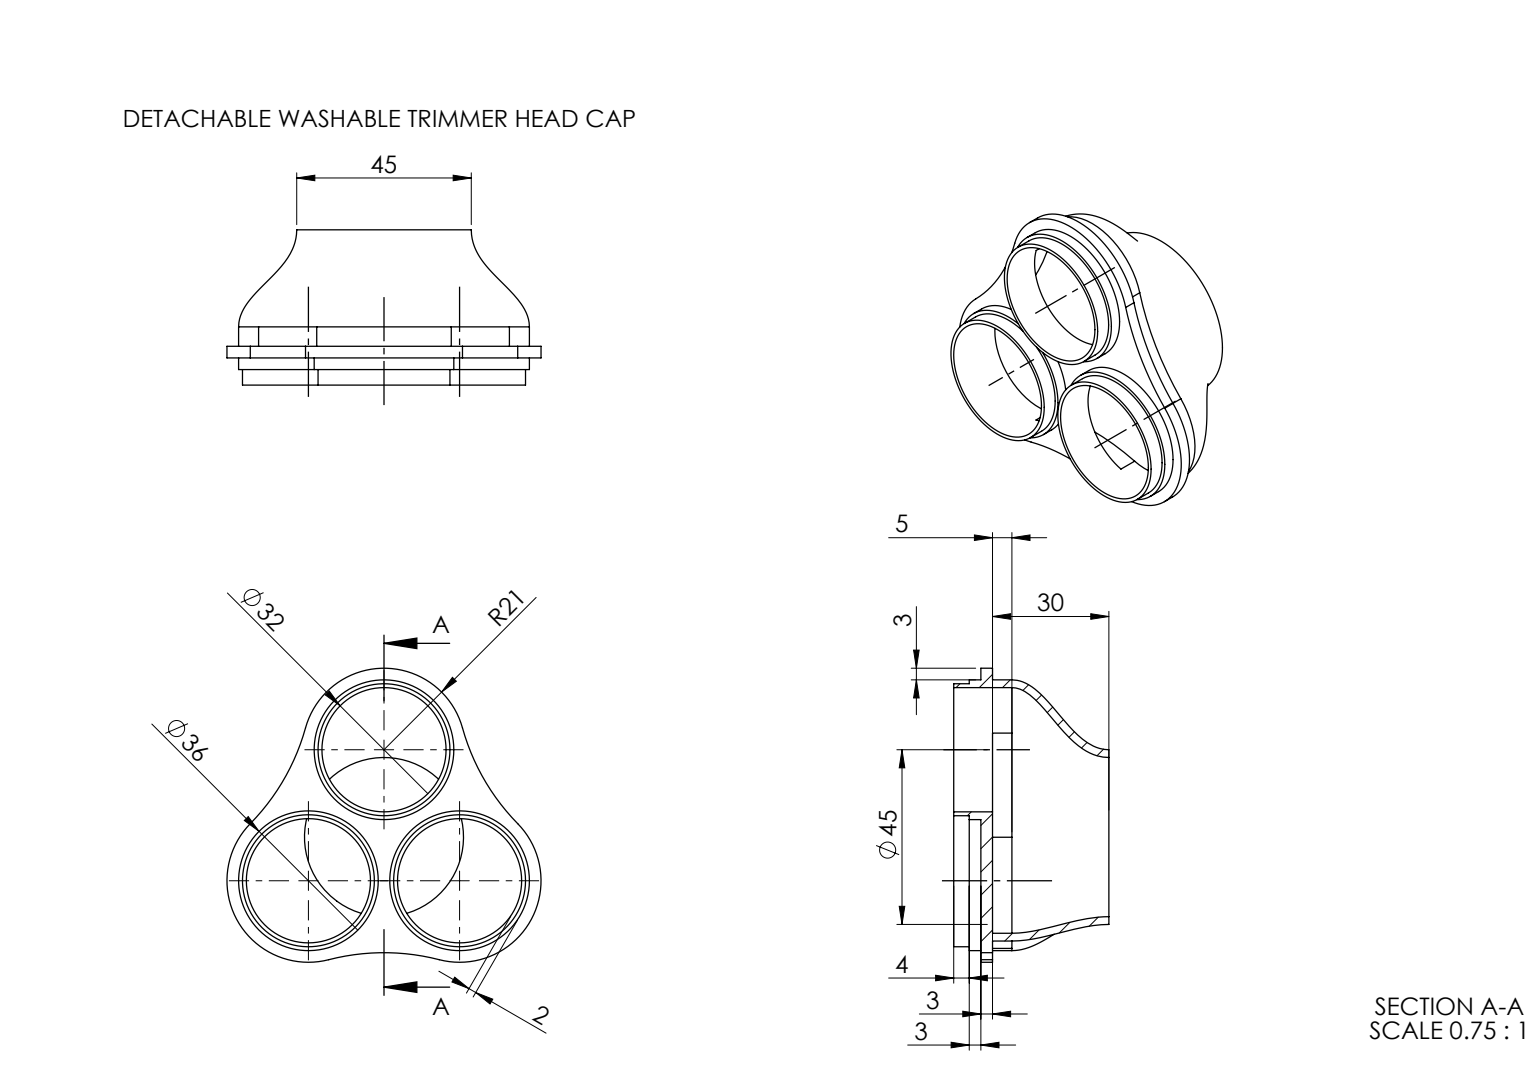
ISO-10303-21;
HEADER;
FILE_DESCRIPTION (('STEP AP214'),
    '1' );
FILE_NAME ('Detachable Washable Trimmer Head Cap.step',
    '2026-10-04T08:29:30',
    ( '' ),
    ( '' ),
    'SwSTEP 2.0',
    'SolidWorks 2026',
    '' );
FILE_SCHEMA (( 'AUTOMOTIVE_DESIGN' ));
ENDSEC;

DATA;
#3=CARTESIAN_POINT ( 'NONE',  ( -6.039637753342756987, 20.17599680590523192, -26.42895019650636712 ) ) ;
#8=CARTESIAN_POINT ( 'NONE',  ( 30.17671132303273041, 0.02011987000799879410, -8.767782600480947153 ) ) ;
#12=CARTESIAN_POINT ( 'NONE',  ( -29.54807517884461632, 0.1037351573273601335, -10.18168607448700591 ) ) ;
#15=CARTESIAN_POINT ( 'NONE',  ( 34.91117196809893386, -7.323106101878850360, -6.322142741489443551 ) ) ;
#28=CARTESIAN_POINT ( 'NONE',  ( 8.056271088701681293, 31.17318759581355536, -12.99397879114828491 ) ) ;
#30=CARTESIAN_POINT ( 'NONE',  ( 10.89305648074092225, -17.83927469781341912, -26.72577608409487127 ) ) ;
#31=PRESENTATION_STYLE_ASSIGNMENT (( #30520 ) ) ;
#35=CARTESIAN_POINT ( 'NONE',  ( -12.95130549116995766, 21.61585988689554227, -17.44156443216185437 ) ) ;
#38=CARTESIAN_POINT ( 'NONE',  ( 9.469227640886519026, -18.41450066817799680, -27.45857254820928262 ) ) ;
#43=CARTESIAN_POINT ( 'NONE',  ( -9.458574418659280170, 18.26235614098742843, -28.64307802517810941 ) ) ;
#44=CARTESIAN_POINT ( 'NONE',  ( -18.65979626009148973, -26.26407584738503331, -9.537061111741776287 ) ) ;
#47=CARTESIAN_POINT ( 'NONE',  ( -20.13126830103601250, -6.281551959463021362, -26.35909575268052052 ) ) ;
#49=CARTESIAN_POINT ( 'NONE',  ( -9.699069978481025700, -18.92072388944653127, -25.04460771491937265 ) ) ;
#52=CARTESIAN_POINT ( 'NONE',  ( 24.45230663209730793, 0.6563593020860170046, -18.47643289388101806 ) ) ;
#57=CARTESIAN_POINT ( 'NONE',  ( -29.40282053116814609, 0.01990383680175984021, -10.64941467521011909 ) ) ;
#59=CARTESIAN_POINT ( 'NONE',  ( 25.10121631073093340, -0.7699293454477268428, -18.29635744866308400 ) ) ;
#60=CARTESIAN_POINT ( 'NONE',  ( 8.060031444180253857, -18.86142350993543104, -30.00000000000000000 ) ) ;
#64=CARTESIAN_POINT ( 'NONE',  ( -20.37227374329378549, 4.299522256352382499, -26.46881427764473926 ) ) ;
#67=DIRECTION ( 'NONE',  ( 0.000000000000000000, 0.000000000000000000, 1.000000000000000000 ) ) ;
#76=CARTESIAN_POINT ( 'NONE',  ( -24.05674159856693706, 7.010567539539591664, -10.83448856670747062 ) ) ;
#79=CARTESIAN_POINT ( 'NONE',  ( 23.11526344011869938, -26.83253816688370819, -5.449048760028999183 ) ) ;
#82=CARTESIAN_POINT ( 'NONE',  ( 11.98848786654193255, 20.09305581486839287, -20.51223356901921235 ) ) ;
#84=CARTESIAN_POINT ( 'NONE',  ( -15.67656793722190045, 23.98187497218004083, -9.264872189972811256 ) ) ;
#89=CARTESIAN_POINT ( 'NONE',  ( 15.36333771843081841, 26.52970315206185958, -6.888084564221619743 ) ) ;
#93=CARTESIAN_POINT ( 'NONE',  ( -15.15181741199034882, 26.67644226825787612, -7.818864437366713993 ) ) ;
#95=CARTESIAN_POINT ( 'NONE',  ( -14.89520944345796494, -25.68604227067969603, -10.17218003502877899 ) ) ;
#99=CARTESIAN_POINT ( 'NONE',  ( -34.90754895111634681, -15.66705718490307753, -5.000000000000001776 ) ) ;
#100=CARTESIAN_POINT ( 'NONE',  ( -8.710418783113659913, -18.55732502341819767, -29.36346440193179674 ) ) ;
#102=CARTESIAN_POINT ( 'NONE',  ( 14.62730537770042893, 21.61436029863431685, -14.58249002882225476 ) ) ;
#104=CARTESIAN_POINT ( 'NONE',  ( 26.12479609234808819, 4.655573347657212757, -9.320158625236146577 ) ) ;
#109=CARTESIAN_POINT ( 'NONE',  ( -20.86432690731735562, 0.1532841330718156259, -26.77785373325384199 ) ) ;
#110=CARTESIAN_POINT ( 'NONE',  ( 30.11859346776113000, -0.3084563647293983579, -9.685108080598787694 ) ) ;
#115=EDGE_CURVE ( 'NONE', #32074, #26123, #27464, .T. ) ;
#116=CARTESIAN_POINT ( 'NONE',  ( 19.54664213359407654, -11.28525909758385914, -19.69475445967423610 ) ) ;
#122=CARTESIAN_POINT ( 'NONE',  ( 0.8345715822200899803, 20.57921025466891507, -28.44513613269969099 ) ) ;
#123=CARTESIAN_POINT ( 'NONE',  ( 0.000000000000000000, 22.50000000000000355, 6.000000000000000000 ) ) ;
#128=CARTESIAN_POINT ( 'NONE',  ( 14.95529536635265089, 27.95853494889172808, -6.397368112980813315 ) ) ;
#131=CARTESIAN_POINT ( 'NONE',  ( -14.93930595609077372, 14.05784520172980834, -29.41333909553293680 ) ) ;
#135=CARTESIAN_POINT ( 'NONE',  ( 15.46971733045241670, -26.73784336799789330, -5.000000000000000000 ) ) ;
#137=CARTESIAN_POINT ( 'NONE',  ( -22.79932625038946981, -26.94340799757786442, -5.449688136485410617 ) ) ;
#138=CARTESIAN_POINT ( 'NONE',  ( 11.00941871237314906, 17.34598387146357013, -28.70709525229845838 ) ) ;
#140=CARTESIAN_POINT ( 'NONE',  ( 11.46362546061642718, 18.45517822843765643, -23.85068629872059986 ) ) ;
#143=CARTESIAN_POINT ( 'NONE',  ( -9.432189322962019062, -18.20121415529274600, -30.00000000000000000 ) ) ;
#146=CARTESIAN_POINT ( 'NONE',  ( -28.29430579339429386, -20.85964472249671076, -11.08156269910200109 ) ) ;
#147=CARTESIAN_POINT ( 'NONE',  ( -0.3376553287050821917, -22.96943114444468392, -15.94602349255009521 ) ) ;
#148=CARTESIAN_POINT ( 'NONE',  ( 12.89389314760598104, 20.70404999538203228, -18.49322484050768267 ) ) ;
#149=CARTESIAN_POINT ( 'NONE',  ( 21.24142803452728501, 10.67320610155583971, -12.88465657304564083 ) ) ;
#152=CARTESIAN_POINT ( 'NONE',  ( -34.78690698786454760, -6.577732317142261032, -5.889322506088498166 ) ) ;
#158=CARTESIAN_POINT ( 'NONE',  ( -22.13218141308518483, 1.022649068119683147, -22.77793944450150931 ) ) ;
#160=CARTESIAN_POINT ( 'NONE',  ( 20.77567436899659725, -6.972680293972757681, -24.33364738463043153 ) ) ;
#173=CARTESIAN_POINT ( 'NONE',  ( -3.068187625016429276, 38.20266742920320269, -4.999999999999997335 ) ) ;
#176=B_SPLINE_CURVE_WITH_KNOTS ( 'NONE', 3,
 ( #11426, #39044, #29102, #33170, #14266, #32361 ),
 .UNSPECIFIED., .F., .F.,
 ( 4, 2, 4 ),
 ( 0.000000000000000000, 0.4999999999999998890, 1.000000000000000000 ),
 .UNSPECIFIED. ) ;
#179=CARTESIAN_POINT ( 'NONE',  ( 13.42433502267052958, 29.97960619171108476, -8.615981373113749342 ) ) ;
#181=CARTESIAN_POINT ( 'NONE',  ( -18.60936157838533589, 11.09020867803737609, -21.18208952860758387 ) ) ;
#183=CARTESIAN_POINT ( 'NONE',  ( 15.61814132907574759, -26.77569883083870650, -5.473565389543558091 ) ) ;
#185=CARTESIAN_POINT ( 'NONE',  ( 11.02015971874664224, 17.53795386546354962, -27.44368206178839387 ) ) ;
#187=CARTESIAN_POINT ( 'NONE',  ( -13.28992586503615847, -18.25382200079944539, -30.00000000000000711 ) ) ;
#191=CARTESIAN_POINT ( 'NONE',  ( -15.40573053741202791, 26.82015453055286969, -5.474029462766525356 ) ) ;
#192=CARTESIAN_POINT ( 'NONE',  ( -23.94859168923916215, -23.92721191009457726, -11.16030928171529979 ) ) ;
#193=CARTESIAN_POINT ( 'NONE',  ( 10.29923522730770280, -24.86304583090714004, -10.26489670867711546 ) ) ;
#194=CARTESIAN_POINT ( 'NONE',  ( 11.75310639014839431, 18.84718256836299588, -22.74606834583529036 ) ) ;
#195=CARTESIAN_POINT ( 'NONE',  ( 27.78181535516823786, -20.09500351851029265, -11.98703701457788462 ) ) ;
#199=CARTESIAN_POINT ( 'NONE',  ( -9.363295122093004963, 31.29718702830158605, -12.10286225948017602 ) ) ;
#200=CARTESIAN_POINT ( 'NONE',  ( 19.48557158514988075, -11.24999999999998224, 6.000000000000000000 ) ) ;
#204=CARTESIAN_POINT ( 'NONE',  ( 20.69210506600241217, 0.8672995041115374448, -27.44967104096003396 ) ) ;
#208=CARTESIAN_POINT ( 'NONE',  ( -20.60935208275203578, 0.8679898295200253466, -28.07838543686035493 ) ) ;
#213=CARTESIAN_POINT ( 'NONE',  ( 21.39727014468892108, -3.719077462541732437, -24.55904260327581667 ) ) ;
#214=AXIS2_PLACEMENT_3D ( 'NONE', #6009, #9672, #24306 ) ;
#227=CARTESIAN_POINT ( 'NONE',  ( -17.67638173720171935, 10.46809921990191228, -30.00000000000000355 ) ) ;
#231=CARTESIAN_POINT ( 'NONE',  ( 8.287352997579366942, 32.06355925594149880, -12.06759070029764480 ) ) ;
#233=CARTESIAN_POINT ( 'NONE',  ( 15.92400346575717762, -24.84455697418767528, -12.40895801513320507 ) ) ;
#238=CARTESIAN_POINT ( 'NONE',  ( -11.15269954372922356, 17.20160742699127709, -29.35198317640747234 ) ) ;
#241=CARTESIAN_POINT ( 'NONE',  ( 12.53737549699592435, -22.55629599919020123, -16.45275500735702323 ) ) ;
#243=ORIENTED_EDGE ( 'NONE', *, *, #35669, .F. ) ;
#245=CARTESIAN_POINT ( 'NONE',  ( -12.34506054626673333, 24.84528727421060523, -15.23039115023100543 ) ) ;
#246=CARTESIAN_POINT ( 'NONE',  ( -12.69359228199308376, -19.47210042018829768, -21.37302842195050800 ) ) ;
#250=CARTESIAN_POINT ( 'NONE',  ( -34.76827517156570480, -10.82915826946258697, -8.018781004229030174 ) ) ;
#251=CARTESIAN_POINT ( 'NONE',  ( -10.41464456071557265, -19.61101364636477484, -22.74980965849629300 ) ) ;
#254=CARTESIAN_POINT ( 'NONE',  ( 26.95107570311581213, 1.250167503761063559, -13.57310776412708897 ) ) ;
#258=CARTESIAN_POINT ( 'NONE',  ( -25.23791706649960176, 0.3308843942117839498, -17.43238208906259601 ) ) ;
#260=CARTESIAN_POINT ( 'NONE',  ( 20.49417979596975314, -0.6040919881699248206, -29.32140277093775893 ) ) ;
#261=VECTOR ( 'NONE', #29396, 1000.000000000000000 ) ;
#262=CARTESIAN_POINT ( 'NONE',  ( 17.66709127915118671, -10.40404091307350143, -30.00000000000003553 ) ) ;
#264=EDGE_CURVE ( 'NONE', #18645, #2968, #39539, .T. ) ;
#266=CARTESIAN_POINT ( 'NONE',  ( -26.84733007877831312, 4.410852123475765829, -6.430833405535962832 ) ) ;
#270=DIRECTION ( 'NONE',  ( 0.000000000000000000, 0.000000000000000000, 1.000000000000000000 ) ) ;
#276=CARTESIAN_POINT ( 'NONE',  ( -24.00624866131704493, 7.997915524243389918, -7.901842696615398509 ) ) ;
#279=CARTESIAN_POINT ( 'NONE',  ( 24.11167876243596098, -26.47814462355511367, -6.319563270833929103 ) ) ;
#281=CARTESIAN_POINT ( 'NONE',  ( 15.24364315846217899, 26.94041793836633403, -6.881005480939310637 ) ) ;
#284=CARTESIAN_POINT ( 'NONE',  ( -15.22236539853330761, 22.23089076743169912, -12.63797464781087676 ) ) ;
#286=ADVANCED_FACE ( 'NONE', ( #33861 ), #24901, .T. ) ;
#288=CARTESIAN_POINT ( 'NONE',  ( 14.31318613898417524, 24.41519415167184803, -12.55250302939356821 ) ) ;
#293=CARTESIAN_POINT ( 'NONE',  ( -10.86943063858312364, 17.38123995523577037, -29.34587341292847995 ) ) ;
#295=CARTESIAN_POINT ( 'NONE',  ( -15.32260095203325001, -26.31805409878302271, -8.292144503809835143 ) ) ;
#296=DIRECTION ( 'NONE',  ( 0.000000000000000000, 0.000000000000000000, 1.000000000000000000 ) ) ;
#298=CARTESIAN_POINT ( 'NONE',  ( -26.12381248617423068, -12.68530465514329997, -16.63598258512395489 ) ) ;
#299=CARTESIAN_POINT ( 'NONE',  ( -14.44360165411499786, -26.36321174074733165, -6.890051424692051896 ) ) ;
#301=CARTESIAN_POINT ( 'NONE',  ( 13.00986382136603048, 17.59953731938587040, -22.93413497736658258 ) ) ;
#303=CARTESIAN_POINT ( 'NONE',  ( 23.03828965240228754, 4.549470553047555654, -17.79268152331741604 ) ) ;
#309=CARTESIAN_POINT ( 'NONE',  ( -22.83159479309421869, 0.2693187709842888578, -21.57099463304014364 ) ) ;
#311=CARTESIAN_POINT ( 'NONE',  ( 30.96672106747950792, -0.2830252396438242557, -6.880588437363266863 ) ) ;
#315=CARTESIAN_POINT ( 'NONE',  ( -8.937590682902627037, -20.71651963383551731, -30.00000000000000000 ) ) ;
#319=ADVANCED_FACE ( 'NONE', ( #18023 ), #21649, .T. ) ;
#323=CARTESIAN_POINT ( 'NONE',  ( 1.450876755219358882, 20.54457168034460679, -28.44848653506505443 ) ) ;
#330=CIRCLE ( 'NONE', #13283, 56.99999999999991473 ) ;
#331=CARTESIAN_POINT ( 'NONE',  ( 12.99210526215103556, 23.76632269208105441, -15.34428991681221532 ) ) ;
#334=CARTESIAN_POINT ( 'NONE',  ( -16.63603619446163862, 16.45028161191871874, -16.85965045874825563 ) ) ;
#338=CARTESIAN_POINT ( 'NONE',  ( 9.776760815194750265, -18.56791727838074380, -26.22569070247839917 ) ) ;
#339=CARTESIAN_POINT ( 'NONE',  ( -21.82450030762573689, -25.89388939475013629, -9.434448713217458149 ) ) ;
#340=CARTESIAN_POINT ( 'NONE',  ( 15.37031333667682098, 26.67843416892376496, -6.417118344468947910 ) ) ;
#341=CARTESIAN_POINT ( 'NONE',  ( 14.28094865762740007, 24.49797395571547654, -12.54832579113776880 ) ) ;
#345=CARTESIAN_POINT ( 'NONE',  ( -12.21665226880467614, -22.02497210351782542, -17.44395964285717326 ) ) ;
#349=CARTESIAN_POINT ( 'NONE',  ( -16.60566614357999171, -12.18170714992408499, -28.45539122509774899 ) ) ;
#350=CARTESIAN_POINT ( 'NONE',  ( -0.2655791104724142260, -20.51720577492729092, -28.86250569332989002 ) ) ;
#351=CARTESIAN_POINT ( 'NONE',  ( 15.20852936758548779, 24.97080914613512448, -9.721994908021176940 ) ) ;
#353=CARTESIAN_POINT ( 'NONE',  ( 21.80268670686854549, 10.92046029907020888, -9.886650491983484557 ) ) ;
#355=EDGE_CURVE ( 'NONE', #35064, #7027, #28384, .T. ) ;
#357=CARTESIAN_POINT ( 'NONE',  ( -22.70368315883370158, -2.084503118412175393, -22.39977614792177008 ) ) ;
#362=CARTESIAN_POINT ( 'NONE',  ( -22.08665753359741402, 1.201892654560031248, -22.79865112719603459 ) ) ;
#363=CARTESIAN_POINT ( 'NONE',  ( 35.20762394452638944, -14.18514843260475011, -5.860995113772236920 ) ) ;
#378=CARTESIAN_POINT ( 'NONE',  ( -2.141861647269084123, 26.68515866033992623, -18.63047281487552098 ) ) ;
#384=CARTESIAN_POINT ( 'NONE',  ( 8.496730143421112658, 19.88634191853696720, -24.66085836945053700 ) ) ;
#386=CARTESIAN_POINT ( 'NONE',  ( -20.41576651639842765, 13.46337821832906201, -9.393711450338390279 ) ) ;
#388=CARTESIAN_POINT ( 'NONE',  ( 9.606819337878498288, -18.10969338424137831, -30.00000000000000000 ) ) ;
#390=CARTESIAN_POINT ( 'NONE',  ( 12.61335593425192769, 21.11317950107521568, -18.44339444917419613 ) ) ;
#391=CARTESIAN_POINT ( 'NONE',  ( 20.90924525106827758, -8.502318254486461058, -30.00000000000001421 ) ) ;
#394=CARTESIAN_POINT ( 'NONE',  ( -27.04961384508420608, -25.34883885810744886, -5.000000000000005329 ) ) ;
#395=CARTESIAN_POINT ( 'NONE',  ( 12.91994108110150208, -25.87706059209097731, -7.842292722746678990 ) ) ;
#396=CARTESIAN_POINT ( 'NONE',  ( 11.37508884758295657, 17.98716365035634368, -25.02329199648203328 ) ) ;
#397=CARTESIAN_POINT ( 'NONE',  ( 23.48339511270637914, -16.96163556805249684, -16.64869766514032889 ) ) ;
#401=CARTESIAN_POINT ( 'NONE',  ( -8.576574787394006805, 28.66784900714714723, -14.90473514947470157 ) ) ;
#403=CARTESIAN_POINT ( 'NONE',  ( -15.48853126089653642, -26.74269726827072446, -4.999999999999999112 ) ) ;
#409=CARTESIAN_POINT ( 'NONE',  ( 26.48649879351080472, 0.3041964394036508201, -15.45264338181639019 ) ) ;
#411=CIRCLE ( 'NONE', #35441, 18.00000000000000000 ) ;
#412=DIRECTION ( 'NONE',  ( 0.000000000000000000, 0.000000000000000000, 1.000000000000000000 ) ) ;
#414=CARTESIAN_POINT ( 'NONE',  ( -21.70419570142134802, 0.7541476106288704795, -23.85713393182268049 ) ) ;
#415=CARTESIAN_POINT ( 'NONE',  ( -20.01115660715129962, -26.54103525642217321, -8.595240659906115965 ) ) ;
#417=CARTESIAN_POINT ( 'NONE',  ( 20.40443380874665991, -3.526399787616441461, -27.86714167302821821 ) ) ;
#424=CARTESIAN_POINT ( 'NONE',  ( -19.48557158514988785, -11.24999999999987743, 10.00000000000000000 ) ) ;
#427=CARTESIAN_POINT ( 'NONE',  ( -20.50991189059329400, -0.1799011681176667099, -29.99999999999999645 ) ) ;
#430=CARTESIAN_POINT ( 'NONE',  ( 16.64822277588917032, 18.43813335370595752, -13.76538777124787494 ) ) ;
#431=CARTESIAN_POINT ( 'NONE',  ( 5.310336667938341471, 20.67330757391770035, -25.72323559496285128 ) ) ;
#434=CARTESIAN_POINT ( 'NONE',  ( 15.14142468963127897, -22.46172105866550339, -16.19430842129408177 ) ) ;
#439=CARTESIAN_POINT ( 'NONE',  ( -11.15269954372922356, 17.20160742699127709, -29.99999999999999645 ) ) ;
#441=CARTESIAN_POINT ( 'NONE',  ( 12.06224686842067406, -22.02997600949163015, -17.45733707754455821 ) ) ;
#446=CARTESIAN_POINT ( 'NONE',  ( -9.540218894060958021, 18.45143627731958347, -27.33005333713524720 ) ) ;
#447=CARTESIAN_POINT ( 'NONE',  ( -11.69803459526607625, -17.05285100544052312, -27.95431881375518657 ) ) ;
#451=CARTESIAN_POINT ( 'NONE',  ( -30.99736797329587290, -9.614891179495492324, -12.97104570887609931 ) ) ;
#452=CARTESIAN_POINT ( 'NONE',  ( -12.89014915853426224, -23.08559641726087719, -15.45851670612495887 ) ) ;
#455=CARTESIAN_POINT ( 'NONE',  ( 29.37184732250830521, 0.3033203897905300539, -10.18640792684451846 ) ) ;
#459=CARTESIAN_POINT ( 'NONE',  ( -30.88976141255646368, -0.06313707789208813925, -5.945739447080108597 ) ) ;
#461=CARTESIAN_POINT ( 'NONE',  ( 20.74532546937688338, -0.6322448352572834773, -27.35194312868669186 ) ) ;
#463=CARTESIAN_POINT ( 'NONE',  ( -5.359815401306925686, -19.79953048918116565, -30.00000000000000000 ) ) ;
#475=CARTESIAN_POINT ( 'NONE',  ( -19.72218505466810967, 7.980765556227030544, -23.29036116115986133 ) ) ;
#476=CARTESIAN_POINT ( 'NONE',  ( 22.61779009251464956, -26.31551665274535523, -8.089115201911514674 ) ) ;
#479=CARTESIAN_POINT ( 'NONE',  ( 10.88003517233900297, 17.37455259072008573, -30.00000000000000000 ) ) ;
#482=CARTESIAN_POINT ( 'NONE',  ( -14.02863424743453891, 20.80391705836231608, -16.56546359749882669 ) ) ;
#485=EDGE_CURVE ( 'NONE', #2217, #31250, #21009, .T. ) ;
#487=CARTESIAN_POINT ( 'NONE',  ( 11.04029860655090012, 17.32608448718281480, -28.70838011759155961 ) ) ;
#492=CARTESIAN_POINT ( 'NONE',  ( -11.33960866872714135, 18.56140262423198450, -23.83101412075703252 ) ) ;
#494=CARTESIAN_POINT ( 'NONE',  ( -14.24405758500416930, -24.64403535565174508, -12.53474328698910334 ) ) ;
#496=AXIS2_PLACEMENT_3D ( 'NONE', #14949, #12490, #18205 ) ;
#498=CARTESIAN_POINT ( 'NONE',  ( -33.71791919605428944, -15.10493296938091845, -8.852922798908716473 ) ) ;
#499=CARTESIAN_POINT ( 'NONE',  ( -9.692485564073882287, -19.34668444509729568, -23.91709408057471364 ) ) ;
#501=CARTESIAN_POINT ( 'NONE',  ( 13.86637344848912257, 19.30070053511032668, -18.64709189320727489 ) ) ;
#503=CARTESIAN_POINT ( 'NONE',  ( 26.00311425638208362, 4.651086067102406574, -9.804938788202040456 ) ) ;
#508=CARTESIAN_POINT ( 'NONE',  ( -22.38012257604306399, -0.01397392160533758761, -22.64776935873009123 ) ) ;
#509=CARTESIAN_POINT ( 'NONE',  ( 21.73684131651624796, 0.5819632018348794844, -23.83618332979514776 ) ) ;
#513=CARTESIAN_POINT ( 'NONE',  ( 12.33616729053617966, -27.99489201236593416, -13.58461195433497437 ) ) ;
#522=CARTESIAN_POINT ( 'NONE',  ( 2.722378455267432606, 20.72894175598409205, -26.99545394230949924 ) ) ;
#529=CARTESIAN_POINT ( 'NONE',  ( 14.90937338384046207, 27.40770937021949294, -7.795567658461852290 ) ) ;
#532=CARTESIAN_POINT ( 'NONE',  ( -17.91418368663225635, 16.64594202802076595, -12.82604463341725598 ) ) ;
#535=CARTESIAN_POINT ( 'NONE',  ( 11.53193418976769102, -20.97837345754841820, -19.49836150433041837 ) ) ;
#537=CARTESIAN_POINT ( 'NONE',  ( 15.17870064116790374, 26.26746426438345594, -8.297842380696128117 ) ) ;
#538=CARTESIAN_POINT ( 'NONE',  ( 14.73308801456976980, 25.40969082412797420, -10.65228738806455766 ) ) ;
#541=CARTESIAN_POINT ( 'NONE',  ( -9.556882383769263356, -18.37204861498985053, -27.45237673257718924 ) ) ;
#545=CARTESIAN_POINT ( 'NONE',  ( -26.76216378966945086, -19.72671915244844953, -12.90723624995964691 ) ) ;
#546=CARTESIAN_POINT ( 'NONE',  ( -4.347975343347115995, -23.51214084136499594, -13.86639182548506533 ) ) ;
#547=CARTESIAN_POINT ( 'NONE',  ( 15.43728935786161216, 25.42686383105192860, -8.304351359789887255 ) ) ;
#549=CARTESIAN_POINT ( 'NONE',  ( 21.75928845812402557, 9.796106908765645827, -12.87849264206665190 ) ) ;
#554=CARTESIAN_POINT ( 'NONE',  ( -32.67788646804365271, -3.365289809214419670, -8.615938099305980202 ) ) ;
#560=CARTESIAN_POINT ( 'NONE',  ( -29.88325193432147842, 0.8555504981620180027, -6.890743476730220252 ) ) ;
#561=CARTESIAN_POINT ( 'NONE',  ( 29.51672614961463736, -12.91057139293011602, -13.82673195968690649 ) ) ;
#572=CARTESIAN_POINT ( 'NONE',  ( -1.887696780556682219, 23.64799547898650189, -21.85798975256318855 ) ) ;
#573=CARTESIAN_POINT ( 'NONE',  ( -35.07906678349440455, -7.111640533861553592, -4.999999999999999112 ) ) ;
#580=CARTESIAN_POINT ( 'NONE',  ( 13.04798778810585347, 29.04188371427077087, -10.44273296311215304 ) ) ;
#582=CARTESIAN_POINT ( 'NONE',  ( -21.00653608580854481, 12.56855149973239172, -8.901572196327759201 ) ) ;
#583=DIRECTION ( 'NONE',  ( 0.000000000000000000, 0.000000000000000000, 1.000000000000000000 ) ) ;
#584=CARTESIAN_POINT ( 'NONE',  ( 10.31172964540912673, -19.13411530003786964, -23.84291266785244545 ) ) ;
#586=CARTESIAN_POINT ( 'NONE',  ( 15.26830110528803530, 26.60668572641256802, -7.355644065423295075 ) ) ;
#587=CARTESIAN_POINT ( 'NONE',  ( 37.62663912510992503, -8.659558992827971480, -14.26382729546509687 ) ) ;
#589=CARTESIAN_POINT ( 'NONE',  ( -25.85745970633643864, -25.73337701278340006, -6.737025561790457751 ) ) ;
#590=CARTESIAN_POINT ( 'NONE',  ( 8.302662708387121171, -24.93668839658822023, -8.846291834586214264 ) ) ;
#591=CARTESIAN_POINT ( 'NONE',  ( 15.08502492231579595, 25.75735284694121319, -9.240969017626685655 ) ) ;
#592=CARTESIAN_POINT ( 'NONE',  ( 18.23446778745489638, -12.32129691478622213, -24.23299356642612423 ) ) ;
#598=CARTESIAN_POINT ( 'NONE',  ( -8.428619364643951783, 35.98800784865809277, -6.299206775149388982 ) ) ;
#604=CARTESIAN_POINT ( 'NONE',  ( 28.92463652500844162, 0.06159917911152616721, -11.59545931083614079 ) ) ;
#610=CARTESIAN_POINT ( 'NONE',  ( -30.44556900789973852, 0.02942595176201418319, -7.828065574714944574 ) ) ;
#613=CARTESIAN_POINT ( 'NONE',  ( 31.36889017270395286, -5.558195913421866585, -12.17070191464305751 ) ) ;
#620=DIRECTION ( 'NONE',  ( 0.000000000000000000, 0.000000000000000000, 1.000000000000000000 ) ) ;
#623=CARTESIAN_POINT ( 'NONE',  ( -13.94509305167025204, 15.04106830562277253, -30.00000000000002132 ) ) ;
#626=CARTESIAN_POINT ( 'NONE',  ( 14.98739814520312130, 15.86604096426238364, -22.05070079658612059 ) ) ;
#627=CARTESIAN_POINT ( 'NONE',  ( 4.580011667354150440, 20.37550453228363878, -27.05156434026686441 ) ) ;
#630=CARTESIAN_POINT ( 'NONE',  ( 10.08241157172804670, -17.84938614438609505, -30.00000000000000000 ) ) ;
#635=CARTESIAN_POINT ( 'NONE',  ( -11.01210778500241361, 17.34425618060466689, -28.70720727591743682 ) ) ;
#637=CARTESIAN_POINT ( 'NONE',  ( 9.889788205164110835, -18.84469253480084205, -25.02328945438690866 ) ) ;
#639=EDGE_CURVE ( 'NONE', #11613, #16948, #14507, .T. ) ;
#640=ORIENTED_EDGE ( 'NONE', *, *, #14841, .F. ) ;
#642=CARTESIAN_POINT ( 'NONE',  ( -8.669908543505703946, 19.79285976321129681, -24.67981830963679357 ) ) ;
#645=CARTESIAN_POINT ( 'NONE',  ( -35.42614648568259383, -9.922089300916915988, -5.873467316378663483 ) ) ;
#646=CARTESIAN_POINT ( 'NONE',  ( -13.57768790248920254, -24.10155420078447719, -13.51926864417577079 ) ) ;
#648=VERTEX_POINT ( 'NONE', #32814 ) ;
#649=CARTESIAN_POINT ( 'NONE',  ( 24.49786104224794769, 0.5606131564536942502, -18.46619948923875754 ) ) ;
#653=CARTESIAN_POINT ( 'NONE',  ( -30.66481745429630834, -0.06869490606624445439, -7.356079483744078829 ) ) ;
#655=CARTESIAN_POINT ( 'NONE',  ( 31.43862993417205587, -1.740267522059486760, -9.139700976824004286 ) ) ;
#671=CARTESIAN_POINT ( 'NONE',  ( -22.79758257504442653, 9.829873109737514270, -7.912986613509453981 ) ) ;
#672=CARTESIAN_POINT ( 'NONE',  ( 24.21359695930263101, -26.57684320323437532, -5.000000000000000888 ) ) ;
#674=CARTESIAN_POINT ( 'NONE',  ( 14.20562871930490978, 24.69601559057154816, -12.53150451778845564 ) ) ;
#676=CARTESIAN_POINT ( 'NONE',  ( -13.79767463674636296, 21.20177806324913306, -16.53259672287590831 ) ) ;
#679=CARTESIAN_POINT ( 'NONE',  ( 11.91825936693510535, 19.35450465693568844, -21.62159660657380300 ) ) ;
#681=CARTESIAN_POINT ( 'NONE',  ( 18.51255757462615037, -10.21466864353301141, -26.25688464355175711 ) ) ;
#685=EDGE_LOOP ( 'NONE', ( #29987, #10385, #3731, #31281 ) ) ;
#686=CARTESIAN_POINT ( 'NONE',  ( -15.13223720903381420, 26.73911770198351334, -7.816828578819325024 ) ) ;
#689=CARTESIAN_POINT ( 'NONE',  ( -11.68873037371707646, -20.37810347578055215, -20.47508729926761006 ) ) ;
#693=CARTESIAN_POINT ( 'NONE',  ( -34.20107842149033672, -15.32937321432364541, -7.980157440187811702 ) ) ;
#694=CARTESIAN_POINT ( 'NONE',  ( -14.38923059561778750, -26.28103352123245884, -7.361378720437378398 ) ) ;
#696=CARTESIAN_POINT ( 'NONE',  ( 13.27244829273280580, 17.32419186230290364, -22.96854396723484371 ) ) ;
#698=CARTESIAN_POINT ( 'NONE',  ( 25.23600728880220601, 5.524756554899235006, -10.31010501861125483 ) ) ;
#703=CARTESIAN_POINT ( 'NONE',  ( -26.28050422335599734, -0.3854494769453477576, -16.35547130288665585 ) ) ;
#704=CARTESIAN_POINT ( 'NONE',  ( 29.81715026116830813, -0.1969218862350708976, -10.16156011328718733 ) ) ;
#709=CARTESIAN_POINT ( 'NONE',  ( 8.937590682902566641, -20.71651963383554218, -30.00000000000000000 ) ) ;
#718=CARTESIAN_POINT ( 'NONE',  ( 2.668841116913946987, 20.33496311051875693, -29.22043024060798544 ) ) ;
#723=CARTESIAN_POINT ( 'NONE',  ( 29.12711452743133123, -22.43287856296975136, -8.860495667039732126 ) ) ;
#726=LINE ( 'NONE', #37894, #21676 ) ;
#727=CARTESIAN_POINT ( 'NONE',  ( 10.90121339050992688, 18.34931554698703238, -24.95865895646690902 ) ) ;
#729=ORIENTED_EDGE ( 'NONE', *, *, #21810, .F. ) ;
#731=CARTESIAN_POINT ( 'NONE',  ( -17.41140981635742691, 20.80174530708337244, -5.476551464811988623 ) ) ;
#735=CARTESIAN_POINT ( 'NONE',  ( 10.20950366300454171, -19.16978685508543023, -23.85584966388176298 ) ) ;
#737=CARTESIAN_POINT ( 'NONE',  ( 10.99090272494190224, 17.30462611091308034, -29.34849402232231697 ) ) ;
#739=CARTESIAN_POINT ( 'NONE',  ( 15.22950456640031014, 26.41560797655204240, -7.827722518576876176 ) ) ;
#742=CARTESIAN_POINT ( 'NONE',  ( -9.628986672078191589, -18.46998302835118011, -26.83562301995240773 ) ) ;
#744=CARTESIAN_POINT ( 'NONE',  ( -31.54076586169206919, -21.75719626739306634, -5.857273151554024615 ) ) ;
#745=CARTESIAN_POINT ( 'NONE',  ( -4.676031460464607825, -24.51955512654058467, -9.374897136078594428 ) ) ;
#746=CARTESIAN_POINT ( 'NONE',  ( 11.42286652154374416, 17.26241004482871588, -27.47436460497770838 ) ) ;
#748=CARTESIAN_POINT ( 'NONE',  ( 18.42271044342168551, 9.437130544017666267, -26.61798538005301751 ) ) ;
#752=CARTESIAN_POINT ( 'NONE',  ( -33.32611593189657384, -4.382374629824890455, -8.137203135799296660 ) ) ;
#757=CARTESIAN_POINT ( 'NONE',  ( -24.93452846701059045, 1.910380023892134904, -16.57983970799203988 ) ) ;
#758=CARTESIAN_POINT ( 'NONE',  ( 33.76608682364540925, -14.77791854593863441, -8.856012205662965542 ) ) ;
#767=CARTESIAN_POINT ( 'NONE',  ( -0.5252917279287608876, 26.85053590416535485, -18.61061436390101420 ) ) ;
#774=CARTESIAN_POINT ( 'NONE',  ( 14.48331725184759478, 29.32085274443433676, -5.463096073128409280 ) ) ;
#777=CARTESIAN_POINT ( 'NONE',  ( -20.20127174136113979, 10.94879929003026575, -15.94514669860665812 ) ) ;
#780=CARTESIAN_POINT ( 'NONE',  ( 9.559327499438646569, -18.18575031750659576, -28.70543891380848933 ) ) ;
#782=CARTESIAN_POINT ( 'NONE',  ( 11.84840861761741770, 19.42896758927500755, -21.60864054467572970 ) ) ;
#783=CARTESIAN_POINT ( 'NONE',  ( -6.023418944065151770, 39.81932404830322270, -14.45070082761206365 ) ) ;
#784=FACE_OUTER_BOUND ( 'NONE', #14646, .T. ) ;
#785=CARTESIAN_POINT ( 'NONE',  ( -25.61532841618020129, -25.51455009192830659, -7.602007375326987670 ) ) ;
#786=CARTESIAN_POINT ( 'NONE',  ( 6.254033923143232698, -25.07628688208260215, -5.959964782852217979 ) ) ;
#787=CARTESIAN_POINT ( 'NONE',  ( 12.02371930289417712, 19.24250431711205422, -21.63974928700125844 ) ) ;
#788=CARTESIAN_POINT ( 'NONE',  ( 28.51898608182493433, -20.62815466463653635, -11.07930801063890591 ) ) ;
#793=CARTESIAN_POINT ( 'NONE',  ( -5.299830568715972134, 19.88204471691616249, -28.50950821733531271 ) ) ;
#796=CARTESIAN_POINT ( 'NONE',  ( 20.97107657471919140, 0.7936463442397385659, -26.22365389466587970 ) ) ;
#803=CARTESIAN_POINT ( 'NONE',  ( -29.22185649745145852, 0.2267782905184046460, -10.65771505781855844 ) ) ;
#804=CARTESIAN_POINT ( 'NONE',  ( -20.43668243666616391, -27.04690956338842867, -6.800953625924956114 ) ) ;
#806=CARTESIAN_POINT ( 'NONE',  ( 30.02603344819934961, -7.132601230694261218, -13.96448966489334254 ) ) ;
#818=( NAMED_UNIT ( * ) SI_UNIT ( $, .STERADIAN. ) SOLID_ANGLE_UNIT ( ) );
#819=CARTESIAN_POINT ( 'NONE',  ( 8.691530736372195420, 18.57012985596350774, -29.99999999999999645 ) ) ;
#823=CARTESIAN_POINT ( 'NONE',  ( 18.08305879496937507, 18.91083807987443777, -6.919464382693917059 ) ) ;
#825=CARTESIAN_POINT ( 'NONE',  ( 9.988892050414650114, 34.83439005035236846, -6.311689768854881422 ) ) ;
#828=CARTESIAN_POINT ( 'NONE',  ( 15.07574506840335182, -25.19415529391676145, -11.54849945562353675 ) ) ;
#832=CARTESIAN_POINT ( 'NONE',  ( -15.41919230091076187, 26.77186013819068577, -5.000000000000001776 ) ) ;
#835=CARTESIAN_POINT ( 'NONE',  ( 9.471631541704100599, -18.70210992107973880, -26.25392865717030233 ) ) ;
#838=B_SPLINE_CURVE_WITH_KNOTS ( 'NONE', 3,
 ( #28197, #3416, #573, #3223, #34107, #28798 ),
 .UNSPECIFIED., .F., .F.,
 ( 4, 2, 4 ),
 ( 0.7014326802556738460, 0.8507163401278369230, 1.000000000000000000 ),
 .UNSPECIFIED. ) ;
#840=CARTESIAN_POINT ( 'NONE',  ( -12.69759596664596479, 27.62578264501285474, -12.31174057995972859 ) ) ;
#841=CARTESIAN_POINT ( 'NONE',  ( -18.07439754813544042, -24.11643431014769234, -13.20271803398926735 ) ) ;
#845=CARTESIAN_POINT ( 'NONE',  ( -20.56951523689105343, -4.408057065260900131, -26.45586068485761189 ) ) ;
#848=CARTESIAN_POINT ( 'NONE',  ( 23.25665023848704749, 0.7203469195909389944, -20.56232886303743257 ) ) ;
#849=CARTESIAN_POINT ( 'NONE',  ( 11.47989394321261258, 18.44111858363577383, -23.85327844017400523 ) ) ;
#851=EDGE_CURVE ( 'NONE', #39696, #20959, #15707, .T. ) ;
#853=CARTESIAN_POINT ( 'NONE',  ( -29.63796514091300338, 0.003639834609975854327, -10.17682443054809838 ) ) ;
#856=CARTESIAN_POINT ( 'NONE',  ( 30.99264825080417651, -2.094996292503707558, -10.50450261084496262 ) ) ;
#860=VERTEX_POINT ( 'NONE', #18763 ) ;
#861=VECTOR ( 'NONE', #15724, 1000.000000000000000 ) ;
#874=CARTESIAN_POINT ( 'NONE',  ( -19.24333380943624050, 7.104126583969421205, -29.42120498672176154 ) ) ;
#875=CARTESIAN_POINT ( 'NONE',  ( 19.08127237847830315, -22.31786008396426624, -14.97965334449903629 ) ) ;
#878=CARTESIAN_POINT ( 'NONE',  ( 15.36998952511977912, 26.94570423236723755, -5.000000000000000888 ) ) ;
#881=CARTESIAN_POINT ( 'NONE',  ( -15.13444618763030469, 24.74347023186265204, -10.19675551309649997 ) ) ;
#884=CARTESIAN_POINT ( 'NONE',  ( 11.21793679047693892, 17.73202320564904966, -26.22846769416230472 ) ) ;
#886=CARTESIAN_POINT ( 'NONE',  ( 29.77249239352657284, -15.24433919496233258, -12.89210252282047797 ) ) ;
#887=DIRECTION ( 'NONE',  ( 1.000000000000000000, 0.000000000000000000, 0.000000000000000000 ) ) ;
#889=CARTESIAN_POINT ( 'NONE',  ( -15.23011890149219738, 27.15271631207409797, -6.409557253276911837 ) ) ;
#891=CARTESIAN_POINT ( 'NONE',  ( -9.617847002920147048, -18.10379274102027836, -29.34587326035947541 ) ) ;
#896=CARTESIAN_POINT ( 'NONE',  ( -35.24776836081323239, -13.33918002079275844, -6.287261223954184075 ) ) ;
#897=CARTESIAN_POINT ( 'NONE',  ( -8.710418783113659913, -18.55732502341819767, -29.99999999999999645 ) ) ;
#899=CARTESIAN_POINT ( 'NONE',  ( 15.07270250660410227, 20.73502926711271854, -14.63261333351891480 ) ) ;
#901=CARTESIAN_POINT ( 'NONE',  ( 26.80184643760344798, 3.774889638419365312, -9.304333590497897433 ) ) ;
#906=CARTESIAN_POINT ( 'NONE',  ( -20.62742209940435600, 0.5119082021479205435, -28.06054629692573243 ) ) ;
#907=CARTESIAN_POINT ( 'NONE',  ( 30.31228144303179661, -0.3231585995110547449, -9.216521076407452995 ) ) ;
#911=CARTESIAN_POINT ( 'NONE',  ( -20.55563217186184133, -29.52600041847739476, -4.999999999999992006 ) ) ;
#924=CARTESIAN_POINT ( 'NONE',  ( 16.57621650368579935, -13.52450271667361648, -25.63860445636134244 ) ) ;
#927=CARTESIAN_POINT ( 'NONE',  ( 10.41696638283783471, 17.65700839937217381, -30.00000000000000355 ) ) ;
#930=CARTESIAN_POINT ( 'NONE',  ( -16.52919907445785697, 19.39618867232801591, -12.74319168300435123 ) ) ;
#934=CARTESIAN_POINT ( 'NONE',  ( 12.62357604078584572, -22.55721479133982044, -16.44622715326968532 ) ) ;
#936=CARTESIAN_POINT ( 'NONE',  ( 14.93762947894291493, 25.79075299017892320, -9.709418743867059831 ) ) ;
#938=CARTESIAN_POINT ( 'NONE',  ( 15.41558956916364664, 26.78481017491955285, -5.474206059968303784 ) ) ;
#941=CARTESIAN_POINT ( 'NONE',  ( -11.26290815293687686, 18.07476739303793067, -25.00808982776462841 ) ) ;
#943=CARTESIAN_POINT ( 'NONE',  ( -14.82428456515288673, -25.82275059238470760, -9.709745829346953627 ) ) ;
#946=CARTESIAN_POINT ( 'NONE',  ( -19.10838325939929661, -14.03250534646638137, -21.87301868147889650 ) ) ;
#947=CARTESIAN_POINT ( 'NONE',  ( -7.052297394767913730, -25.17996142191265463, -5.478637597918203817 ) ) ;
#948=CARTESIAN_POINT ( 'NONE',  ( 15.36816765326552314, 25.28887897332994328, -8.776245744413783356 ) ) ;
#951=CARTESIAN_POINT ( 'NONE',  ( 20.10518103393213352, 8.324311984002667586, -21.14455001357749708 ) ) ;
#955=CARTESIAN_POINT ( 'NONE',  ( -33.52901403654990276, -3.501605748354566394, -5.457694923509727403 ) ) ;
#962=CARTESIAN_POINT ( 'NONE',  ( 34.52637764006742316, -16.38715731849997681, -6.278547096120509430 ) ) ;
#967=CARTESIAN_POINT ( 'NONE',  ( -20.20214925928707572, 14.56229221429976128, -5.000000000000000000 ) ) ;
#968=EDGE_CURVE ( 'NONE', #18645, #35629, #176, .T. ) ;
#973=CARTESIAN_POINT ( 'NONE',  ( -1.088922936409942421, 21.99923614848890097, -24.22294042631511246 ) ) ;
#980=CARTESIAN_POINT ( 'NONE',  ( 14.23920029309381974, 28.74314447264790928, -8.209473521281651642 ) ) ;
#983=ORIENTED_EDGE ( 'NONE', *, *, #3827, .F. ) ;
#984=CARTESIAN_POINT ( 'NONE',  ( -20.28121371388173344, 13.36466378765053165, -10.38440001512937627 ) ) ;
#987=CARTESIAN_POINT ( 'NONE',  ( 12.33240784613131602, -22.02210067590966958, -17.43238452351191370 ) ) ;
#989=CARTESIAN_POINT ( 'NONE',  ( 15.38567911973872171, 26.79894733746586510, -5.945569934900782449 ) ) ;
#990=CARTESIAN_POINT ( 'NONE',  ( 3.091399026088761826, 22.35909668862748489, -19.80438750953543803 ) ) ;
#993=CARTESIAN_POINT ( 'NONE',  ( -14.07208788724811477, -14.92005942896404669, -29.25347274896327932 ) ) ;
#994=CARTESIAN_POINT ( 'NONE',  ( 5.770784699189574596, -20.01892754147923270, -26.51040416381328058 ) ) ;
#995=CARTESIAN_POINT ( 'NONE',  ( 14.80735206003844340, 25.19352138484959980, -10.65771637371773117 ) ) ;
#997=CARTESIAN_POINT ( 'NONE',  ( 26.16185303258038886, -18.91739542788047501, -13.82176542154406818 ) ) ;
#998=CARTESIAN_POINT ( 'NONE',  ( -19.48557158514998022, -11.24999999999982414, -5.000000000000000000 ) ) ;
#1001=CARTESIAN_POINT ( 'NONE',  ( -6.470191821340285365, 24.31185124780299844, -19.83456026983462905 ) ) ;
#1005=CARTESIAN_POINT ( 'NONE',  ( 30.88264071866746008, -0.05584998072600699803, -5.946076430058510276 ) ) ;
#1009=CIRCLE ( 'NONE', #38616, 16.00000000000000000 ) ;
#1010=CARTESIAN_POINT ( 'NONE',  ( -26.44429670257990495, 0.3694839107847344151, -15.45773263958803945 ) ) ;
#1013=CARTESIAN_POINT ( 'NONE',  ( 33.18948647224070214, -7.908499970437028459, -10.28410421794941776 ) ) ;
#1023=ORIENTED_EDGE ( 'NONE', *, *, #968, .T. ) ;
#1024=CARTESIAN_POINT ( 'NONE',  ( -12.43436401264212954, 16.30149266761548787, -29.99999999999998579 ) ) ;
#1028=CARTESIAN_POINT ( 'NONE',  ( 16.44760013473877791, 18.13359219541155909, -14.76563877920854573 ) ) ;
#1029=CARTESIAN_POINT ( 'NONE',  ( 8.055990078716707359, 27.84801368489809192, -15.86024324141795105 ) ) ;
#1033=CARTESIAN_POINT ( 'NONE',  ( 10.44076220327837135, -18.61599742478032127, -24.95863081061211020 ) ) ;
#1038=CARTESIAN_POINT ( 'NONE',  ( -11.08838803815796048, 17.49214405190394217, -27.44899145124595918 ) ) ;
#1041=CARTESIAN_POINT ( 'NONE',  ( 14.97886844088684200, -26.54010076781190364, -6.417509905602858389 ) ) ;
#1046=CARTESIAN_POINT ( 'NONE',  ( -11.80691721808442018, 25.54223282131769324, -15.16446032101342034 ) ) ;
#1049=CARTESIAN_POINT ( 'NONE',  ( -20.04600691274970714, -4.289688609580842638, -29.25985845626247084 ) ) ;
#1052=CARTESIAN_POINT ( 'NONE',  ( 27.05411555961266856, 0.3588468966283088202, -14.48483347321499259 ) ) ;
#1057=CARTESIAN_POINT ( 'NONE',  ( -27.75511952204637112, 0.1671360698226562469, -13.51159890575608458 ) ) ;
#1060=CARTESIAN_POINT ( 'NONE',  ( 20.88781296840016566, -0.9792067608458780992, -26.69013418581465658 ) ) ;
#1061=CARTESIAN_POINT ( 'NONE',  ( 16.08977793723792615, 12.77418664379545277, -30.00000000000000000 ) ) ;
#1078=CARTESIAN_POINT ( 'NONE',  ( -22.43125282700144396, 9.709888685033304156, -10.37626387228879921 ) ) ;
#1080=CARTESIAN_POINT ( 'NONE',  ( 13.53326846751017776, -16.93861287502592461, -24.59972970754256139 ) ) ;
#1083=CARTESIAN_POINT ( 'NONE',  ( 13.39395081145689126, 23.01331212264283010, -15.42805658671999147 ) ) ;
#1085=CARTESIAN_POINT ( 'NONE',  ( -15.32210889896768080, 24.20449498080214568, -10.20718785661471273 ) ) ;
#1088=CARTESIAN_POINT ( 'NONE',  ( 15.43057444885795526, 26.63884252548692899, -5.946095807145699297 ) ) ;
#1089=VERTEX_POINT ( 'NONE', #32564 ) ;
#1090=CARTESIAN_POINT ( 'NONE',  ( 23.49686793660233164, -12.95939375123112924, -18.61325731074879641 ) ) ;
#1093=CARTESIAN_POINT ( 'NONE',  ( -11.97960752203429635, 20.10336228911335610, -20.51048379201368732 ) ) ;
#1095=CARTESIAN_POINT ( 'NONE',  ( -15.17654956054996340, -24.76925620166926834, -12.46321089911742419 ) ) ;
#1096=CARTESIAN_POINT ( 'NONE',  ( 0.000000000000000000, 22.50000000000000355, 0.000000000000000000 ) ) ;
#1098=CARTESIAN_POINT ( 'NONE',  ( -29.69559183934828184, -12.23830469681641198, -13.83596335006340361 ) ) ;
#1099=CARTESIAN_POINT ( 'NONE',  ( -13.96032889325439896, -26.00713114000728154, -8.307085670361487928 ) ) ;
#1100=DIRECTION ( 'NONE',  ( 1.000000000000000000, 0.000000000000000000, 0.000000000000000000 ) ) ;
#1101=CARTESIAN_POINT ( 'NONE',  ( 16.44978060298200262, 23.23702767493066901, -6.423945567198219742 ) ) ;
#1104=CARTESIAN_POINT ( 'NONE',  ( 20.14573521205405626, 4.508281606648074202, -27.63363721710107157 ) ) ;
#1109=ORIENTED_EDGE ( 'NONE', *, *, #6611, .F. ) ;
#1110=CARTESIAN_POINT ( 'NONE',  ( -22.28238350020720304, 0.4113152637605046458, -22.70236739277193294 ) ) ;
#1111=CARTESIAN_POINT ( 'NONE',  ( 20.62616697249115560, 0.5412120207698293273, -28.06201873610561748 ) ) ;
#1114=CARTESIAN_POINT ( 'NONE',  ( -16.77267017469753085, -29.13948811618693924, -13.79123840944732748 ) ) ;
#1126=CARTESIAN_POINT ( 'NONE',  ( 15.78360135397623232, -13.68898427767162218, -27.02986149001527849 ) ) ;
#1130=CARTESIAN_POINT ( 'NONE',  ( 11.52463565043312776, 19.76527168737703732, -21.54802219502610683 ) ) ;
#1132=CARTESIAN_POINT ( 'NONE',  ( 35.48557158514975640, -11.24999999999998046, 10.00000000000000000 ) ) ;
#1134=CARTESIAN_POINT ( 'NONE',  ( -17.46789482202738242, 19.19107468640789449, -9.821805770008548819 ) ) ;
#1136=CARTESIAN_POINT ( 'NONE',  ( 9.612089455291110696, -18.34516641601810960, -27.44844517416429852 ) ) ;
#1138=CARTESIAN_POINT ( 'NONE',  ( 15.42600414702388001, 26.74738280129588475, -5.474195457183328450 ) ) ;
#1140=CARTESIAN_POINT ( 'NONE',  ( 15.29107182738991355, 26.52751320015934056, -7.357832120508806639 ) ) ;
#1142=CARTESIAN_POINT ( 'NONE',  ( -11.85453240479826498, 19.42245932160622601, -21.60981001402871016 ) ) ;
#1144=CARTESIAN_POINT ( 'NONE',  ( -15.16455904780920605, -26.28013905145489559, -8.298198564278338907 ) ) ;
#1146=CARTESIAN_POINT ( 'NONE',  ( -31.16588773407646684, -20.14524002064360886, -8.845864470397883039 ) ) ;
#1147=CARTESIAN_POINT ( 'NONE',  ( -3.789163634868768504, -21.80995766230909183, -20.07097836427437443 ) ) ;
#1148=CARTESIAN_POINT ( 'NONE',  ( 11.49276420112067676, 17.21302641401697642, -27.47950092418111012 ) ) ;
#1150=CARTESIAN_POINT ( 'NONE',  ( 20.19436507835331440, 7.509872463613282534, -22.18560086142950993 ) ) ;
#1156=CARTESIAN_POINT ( 'NONE',  ( -32.75383215441653562, -2.524879539945301232, -6.828243879031231423 ) ) ;
#1163=CARTESIAN_POINT ( 'NONE',  ( 32.91113856765019108, -15.59652155672033125, -9.731851003150181256 ) ) ;
#1168=CARTESIAN_POINT ( 'NONE',  ( -15.49888991410544392, 26.48751662061146916, -5.000000000000000000 ) ) ;
#1173=CARTESIAN_POINT ( 'NONE',  ( -1.884094491940191407, 37.39490938450266100, -8.406240364095751261 ) ) ;
#1179=CARTESIAN_POINT ( 'NONE',  ( 10.37878353480403071, 20.06555603763842655, -22.52087948115185156 ) ) ;
#1184=CARTESIAN_POINT ( 'NONE',  ( -16.84542159628621860, 11.77608213748940358, -28.29354725645489665 ) ) ;
#1187=CARTESIAN_POINT ( 'NONE',  ( 15.31617560365994812, -26.41030191234985125, -7.825682279171108924 ) ) ;
#1189=CARTESIAN_POINT ( 'NONE',  ( 11.09563071542133450, 17.63336311864914663, -26.82764557179471510 ) ) ;
#1190=AXIS2_PLACEMENT_3D ( 'NONE', #27894, #67, #9614 ) ;
#1191=CARTESIAN_POINT ( 'NONE',  ( -19.69645987729884595, 11.37175641224115097, -29.99999999999998934 ) ) ;
#1194=CARTESIAN_POINT ( 'NONE',  ( -29.02322137993849438, -24.14915179229603837, -5.000000000000007994 ) ) ;
#1195=CARTESIAN_POINT ( 'NONE',  ( 5.647652911981364099, -19.78961436050011713, -28.81940954220644713 ) ) ;
#1196=CARTESIAN_POINT ( 'NONE',  ( 14.38725729136163345, 24.22873298939326148, -12.55976455580122675 ) ) ;
#1197=CARTESIAN_POINT ( 'NONE',  ( 17.17189741702122063, 11.35564286007100065, -27.73265135103572376 ) ) ;
#1202=CARTESIAN_POINT ( 'NONE',  ( -6.727062190665558106, 25.26119790492828088, -18.80720107704606647 ) ) ;
#1208=CARTESIAN_POINT ( 'NONE',  ( 29.82425386686576019, 0.01900928345093852792, -9.708684470575656533 ) ) ;
#1212=CARTESIAN_POINT ( 'NONE',  ( -29.89861541276895451, 0.1309397030943943996, -9.240080585033846106 ) ) ;
#1214=CARTESIAN_POINT ( 'NONE',  ( 30.12854829685219826, -8.081545850541484555, -13.92922311047432693 ) ) ;
#1231=CARTESIAN_POINT ( 'NONE',  ( 14.37745063133728962, 14.88579328056754392, -27.07234760961560838 ) ) ;
#1232=CARTESIAN_POINT ( 'NONE',  ( 10.87246471302026585, 34.12433032489231977, -6.319560934679609332 ) ) ;
#1236=CARTESIAN_POINT ( 'NONE',  ( 11.20115890257327429, -19.37169324739840803, -22.64800607319368098 ) ) ;
#1241=CARTESIAN_POINT ( 'NONE',  ( -12.14073867079856228, 19.91215881038760216, -20.54295507933877829 ) ) ;
#1244=CARTESIAN_POINT ( 'NONE',  ( 10.56033047147009363, -20.05577440089765773, -21.65083658459305838 ) ) ;
#1249=CARTESIAN_POINT ( 'NONE',  ( -12.16410700443224435, 28.43824891296100787, -12.25767132112050284 ) ) ;
#1252=CARTESIAN_POINT ( 'NONE',  ( -34.40806036129627898, -8.519187409710106351, -8.488083742945722321 ) ) ;
#1255=CARTESIAN_POINT ( 'NONE',  ( 30.57967879765778108, 0.1203670305863910467, -6.888307866855733153 ) ) ;
#1259=CARTESIAN_POINT ( 'NONE',  ( -20.81612948364115567, 0.8239250655022540837, -26.83009370459933152 ) ) ;
#1262=CARTESIAN_POINT ( 'NONE',  ( 33.89061681622978028, -4.196143601155450931, -5.455404339117079004 ) ) ;
#1273=CIRCLE ( 'NONE', #40184, 21.00000000000002842 ) ;
#1277=CARTESIAN_POINT ( 'NONE',  ( -23.34228009291333805, 8.898789006328664541, -8.395681560599031812 ) ) ;
#1278=CARTESIAN_POINT ( 'NONE',  ( 12.77972917816506104, -16.04224856310990432, -29.99999999999998224 ) ) ;
#1279=CARTESIAN_POINT ( 'NONE',  ( -13.29616015536805662, -18.15165799370312882, -30.00000000000000711 ) ) ;
#1281=CARTESIAN_POINT ( 'NONE',  ( 12.04731220300567962, 20.02368371182513229, -20.52401430719184816 ) ) ;
#1282=ORIENTED_EDGE ( 'NONE', *, *, #10347, .F. ) ;
#1283=CARTESIAN_POINT ( 'NONE',  ( -14.05791702678590482, 21.72486893603357316, -15.52982955538085363 ) ) ;
#1286=CARTESIAN_POINT ( 'NONE',  ( 12.44038979486233742, 20.42548900545279977, -19.50506954796185610 ) ) ;
#1288=CARTESIAN_POINT ( 'NONE',  ( 17.94885553750267349, -9.904091770223047320, -29.21232500953899347 ) ) ;
#1290=VERTEX_POINT ( 'NONE', #17733 ) ;
#1291=CARTESIAN_POINT ( 'NONE',  ( -13.60097212438034653, 23.76709706593192095, -14.43766431921598681 ) ) ;
#1293=CARTESIAN_POINT ( 'NONE',  ( -9.617847002920147048, -18.10379274102027836, -30.00000000000000000 ) ) ;
#1297=CARTESIAN_POINT ( 'NONE',  ( -19.30384401185921917, -8.002489564330206306, -26.99704546719047471 ) ) ;
#1298=CARTESIAN_POINT ( 'NONE',  ( -9.169462346764058580, -18.33493501355543742, -30.00000000000000000 ) ) ;
#1300=CARTESIAN_POINT ( 'NONE',  ( 14.17125917010577574, 17.46214553589771157, -20.85956934933411233 ) ) ;
#1302=CARTESIAN_POINT ( 'NONE',  ( 27.36042259163830082, 3.779474170926635512, -6.428186719520351922 ) ) ;
#1308=CARTESIAN_POINT ( 'NONE',  ( -30.66527662088913075, -0.2016734898252389718, -7.819459957311872600 ) ) ;
#1309=CARTESIAN_POINT ( 'NONE',  ( 31.16058696847114362, -0.7566004393934862016, -7.796922074218358922 ) ) ;
#1314=CARTESIAN_POINT ( 'NONE',  ( -11.10756861982300947, 19.59949212537556562, -29.99999999999999645 ) ) ;
#1319=CARTESIAN_POINT ( 'NONE',  ( 30.90412082983250741, -0.04211290444289944590, -5.000000000000000000 ) ) ;
#1326=CARTESIAN_POINT ( 'NONE',  ( 15.49469401537697877, -13.43643885346290645, -30.00000000000000000 ) ) ;
#1329=CARTESIAN_POINT ( 'NONE',  ( 13.75857034051007588, 24.56595210210346636, -13.45474119376723188 ) ) ;
#1332=CARTESIAN_POINT ( 'NONE',  ( -14.93930595609077372, 14.05784520172980834, -30.00000000000002132 ) ) ;
#1334=CARTESIAN_POINT ( 'NONE',  ( 9.515264969114221927, -18.30106724108619787, -28.08047306799037202 ) ) ;
#1336=CARTESIAN_POINT ( 'NONE',  ( 15.02664410326935851, 25.94178776440897494, -9.238651380280199277 ) ) ;
#1338=CARTESIAN_POINT ( 'NONE',  ( 15.09864989872857244, 26.14700263954316029, -8.767557201553991320 ) ) ;
#1340=CARTESIAN_POINT ( 'NONE',  ( -14.70308516012370248, 25.50042804345432756, -10.64636925701135617 ) ) ;
#1342=CARTESIAN_POINT ( 'NONE',  ( -14.31400716352764668, -25.06285765673995769, -11.60025332831071054 ) ) ;
#1345=CARTESIAN_POINT ( 'NONE',  ( -31.84658246857330965, -19.23773494732160572, -8.842712113036586885 ) ) ;
#1346=CARTESIAN_POINT ( 'NONE',  ( -2.475031807174856713, -24.15412266750587023, -10.88196088067523881 ) ) ;
#1347=CARTESIAN_POINT ( 'NONE',  ( 11.56847964180033728, 16.97430105090107233, -28.72963091288654169 ) ) ;
#1349=CARTESIAN_POINT ( 'NONE',  ( 22.28759716408703895, 8.923642387558418321, -12.86559102559659351 ) ) ;
#1352=CARTESIAN_POINT ( 'NONE',  ( -10.15119711060580343, -25.59814205317665881, -4.999999999999997335 ) ) ;
#1355=CARTESIAN_POINT ( 'NONE',  ( -20.87597923362057983, -1.832164627360789666, -26.62503287721647993 ) ) ;
#1362=CARTESIAN_POINT ( 'NONE',  ( 1.485571585149874529, -11.25000000000009415, 3.000000000000000000 ) ) ;
#1363=CARTESIAN_POINT ( 'NONE',  ( 21.69165369200475624, -9.527500816022886454, -21.87585738750458475 ) ) ;
#1371=CARTESIAN_POINT ( 'NONE',  ( -0.7505169017605982651, 38.27747495725317606, -6.696244658323041499 ) ) ;
#1380=CARTESIAN_POINT ( 'NONE',  ( 11.86081488739372958, 24.33169448125006795, -16.19729836796659939 ) ) ;
#1383=CARTESIAN_POINT ( 'NONE',  ( -17.39430208471609163, 11.24351447107411772, -26.62001118384078779 ) ) ;
#1386=CARTESIAN_POINT ( 'NONE',  ( 9.770751854196934261, -18.40326536504920796, -26.82356556862325547 ) ) ;
#1388=CARTESIAN_POINT ( 'NONE',  ( 15.32336983265158281, 26.66990810724929872, -6.886851398718627948 ) ) ;
#1389=CARTESIAN_POINT ( 'NONE',  ( 4.336808689942017736E-15, 40.84107189184581443, -5.000000000000008882 ) ) ;
#1391=CARTESIAN_POINT ( 'NONE',  ( -16.43502440684527599, -14.51438213871383454, -24.33132401675261747 ) ) ;
#1392=CARTESIAN_POINT ( 'NONE',  ( 5.635282026549600864, -19.76630616200782242, -29.40695735224786844 ) ) ;
#1393=CARTESIAN_POINT ( 'NONE',  ( 15.52561063650128759, 26.30458316266247110, -5.946179686823199972 ) ) ;
#1394=CARTESIAN_POINT ( 'NONE',  ( 18.66890321014120246, 12.51461972714008652, -18.00895683570465522 ) ) ;
#1398=CARTESIAN_POINT ( 'NONE',  ( -8.453943144716905778, 36.13191751627968529, -5.000000000000000888 ) ) ;
#1401=CARTESIAN_POINT ( 'NONE',  ( -11.40809387606930336, -20.99419242044788803, -19.51149134545002184 ) ) ;
#1410=CARTESIAN_POINT ( 'NONE',  ( -30.38029091318623642, 0.09813233376897281812, -7.828559720627486840 ) ) ;
#1412=CARTESIAN_POINT ( 'NONE',  ( 34.90301088146017605, -9.422820822732527191, -7.602032696592240235 ) ) ;
#1428=CARTESIAN_POINT ( 'NONE',  ( 17.57999905932629048, 16.66487347840518041, -13.82914334805849421 ) ) ;
#1429=CARTESIAN_POINT ( 'NONE',  ( 10.76909278579559981, 33.72652210473967926, -7.628981730212053947 ) ) ;
#1433=CARTESIAN_POINT ( 'NONE',  ( 16.42748648437301640, -26.82053992255703889, -6.866534988705063292 ) ) ;
#1434=FACE_BOUND ( 'NONE', #30961, .T. ) ;
#1437=CARTESIAN_POINT ( 'NONE',  ( -10.98473797697927701, 17.30853926952405075, -29.34836101394438401 ) ) ;
#1439=CARTESIAN_POINT ( 'NONE',  ( 14.86825508979877064, -26.56089389575996407, -5.946233135902982525 ) ) ;
#1443=CARTESIAN_POINT ( 'NONE',  ( -13.13940279579264825, 30.96237069512062590, -7.695636096163062767 ) ) ;
#1448=CARTESIAN_POINT ( 'NONE',  ( -33.37315695507471958, -7.245599113437738659, -9.850161829985118800 ) ) ;
#1450=VERTEX_POINT ( 'NONE', #28600 ) ;
#1451=CARTESIAN_POINT ( 'NONE',  ( 27.60362641570377207, 0.3697951749082440953, -13.52364084678252887 ) ) ;
#1457=CARTESIAN_POINT ( 'NONE',  ( -28.35170116396216144, 0.1243089573432585720, -12.54891019634939298 ) ) ;
#1460=CARTESIAN_POINT ( 'NONE',  ( 23.33064708864463555, -1.963756010919469830, -21.28980525675968849 ) ) ;
#1462=CARTESIAN_POINT ( 'NONE',  ( 12.92776996871492479, 15.91343586356105533, -30.00000000000001421 ) ) ;
#1475=CARTESIAN_POINT ( 'NONE',  ( 4.832435196289363688, 29.43795123185613249, -15.73446877130611377 ) ) ;
#1479=CARTESIAN_POINT ( 'NONE',  ( -20.87744296876565286, 11.29336303379088235, -12.88788702006255349 ) ) ;
#1480=CARTESIAN_POINT ( 'NONE',  ( 18.22149445818437385, -22.61346887214493862, -15.02646902325029643 ) ) ;
#1482=CARTESIAN_POINT ( 'NONE',  ( -33.63536641588170539, -18.98279099655679758, -4.999999999999999112 ) ) ;
#1483=CARTESIAN_POINT ( 'NONE',  ( 15.38842093998857230, 26.88136989284191003, -5.000000000000000000 ) ) ;
#1485=CARTESIAN_POINT ( 'NONE',  ( -12.44742484898385904, 17.58201857736815299, -23.99274416867952553 ) ) ;
#1488=CARTESIAN_POINT ( 'NONE',  ( 11.16523723692197478, 17.58493466368048530, -26.83415995730371506 ) ) ;
#1490=CARTESIAN_POINT ( 'NONE',  ( 32.80703094730063185, -16.80140863343335766, -9.283588785457341785 ) ) ;
#1492=CARTESIAN_POINT ( 'NONE',  ( -12.24516985351738718, 20.68376759742653093, -19.46578503039011210 ) ) ;
#1494=CARTESIAN_POINT ( 'NONE',  ( -16.22334360803714404, -26.92298677526160233, -5.000000000000000888 ) ) ;
#1498=CARTESIAN_POINT ( 'NONE',  ( -26.43177126521426956, -11.85372628369261250, -16.64861771188786221 ) ) ;
#1499=CARTESIAN_POINT ( 'NONE',  ( -11.10430509875484084, -21.03298634457605232, -19.54320612427354931 ) ) ;
#1501=CARTESIAN_POINT ( 'NONE',  ( 17.03376377104290640, 20.70341664989160435, -8.831506936632600002 ) ) ;
#1503=CARTESIAN_POINT ( 'NONE',  ( 20.24413271415620841, 3.804288779818567612, -28.19920182012378973 ) ) ;
#1508=CARTESIAN_POINT ( 'NONE',  ( -29.12724189388964291, -0.1775561609936863183, -11.57335334406140426 ) ) ;
#1509=CARTESIAN_POINT ( 'NONE',  ( 30.44880780573000933, -0.6958124801958616157, -9.659808045383314834 ) ) ;
#1513=CARTESIAN_POINT ( 'NONE',  ( -28.42036332966587509, 2.623993810986071651, -5.474604813331526820 ) ) ;
#1514=CARTESIAN_POINT ( 'NONE',  ( 11.31392148919589680, 36.91540483778863546, -14.26382729546508088 ) ) ;
#1528=CARTESIAN_POINT ( 'NONE',  ( 27.06419666510200273, -24.97747390337942619, -7.153125932697236067 ) ) ;
#1532=CARTESIAN_POINT ( 'NONE',  ( 10.61561400868404093, 17.69690613582448080, -28.05214642998929619 ) ) ;
#1536=CARTESIAN_POINT ( 'NONE',  ( -16.97888402983207001, 18.46751920095590194, -12.77518134462292920 ) ) ;
#1538=CARTESIAN_POINT ( 'NONE',  ( 11.46880063084097578, -20.98643766582429393, -19.50507162110192638 ) ) ;
#1541=CARTESIAN_POINT ( 'NONE',  ( 15.02941416159078791, 25.93298973513185146, -9.238761048664686726 ) ) ;
#1543=CARTESIAN_POINT ( 'NONE',  ( 15.39919595897972826, 26.75075905497473627, -5.946079338151666782 ) ) ;
#1545=CARTESIAN_POINT ( 'NONE',  ( -13.99993087335245256, 24.00799898784267583, -13.50638822794025629 ) ) ;
#1547=CARTESIAN_POINT ( 'NONE',  ( -9.487969581998370927, -18.17220041443854583, -29.34855226819949081 ) ) ;
#1549=CARTESIAN_POINT ( 'NONE',  ( -19.95015686455310799, -12.87654000693452083, -21.84574686077818484 ) ) ;
#1551=CARTESIAN_POINT ( 'NONE',  ( -6.273692019901858430, -19.88452076598854745, -26.48636925569244127 ) ) ;
#1552=CARTESIAN_POINT ( 'NONE',  ( 11.77204130854469000, 17.01331900727792856, -27.49973913441361972 ) ) ;
#1554=CARTESIAN_POINT ( 'NONE',  ( 21.35817030649165105, 7.746940167569142943, -17.95549415092490975 ) ) ;
#1559=CARTESIAN_POINT ( 'NONE',  ( -25.18061870383569811, -0.9857286467851488210, -18.27162094256875591 ) ) ;
#1567=CARTESIAN_POINT ( 'NONE',  ( 18.88476749628562246, -8.988548275649279162, -26.97612708522287761 ) ) ;
#1575=CARTESIAN_POINT ( 'NONE',  ( -0.4624081962452046834, 23.76772061069408792, -21.83626832166117282 ) ) ;
#1576=DIRECTION ( 'NONE',  ( 1.000000000000000000, 0.000000000000000000, 0.000000000000000000 ) ) ;
#1584=CARTESIAN_POINT ( 'NONE',  ( 12.73726530754508701, 25.36863251623071491, -14.28276732290829898 ) ) ;
#1587=CARTESIAN_POINT ( 'NONE',  ( -20.06818878704502751, 14.54951294394186689, -7.913531450302784265 ) ) ;
#1591=CARTESIAN_POINT ( 'NONE',  ( 15.44320054554677846, -26.65646054649087660, -6.416728767745834894 ) ) ;
#1594=CARTESIAN_POINT ( 'NONE',  ( 13.75002412159893694, 23.44003394427787512, -14.47165457257529653 ) ) ;
#1595=CARTESIAN_POINT ( 'NONE',  ( -27.08779848459120743, 7.221796966026712283, -13.42901749168596481 ) ) ;
#1598=CARTESIAN_POINT ( 'NONE',  ( -15.21888313924808855, -14.28223729339822157, -27.05990642766832721 ) ) ;
#1599=CARTESIAN_POINT ( 'NONE',  ( 3.973911541953894400, -24.68614102020093881, -7.909360114664225172 ) ) ;
#1600=CARTESIAN_POINT ( 'NONE',  ( 12.57937835649980052, 20.24290211102249160, -19.52900479813045465 ) ) ;
#1601=CARTESIAN_POINT ( 'NONE',  ( 18.03593615372940917, 12.02637506715544724, -21.17004988786488084 ) ) ;
#1604=CARTESIAN_POINT ( 'NONE',  ( -4.144713709954233494, 20.47503900711864588, -27.03594048031756358 ) ) ;
#1609=ADVANCED_FACE ( 'NONE', ( #26963 ), #20476, .T. ) ;
#1613=CARTESIAN_POINT ( 'NONE',  ( -20.96534858468971407, 0.8490077867318273075, -26.22846716918471799 ) ) ;
#1615=CARTESIAN_POINT ( 'NONE',  ( 21.10173320963569310, -5.688633216797759573, -24.40913811835638114 ) ) ;
#1632=CARTESIAN_POINT ( 'NONE',  ( 15.29022352314591870, 13.67480013622697044, -29.41691902321640129 ) ) ;
#1633=CARTESIAN_POINT ( 'NONE',  ( 6.698736661597710196, 23.19293624795248121, -20.94025436800699680 ) ) ;
#1637=CARTESIAN_POINT ( 'NONE',  ( 16.00895768845574096, -26.86996021029318626, -5.000000000000000888 ) ) ;
#1642=CARTESIAN_POINT ( 'NONE',  ( -10.97587534684186927, 17.31416389292776614, -29.99999999999999289 ) ) ;
#1644=CARTESIAN_POINT ( 'NONE',  ( 14.88849274807932765, -26.59100623965352739, -5.474081762690492958 ) ) ;
#1648=CARTESIAN_POINT ( 'NONE',  ( -9.086544612771062290, 22.80237608603660959, -20.06330228535229310 ) ) ;
#1653=CARTESIAN_POINT ( 'NONE',  ( -26.18072848307312483, -5.656370036759490461, -17.86034429590615602 ) ) ;
#1657=CARTESIAN_POINT ( 'NONE',  ( 29.30560488958938237, 0.1302769183488891036, -10.65503282581417643 ) ) ;
#1662=CARTESIAN_POINT ( 'NONE',  ( -20.61119921438281821, 0.8364689388151540506, -28.07681394956128784 ) ) ;
#1666=CARTESIAN_POINT ( 'NONE',  ( 33.23936858253276228, -3.197057837266320313, -6.364182858326340231 ) ) ;
#1668=ORIENTED_EDGE ( 'NONE', *, *, #24369, .T. ) ;
#1679=CARTESIAN_POINT ( 'NONE',  ( 6.086663952044554016, 37.28955090192621213, -5.862872072945212842 ) ) ;
#1684=CARTESIAN_POINT ( 'NONE',  ( 18.27717518933982177, -25.33298382040178609, -11.36505120164252247 ) ) ;
#1689=CARTESIAN_POINT ( 'NONE',  ( 15.37200336808687950, 26.84711675505732131, -5.945063123470434974 ) ) ;
#1691=CARTESIAN_POINT ( 'NONE',  ( -11.29390458575034373, 17.10922195600983997, -29.99999999999999645 ) ) ;
#1695=CARTESIAN_POINT ( 'NONE',  ( 14.06582128944119070, 23.85096756361283354, -13.51722347730761697 ) ) ;
#1697=CARTESIAN_POINT ( 'NONE',  ( 28.82830481445685677, -17.06062050408562669, -12.88833261073628478 ) ) ;
#1699=CARTESIAN_POINT ( 'NONE',  ( -11.51955146840040456, 19.07033770647171877, -22.70621963616805061 ) ) ;
#1701=CARTESIAN_POINT ( 'NONE',  ( -10.72424208444558147, -18.49280626366203961, -24.92494540156139138 ) ) ;
#1704=CARTESIAN_POINT ( 'NONE',  ( -35.38382356931356298, -13.39769055746643112, -5.000000000000005329 ) ) ;
#1705=CARTESIAN_POINT ( 'NONE',  ( -10.14892113523442951, -19.68697069789514842, -22.78142312659023005 ) ) ;
#1707=CARTESIAN_POINT ( 'NONE',  ( 14.83185561455345791, 18.64992817094902122, -17.71824246541178738 ) ) ;
#1709=CARTESIAN_POINT ( 'NONE',  ( 21.00252652683522570, 3.785488330333473872, -24.15676876065577972 ) ) ;
#1716=CARTESIAN_POINT ( 'NONE',  ( -31.05219368549945003, -0.2312423517573455878, -5.943383185067190766 ) ) ;
#1718=CARTESIAN_POINT ( 'NONE',  ( 20.99902718400924329, 0.4997691857017135253, -26.19762432007799546 ) ) ;
#1723=CARTESIAN_POINT ( 'NONE',  ( -28.19395260050296770, 0.9484113493885590884, -11.62985173043690246 ) ) ;
#1724=CARTESIAN_POINT ( 'NONE',  ( -15.29245034862078256, 32.56469986091995850, -13.99876745781543441 ) ) ;
#1733=CARTESIAN_POINT ( 'NONE',  ( -21.26609381498803231, 5.820186529508268869, -21.02685273093531748 ) ) ;
#1736=CARTESIAN_POINT ( 'NONE',  ( 15.94941446643157512, -13.01052313326162491, -28.46982544010355198 ) ) ;
#1739=CARTESIAN_POINT ( 'NONE',  ( 11.83975480655455392, 20.26533495932481799, -20.48298615583043869 ) ) ;
#1742=CARTESIAN_POINT ( 'NONE',  ( -13.44539276212325341, 15.67996942108016967, -27.60600344130554262 ) ) ;
#1745=CARTESIAN_POINT ( 'NONE',  ( 14.90790700096789045, -25.97435605518935731, -9.239200025327670929 ) ) ;
#1747=CARTESIAN_POINT ( 'NONE',  ( 14.54031622545319813, 24.94891456728954537, -11.59962563409148650 ) ) ;
#1751=CARTESIAN_POINT ( 'NONE',  ( -14.49572269434710137, 25.07545077057084981, -11.59117096907117173 ) ) ;
#1753=CARTESIAN_POINT ( 'NONE',  ( -9.942277346636780422, -18.82355019788865746, -25.01733364873610199 ) ) ;
#1755=CARTESIAN_POINT ( 'NONE',  ( -26.28505616161186964, -16.99079149096458607, -14.73553854996467827 ) ) ;
#1756=CARTESIAN_POINT ( 'NONE',  ( -7.384991535497307247, -21.86536290796619397, -18.83959722162714812 ) ) ;
#1757=CARTESIAN_POINT ( 'NONE',  ( 15.64374290521436706, 24.45313499581702743, -8.785383034557462167 ) ) ;
#1759=CARTESIAN_POINT ( 'NONE',  ( 19.22578323039330428, 8.090122520240742077, -25.48513230106247107 ) ) ;
#1763=ORIENTED_EDGE ( 'NONE', *, *, #15705, .F. ) ;
#1764=CARTESIAN_POINT ( 'NONE',  ( -32.47918921017399896, -2.488034356860049368, -7.737705398647766408 ) ) ;
#1770=CARTESIAN_POINT ( 'NONE',  ( 25.18859414265934049, -11.95731909848912089, -17.61046221350143526 ) ) ;
#1780=CARTESIAN_POINT ( 'NONE',  ( 0.4095834978660508607, 38.24721862872263500, -6.696645721537974438 ) ) ;
#1786=CARTESIAN_POINT ( 'NONE',  ( 12.58176986377051954, 23.30251563080998878, -16.31430736139012083 ) ) ;
#1789=CARTESIAN_POINT ( 'NONE',  ( -17.05764571048761624, 11.96101966799990812, -25.49672756633158599 ) ) ;
#1792=CARTESIAN_POINT ( 'NONE',  ( 11.92998010801955289, -21.48326688710186616, -18.44930693513468967 ) ) ;
#1793=FACE_OUTER_BOUND ( 'NONE', #18159, .T. ) ;
#1794=CARTESIAN_POINT ( 'NONE',  ( 12.63339664555651609, 21.08327326440629079, -18.44782762665456843 ) ) ;
#1799=CARTESIAN_POINT ( 'NONE',  ( -15.54722730493476135, -13.72744853134184062, -27.75932108635244333 ) ) ;
#1800=CARTESIAN_POINT ( 'NONE',  ( 1.815840917229304186, -24.74890125078012915, -5.967798877961429049 ) ) ;
#1801=CARTESIAN_POINT ( 'NONE',  ( 15.30416110356804182, 25.85440126521964999, -8.300953238907675669 ) ) ;
#1802=CARTESIAN_POINT ( 'NONE',  ( 17.40089361578718297, 12.57718761390114715, -22.22887343362824097 ) ) ;
#1806=CARTESIAN_POINT ( 'NONE',  ( -4.503003596829367794, 22.23197666336542255, -23.10559598243666812 ) ) ;
#1807=AXIS2_PLACEMENT_3D ( 'NONE', #17374, #39086, #17572 ) ;
#1816=CARTESIAN_POINT ( 'NONE',  ( -30.29861199217504009, 0.4131864886508529455, -6.889171040952208891 ) ) ;
#1818=CARTESIAN_POINT ( 'NONE',  ( 34.32017124965129540, -10.33516403750143198, -8.900617703435305117 ) ) ;
#1830=CIRCLE ( 'NONE', #39428, 18.00000000000003553 ) ;
#1838=CARTESIAN_POINT ( 'NONE',  ( 15.49054523282929807, 15.24218747636109050, -22.10330208559187426 ) ) ;
#1840=CARTESIAN_POINT ( 'NONE',  ( 6.309536247299392109, 19.51471286317475773, -29.99999999999999645 ) ) ;
#1846=CARTESIAN_POINT ( 'NONE',  ( 15.43059434986342104, -26.34277824748516039, -8.288079929563053838 ) ) ;
#1847=CARTESIAN_POINT ( 'NONE',  ( 37.48557158514985588, -11.25000000000009415, 0.000000000000000000 ) ) ;
#1849=CARTESIAN_POINT ( 'NONE',  ( -14.73215445377065258, 25.41255716721991220, -10.65209943420422434 ) ) ;
#1851=CARTESIAN_POINT ( 'NONE',  ( 14.23504194582299753, -26.35893216010225615, -6.418547458806204808 ) ) ;
#1855=CARTESIAN_POINT ( 'NONE',  ( -8.078176917764361420, 20.10266963944688356, -24.61727802958278133 ) ) ;
#1860=CARTESIAN_POINT ( 'NONE',  ( -26.92548543374830672, -4.182384202632584369, -16.97462146561391805 ) ) ;
#1863=CARTESIAN_POINT ( 'NONE',  ( 26.45401934139566791, 0.3544644617807020670, -15.45655976044637825 ) ) ;
#1869=CARTESIAN_POINT ( 'NONE',  ( -21.70835098058958934, 0.7322611594438664939, -23.85456472341968492 ) ) ;
#1873=CARTESIAN_POINT ( 'NONE',  ( 22.74168006064742187, -2.578368022317651054, -22.34712926292036883 ) ) ;
#1885=CARTESIAN_POINT ( 'NONE',  ( 5.995512085838934802, 36.57033614599139781, -7.995356539080317404 ) ) ;
#1890=CARTESIAN_POINT ( 'NONE',  ( 11.74422086145278499, -16.80344316252863734, -29.99999999999999289 ) ) ;
#1893=CARTESIAN_POINT ( 'NONE',  ( -35.48557158811166090, -13.25318502726451442, -4.999999999999997335 ) ) ;
#1896=CARTESIAN_POINT ( 'NONE',  ( 12.06198199496667023, 20.00631599209042832, -20.52696379477532673 ) ) ;
#1898=CARTESIAN_POINT ( 'NONE',  ( -14.84652007656822015, 25.07892745533905554, -10.66023937599700844 ) ) ;
#1901=CARTESIAN_POINT ( 'NONE',  ( 12.97456259195843131, 21.57840362866582140, -17.44539012491156171 ) ) ;
#1903=CARTESIAN_POINT ( 'NONE',  ( 31.48159048268411908, -18.63039699574827779, -9.724746473303273575 ) ) ;
#1905=CARTESIAN_POINT ( 'NONE',  ( -12.34485101014255015, 21.50093162914449962, -18.38636203722984774 ) ) ;
#1907=CARTESIAN_POINT ( 'NONE',  ( -15.27090603634302468, -24.25807912277981160, -13.38554782441437574 ) ) ;
#1910=CARTESIAN_POINT ( 'NONE',  ( -23.87677460445570432, -9.044431454778111501, -19.70507607847654441 ) ) ;
#1911=CARTESIAN_POINT ( 'NONE',  ( -10.43523929675511752, -20.08486062915910964, -21.66559121846610481 ) ) ;
#1913=CARTESIAN_POINT ( 'NONE',  ( 16.74741356090710909, 20.23878986518512590, -10.77388661789859547 ) ) ;
#1915=CARTESIAN_POINT ( 'NONE',  ( 29.41166959288484151, 1.126308269877565937, -7.836244769277370459 ) ) ;
#1919=CARTESIAN_POINT ( 'NONE',  ( -27.34250074455049884, -0.04617288401425825167, -14.44431459720212452 ) ) ;
#1921=CARTESIAN_POINT ( 'NONE',  ( 27.75004729309793561, -0.6577060458606293070, -14.37818117014819919 ) ) ;
#1926=CARTESIAN_POINT ( 'NONE',  ( -23.83078355888692812, 1.968671533367746695, -18.61202462238880528 ) ) ;
#1928=CARTESIAN_POINT ( 'NONE',  ( 9.163310636333564574, 20.63632441393291117, -20.55760979252978871 ) ) ;
#1936=CARTESIAN_POINT ( 'NONE',  ( -19.89457789833269885, 5.001894110080484346, -30.00000000000000355 ) ) ;
#1939=CARTESIAN_POINT ( 'NONE',  ( 15.08063968188699633, -13.89948965651085544, -29.23638960183474467 ) ) ;
#1945=CARTESIAN_POINT ( 'NONE',  ( 12.38141567392068687, 21.44998459107262079, -18.39378981892021514 ) ) ;
#1948=ORIENTED_EDGE ( 'NONE', *, *, #13340, .F. ) ;
#1949=CARTESIAN_POINT ( 'NONE',  ( -16.39082840404886454, 22.60326311949512856, -8.330118112291499344 ) ) ;
#1951=CARTESIAN_POINT ( 'NONE',  ( 9.747420686303255977, -18.58103426662601976, -26.22846927056824029 ) ) ;
#1953=CARTESIAN_POINT ( 'NONE',  ( 12.14677104559135223, 19.90516762884751145, -20.54385670340190728 ) ) ;
#1958=CARTESIAN_POINT ( 'NONE',  ( -10.92371859659766997, 17.40081432387707139, -28.70352546633995061 ) ) ;
#1960=CARTESIAN_POINT ( 'NONE',  ( -14.37944461722531209, -25.07460220977852572, -11.59761445704505434 ) ) ;
#1962=CARTESIAN_POINT ( 'NONE',  ( -17.56844388188584105, -11.33456651210386212, -26.97071349576603794 ) ) ;
#1963=CARTESIAN_POINT ( 'NONE',  ( -6.162728302860261742, -19.68972925932091655, -28.22432696427634724 ) ) ;
#1964=CARTESIAN_POINT ( 'NONE',  ( 13.25686098472626284, 20.17904452966509865, -18.55287099426779562 ) ) ;
#1966=CARTESIAN_POINT ( 'NONE',  ( 24.60674742379866942, 6.403599265695853582, -10.32857759193655767 ) ) ;
#1968=CYLINDRICAL_SURFACE ( 'NONE', #10172, 17.00000000000000000 ) ;
#1971=CARTESIAN_POINT ( 'NONE',  ( -28.56073700750507172, -2.042319486728655598, -14.24662277060652649 ) ) ;
#1973=CARTESIAN_POINT ( 'NONE',  ( 29.61024540805226479, 0.03371321916767414106, -10.18003961060840723 ) ) ;
#1987=CARTESIAN_POINT ( 'NONE',  ( 0.2523995269484193282, 23.75652376906266738, -21.83831241996571748 ) ) ;
#1994=CARTESIAN_POINT ( 'NONE',  ( 10.68390316795789907, 19.09395626910841059, -23.73008332297526835 ) ) ;
#1998=CARTESIAN_POINT ( 'NONE',  ( -17.59558984373777335, 14.85646055678510180, -16.92593635294098675 ) ) ;
#2002=CARTESIAN_POINT ( 'NONE',  ( 9.540684313847151543, -18.19539630009126796, -28.70617519958423358 ) ) ;
#2004=CARTESIAN_POINT ( 'NONE',  ( 11.01682622236871190, 17.44023727289612680, -28.07602756421292511 ) ) ;
#2007=CARTESIAN_POINT ( 'NONE',  ( -16.02710008567369471, -14.15296568158351675, -25.66971380233889377 ) ) ;
#2008=CARTESIAN_POINT ( 'NONE',  ( 1.777943910967427765, -24.47318281018553776, -8.902071781458595012 ) ) ;
#2009=CARTESIAN_POINT ( 'NONE',  ( 15.15225747352173080, 25.54735692720815621, -9.243652212863397111 ) ) ;
#2010=CARTESIAN_POINT ( 'NONE',  ( 16.79293355945483768, 12.02408141436283096, -27.16697041235419263 ) ) ;
#2014=CARTESIAN_POINT ( 'NONE',  ( -5.483409067041409735, 26.92266725723538912, -17.70185542587633520 ) ) ;
#2022=CARTESIAN_POINT ( 'NONE',  ( -28.99011627634691379, 0.4950866871714426076, -10.66519856541149203 ) ) ;
#2024=CARTESIAN_POINT ( 'NONE',  ( 21.66385282246533706, -6.550364480499578868, -23.14497041608409944 ) ) ;
#2038=CARTESIAN_POINT ( 'NONE',  ( 17.38826120058489977, 16.41976207655657305, -14.83715943985794006 ) ) ;
#2039=CARTESIAN_POINT ( 'NONE',  ( 7.074295817134445663, 19.80110017896302921, -26.49286407288892420 ) ) ;
#2044=CARTESIAN_POINT ( 'NONE',  ( 15.12144832649043913, -25.88752217724391969, -9.695795975739306627 ) ) ;
#2046=CARTESIAN_POINT ( 'NONE',  ( 12.05832241004688399, 18.99596958976722760, -21.04195414767209726 ) ) ;
#2047=CARTESIAN_POINT ( 'NONE',  ( -11.89245061573173956, 19.38187911134576069, -21.61709387797126425 ) ) ;
#2050=CARTESIAN_POINT ( 'NONE',  ( 11.73272494866245097, -22.55029353769394618, -16.51294986919664254 ) ) ;
#2056=CARTESIAN_POINT ( 'NONE',  ( -9.368025324006740817, 25.77638131019460843, -16.93723336282096881 ) ) ;
#2061=CARTESIAN_POINT ( 'NONE',  ( 21.26977380105256898, 0.8230692367304124346, -25.01963132466870121 ) ) ;
#2067=CARTESIAN_POINT ( 'NONE',  ( -22.21787668464120813, 0.6769409624482073395, -22.73667545006919255 ) ) ;
#2070=CARTESIAN_POINT ( 'NONE',  ( 24.27315791929659028, -3.535071426570953523, -20.06604538996125697 ) ) ;
#2083=CARTESIAN_POINT ( 'NONE',  ( 3.791040245356329663, 23.32460076806784599, -21.91667373837261223 ) ) ;
#2087=CARTESIAN_POINT ( 'NONE',  ( 12.56835645552544811, -16.80047637095704971, -26.57836621293479951 ) ) ;
#2093=CARTESIAN_POINT ( 'NONE',  ( 11.05230858265422711, 17.66332026264438682, -26.82356531899860741 ) ) ;
#2095=CARTESIAN_POINT ( 'NONE',  ( -13.72572330278604014, 22.36032731891220848, -15.48384944483169257 ) ) ;
#2098=CARTESIAN_POINT ( 'NONE',  ( 12.72840175812996755, 20.94423838021117845, -18.46516121132114208 ) ) ;
#2101=CARTESIAN_POINT ( 'NONE',  ( 23.60227988993529280, -14.95294269409316001, -17.59782747150006443 ) ) ;
#2103=CARTESIAN_POINT ( 'NONE',  ( -15.14733410328086549, 27.40717930319807749, -6.405640806656524688 ) ) ;
#2105=CARTESIAN_POINT ( 'NONE',  ( -12.40151229802639676, -20.21468385990432282, -20.38444596684770360 ) ) ;
#2106=LINE ( 'NONE', #30731, #24355 ) ;
#2108=CARTESIAN_POINT ( 'NONE',  ( -34.94561069989751445, -10.89217094161273103, -7.586357350432970215 ) ) ;
#2109=CARTESIAN_POINT ( 'NONE',  ( -13.90572124313496971, -24.99301111420016497, -11.61183353183253253 ) ) ;
#2113=CARTESIAN_POINT ( 'NONE',  ( 20.51349737526394179, 3.099829992517171728, -26.98082256979993687 ) ) ;
#2117=CARTESIAN_POINT ( 'NONE',  ( -30.06351586540304766, -0.04787271998934088807, -9.233772743391703841 ) ) ;
#2118=CARTESIAN_POINT ( 'NONE',  ( 29.03390384994953521, -0.7637727643468541494, -12.46392547968639164 ) ) ;
#2122=CARTESIAN_POINT ( 'NONE',  ( -21.05807794215131068, 2.162551090963098943, -25.15387685026987796 ) ) ;
#2127=DIRECTION ( 'NONE',  ( 1.000000000000000000, 0.000000000000000000, 0.000000000000000000 ) ) ;
#2131=CARTESIAN_POINT ( 'NONE',  ( -20.93483025502773742, 5.035493566568158386, -23.14963160484778015 ) ) ;
#2134=CARTESIAN_POINT ( 'NONE',  ( 26.03909628386253061, -25.46251251313952935, -7.164779507717623730 ) ) ;
#2138=CARTESIAN_POINT ( 'NONE',  ( 11.58716084138019831, 19.70196545170939473, -21.55946877410309881 ) ) ;
#2142=CARTESIAN_POINT ( 'NONE',  ( -16.33001031136068448, 22.49441389709989991, -8.808442500960499189 ) ) ;
#2146=CARTESIAN_POINT ( 'NONE',  ( 11.00857322187251164, 17.29338995577434446, -30.00000000000000000 ) ) ;
#2148=CARTESIAN_POINT ( 'NONE',  ( 11.47989394144910058, 18.44111857959348200, -23.85327845104781019 ) ) ;
#2150=CARTESIAN_POINT ( 'NONE',  ( -14.46546301679569346, 25.16057478527850932, -11.58477129654782978 ) ) ;
#2152=CARTESIAN_POINT ( 'NONE',  ( -14.95434924768307461, -25.85156499263970531, -9.704675056642397379 ) ) ;
#2155=CARTESIAN_POINT ( 'NONE',  ( -18.86238051352358269, -11.38456432792228945, -24.21681366675842284 ) ) ;
#2156=CARTESIAN_POINT ( 'NONE',  ( -11.57545763705510922, -25.81734924782649543, -5.000000000000000000 ) ) ;
#2158=CARTESIAN_POINT ( 'NONE',  ( 12.88915114296325015, 19.83580132678993735, -19.58108076636484896 ) ) ;
#2160=CARTESIAN_POINT ( 'NONE',  ( 24.92982005813157542, 6.438780434261885510, -8.860171362492041069 ) ) ;
#2161=CARTESIAN_POINT ( 'NONE',  ( 17.34253826539385201, 27.32041144647958575, -13.70816084473008800 ) ) ;
#2165=CARTESIAN_POINT ( 'NONE',  ( -23.09408679231368211, -0.7667527528709867646, -21.43583835363619983 ) ) ;
#2167=CARTESIAN_POINT ( 'NONE',  ( 21.72087342840458746, 0.6664541231550867861, -23.84654602765732179 ) ) ;
#2181=CARTESIAN_POINT ( 'NONE',  ( 0.2177955101729588394, 20.58580882239673926, -28.44449306209597239 ) ) ;
#2189=CARTESIAN_POINT ( 'NONE',  ( 14.58515322177743023, 27.60815066180548882, -8.705533694680715584 ) ) ;
#2192=CARTESIAN_POINT ( 'NONE',  ( -17.80184909226064960, 15.08711156140914689, -15.89312851988550968 ) ) ;
#2197=CARTESIAN_POINT ( 'NONE',  ( 14.90512858723619161, -25.84045694921644554, -9.707335597051320875 ) ) ;
#2199=CARTESIAN_POINT ( 'NONE',  ( 12.64006179627876314, 21.07329801286157434, -18.44930732498576376 ) ) ;
#2200=CARTESIAN_POINT ( 'NONE',  ( 6.155076441694338207, 21.71698211341367113, -30.00000000000000000 ) ) ;
#2204=CARTESIAN_POINT ( 'NONE',  ( -24.39385489856421074, -19.12778200130764006, -14.77000471112758007 ) ) ;
#2205=CARTESIAN_POINT ( 'NONE',  ( 1.706488926421375396, -23.94603835514126899, -11.88489013895719815 ) ) ;
#2206=CARTESIAN_POINT ( 'NONE',  ( 11.17946636088399615, 17.33251866449996825, -28.08565060215844866 ) ) ;
#2207=CARTESIAN_POINT ( 'NONE',  ( 17.93241811013781017, 10.94633007592474172, -24.41574245663013443 ) ) ;
#2210=CARTESIAN_POINT ( 'NONE',  ( -6.555649915732293387, 32.00450200170969595, -12.95390610774645879 ) ) ;
#2217=VERTEX_POINT ( 'NONE', #8019 ) ;
#2218=CARTESIAN_POINT ( 'NONE',  ( -20.60288636730601297, 0.9732602012211746256, -28.08358842701117553 ) ) ;
#2221=CARTESIAN_POINT ( 'NONE',  ( 35.51876124919839839, -10.74978321004375559, -5.000000000000007105 ) ) ;
#2235=CARTESIAN_POINT ( 'NONE',  ( 14.80471852002763100, 14.23397828709298629, -28.82854777094696885 ) ) ;
#2236=CARTESIAN_POINT ( 'NONE',  ( 10.76129760716440487, 27.89257969453655051, -14.07744184314324620 ) ) ;
#2239=CARTESIAN_POINT ( 'NONE',  ( -20.42711629762379744, 10.01608555171554471, -16.97676697675829871 ) ) ;
#2243=CARTESIAN_POINT ( 'NONE',  ( 9.940439430138624743, -18.49387460801144911, -26.20988832591048734 ) ) ;
#2246=CARTESIAN_POINT ( 'NONE',  ( -11.88487758710532027, 19.39000425891907042, -21.61563605934467702 ) ) ;
#2247=CARTESIAN_POINT ( 'NONE',  ( 11.89833276060662115, -23.50684206517228603, -14.55647595399420169 ) ) ;
#2251=CARTESIAN_POINT ( 'NONE',  ( -11.54439467976890654, 29.21207630366558305, -12.21176094404378354 ) ) ;
#2257=CARTESIAN_POINT ( 'NONE',  ( 30.83880836401509029, 0.02450782886024076290, -5.474181074949118653 ) ) ;
#2258=CARTESIAN_POINT ( 'NONE',  ( -1.829593030691901284E-15, 22.50000000000001066, 0.000000000000000000 ) ) ;
#2263=CARTESIAN_POINT ( 'NONE',  ( -22.72401455592816077, 0.6329401436149191262, -21.62019267060189165 ) ) ;
#2265=ORIENTED_EDGE ( 'NONE', *, *, #21986, .F. ) ;
#2266=CARTESIAN_POINT ( 'NONE',  ( 34.17835999317385642, -5.203673669061616991, -6.341916554725859356 ) ) ;
#2273=CARTESIAN_POINT ( 'NONE',  ( -17.00000000000000000, 22.50000000000000355, 10.00000000000000000 ) ) ;
#2280=CARTESIAN_POINT ( 'NONE',  ( 7.040733923968011787, 36.25288937278184420, -7.575589961396375749 ) ) ;
#2284=CARTESIAN_POINT ( 'NONE',  ( 18.69514969737914001, -27.26850006250750624, -5.000000000000007105 ) ) ;
#2290=CARTESIAN_POINT ( 'NONE',  ( 10.89778913317478626, 17.36343269013392643, -30.00000000000000000 ) ) ;
#2291=VERTEX_POINT ( 'NONE', #24067 ) ;
#2293=CARTESIAN_POINT ( 'NONE',  ( -15.39107358607109610, 26.18243249704805820, -7.359043735441920475 ) ) ;
#2298=CARTESIAN_POINT ( 'NONE',  ( 11.54739967089177810, 18.38288522691597748, -23.86353388501674644 ) ) ;
#2300=CARTESIAN_POINT ( 'NONE',  ( 25.52108459349270930, -16.17540792513675640, -15.67991740391578048 ) ) ;
#2302=CARTESIAN_POINT ( 'NONE',  ( -14.04492652393572527, 25.09326306025475972, -12.49859865225124267 ) ) ;
#2304=CARTESIAN_POINT ( 'NONE',  ( -17.46439735134465820, -26.04403205724830528, -10.03879580357975421 ) ) ;
#2307=CARTESIAN_POINT ( 'NONE',  ( -21.45327189537562518, -7.409941418364766719, -23.09511941793392253 ) ) ;
#2308=CARTESIAN_POINT ( 'NONE',  ( -14.88933002184502108, -26.10237849226964002, -8.769526409485358442 ) ) ;
#2311=CARTESIAN_POINT ( 'NONE',  ( 20.29617916935422528, 3.110535768804490786, -28.77477341303289293 ) ) ;
#2315=CARTESIAN_POINT ( 'NONE',  ( -30.08515734786159967, -0.07135867236674159342, -9.232266537557617170 ) ) ;
#2317=CARTESIAN_POINT ( 'NONE',  ( 20.73387816077086399, 0.03120835422459670647, -27.39522693578182455 ) ) ;
#2321=CARTESIAN_POINT ( 'NONE',  ( -20.33089032344865998, 3.598786340304104048, -27.59557066844887174 ) ) ;
#2334=CARTESIAN_POINT ( 'NONE',  ( -20.08579387813589179, 4.300271612531742171, -28.80311731544902187 ) ) ;
#2337=CARTESIAN_POINT ( 'NONE',  ( 25.39385983464903873, -24.87502355768076967, -8.913805553225882861 ) ) ;
#2340=CARTESIAN_POINT ( 'NONE',  ( 11.15208866170259761, 18.71877292872446574, -23.80158545199737574 ) ) ;
#2343=CARTESIAN_POINT ( 'NONE',  ( -16.95359871692699727, 21.80622970928592608, -6.428279578752638557 ) ) ;
#2348=CARTESIAN_POINT ( 'NONE',  ( 15.18952781818666331, 26.23141474697915498, -8.298106924336673629 ) ) ;
#2353=CARTESIAN_POINT ( 'NONE',  ( -14.79703636326500060, 25.74263473257225243, -10.17218918890135271 ) ) ;
#2355=CARTESIAN_POINT ( 'NONE',  ( -12.71873048370224346, -22.55951204540982147, -16.43669669196557237 ) ) ;
#2358=CARTESIAN_POINT ( 'NONE',  ( -17.77200783866643263, -10.72547896874518258, -27.70459291383746248 ) ) ;
#2359=CARTESIAN_POINT ( 'NONE',  ( -4.746940016115302363, -20.05784295341780776, -27.67719817960474415 ) ) ;
#2361=CARTESIAN_POINT ( 'NONE',  ( 13.38699610197189571, 19.18010719891643845, -19.66077882286520406 ) ) ;
#2363=CARTESIAN_POINT ( 'NONE',  ( 24.20446040187360026, 7.319688609815201197, -9.361820473650304564 ) ) ;
#2369=CARTESIAN_POINT ( 'NONE',  ( -27.18895464093139935, -0.8152009208677085672, -15.32376075612282662 ) ) ;
#2370=CARTESIAN_POINT ( 'NONE',  ( 25.89641589905429697, 0.2649541786267404220, -16.43670733185422961 ) ) ;
#2374=CARTESIAN_POINT ( 'NONE',  ( 35.84808252048253507, -3.038699442442316379, -13.99876745781542553 ) ) ;
#2377=DIRECTION ( 'NONE',  ( -0.000000000000000000, -0.000000000000000000, 1.000000000000000000 ) ) ;
#2380=CARTESIAN_POINT ( 'NONE',  ( 1.572519005230682332, 38.31547560893784521, -6.276489886563880738 ) ) ;
#2386=DIRECTION ( 'NONE',  ( 1.000000000000000000, 0.000000000000000000, 0.000000000000000000 ) ) ;
#2388=CARTESIAN_POINT ( 'NONE',  ( 14.62822902851280027, 28.63951968782866331, -6.846782395405623056 ) ) ;
#2391=CARTESIAN_POINT ( 'NONE',  ( -16.28833159386192975, 13.37804228123318318, -24.36285121532279518 ) ) ;
#2394=CARTESIAN_POINT ( 'NONE',  ( 15.25261056305548735, -26.39471828263916109, -7.827771010459708911 ) ) ;
#2396=CARTESIAN_POINT ( 'NONE',  ( 14.53140152873307578, 24.97328356840179353, -11.59890379914566338 ) ) ;
#2397=CARTESIAN_POINT ( 'NONE',  ( 11.87877828677522984, 19.39653357432699821, -21.61446414259498994 ) ) ;
#2399=CARTESIAN_POINT ( 'NONE',  ( -28.79410123593970638, 4.962698632456613801, -4.999999999999999112 ) ) ;
#2401=CARTESIAN_POINT ( 'NONE',  ( -29.70272037912319263, -23.25111303184518619, -6.708336780241142883 ) ) ;
#2402=CARTESIAN_POINT ( 'NONE',  ( 4.201337036921611201, -20.08771302450454499, -28.83765527686704999 ) ) ;
#2403=CARTESIAN_POINT ( 'NONE',  ( 11.68239538796815147, 18.26559943105741723, -23.88377865820274693 ) ) ;
#2404=CARTESIAN_POINT ( 'NONE',  ( 18.51501374778856146, 10.35893760720515466, -23.33396074953557431 ) ) ;
#2406=CARTESIAN_POINT ( 'NONE',  ( -5.159834554421613539, 22.03625837824066025, -23.14505616485400807 ) ) ;
#2414=CARTESIAN_POINT ( 'NONE',  ( -22.18768002425451513, 0.7994764990569520613, -22.75141326800756403 ) ) ;
#2416=CARTESIAN_POINT ( 'NONE',  ( 29.06859794668536878, -9.700207295447865974, -14.81230389778934686 ) ) ;
#2431=CARTESIAN_POINT ( 'NONE',  ( 19.75762832862930907, -16.14151280411838130, -19.70786949030270208 ) ) ;
#2432=CARTESIAN_POINT ( 'NONE',  ( 15.76482823105918385, 13.10325120709816105, -30.00000000000000711 ) ) ;
#2434=CARTESIAN_POINT ( 'NONE',  ( 11.57904490959511712, 30.10906470480531638, -11.27760544223991346 ) ) ;
#2437=CARTESIAN_POINT ( 'NONE',  ( -21.75201666326742966, 11.73857275933465871, -6.939711857671738038 ) ) ;
#2440=CARTESIAN_POINT ( 'NONE',  ( 15.74830575105852226, -26.80738400109229147, -5.472937640529008441 ) ) ;
#2448=CARTESIAN_POINT ( 'NONE',  ( -14.01060747619464486, 23.98181712051333747, -13.50887074865789828 ) ) ;
#2449=CARTESIAN_POINT ( 'NONE',  ( -23.04127009990159891, -25.77385733438709892, -8.962383121669381225 ) ) ;
#2450=CARTESIAN_POINT ( 'NONE',  ( 8.986720564395060507, -19.19316913704046001, -25.11960455031415407 ) ) ;
#2454=CARTESIAN_POINT ( 'NONE',  ( -10.29087960479974839, 28.35764963828314933, -14.04442573278240403 ) ) ;
#2459=CARTESIAN_POINT ( 'NONE',  ( 25.81175492159683316, 0.4056748218298066311, -16.45145585693692070 ) ) ;
#2464=CARTESIAN_POINT ( 'NONE',  ( -30.83932063798821943, -0.01157433484235278337, -5.946084096651039985 ) ) ;
#2468=CARTESIAN_POINT ( 'NONE',  ( 20.56644879191631858, -2.251167489236703734, -27.92353585182003428 ) ) ;
#2482=CARTESIAN_POINT ( 'NONE',  ( 4.284595636533838459, 26.24047331256504734, -18.68436667907231552 ) ) ;
#2485=CARTESIAN_POINT ( 'NONE',  ( 15.23343791758566823, -20.13306411397316609, -19.07499260615857395 ) ) ;
#2490=CARTESIAN_POINT ( 'NONE',  ( 12.62004824291777005, 21.10321597694743545, -18.44487059424978170 ) ) ;
#2493=CARTESIAN_POINT ( 'NONE',  ( -12.41076023834438047, 19.59308009719089583, -20.58983577532683285 ) ) ;
#2497=CARTESIAN_POINT ( 'NONE',  ( 13.83252988835445230, 23.26147414863088514, -14.48414622511842786 ) ) ;
#2499=CARTESIAN_POINT ( 'NONE',  ( 20.86300852440544418, -13.20907702042890186, -20.69370547666579441 ) ) ;
#2502=CARTESIAN_POINT ( 'NONE',  ( -14.85775003842022102, 28.53279358564904555, -5.000000000000001776 ) ) ;
#2504=CARTESIAN_POINT ( 'NONE',  ( -10.81924648548876355, -18.06583327712415254, -26.12370104260517678 ) ) ;
#2508=CARTESIAN_POINT ( 'NONE',  ( -35.48442078681456024, -11.08901139838818040, -5.000000000000004441 ) ) ;
#2509=CARTESIAN_POINT ( 'NONE',  ( -9.513019653046374202, -18.52389691873554156, -26.84529393937997099 ) ) ;
#2512=CARTESIAN_POINT ( 'NONE',  ( 29.78831017271203763, 1.106291696078458120, -5.473890122755831200 ) ) ;
#2516=CARTESIAN_POINT ( 'NONE',  ( -30.41772674068107918, -0.07296283099214972978, -8.294073688046619708 ) ) ;
#2517=EDGE_LOOP ( 'NONE', ( #30775, #35673 ) ) ;
#2518=CARTESIAN_POINT ( 'NONE',  ( 21.84932286874548879, -0.09515477611452517748, -23.75395710783811865 ) ) ;
#2521=CARTESIAN_POINT ( 'NONE',  ( -27.27092024678508153, 3.518473056539207722, -8.338086808340122502 ) ) ;
#2522=CARTESIAN_POINT ( 'NONE',  ( -19.48557158514988785, -11.24999999999987743, 10.00000000000000000 ) ) ;
#2532=CARTESIAN_POINT ( 'NONE',  ( -24.09052910358969157, 6.077159936355657877, -12.79381164378030533 ) ) ;
#2535=CARTESIAN_POINT ( 'NONE',  ( 15.61423674409565265, -15.29117231345428252, -24.39877605513977343 ) ) ;
#2537=CARTESIAN_POINT ( 'NONE',  ( 14.81862396006678750, 26.15963469534062469, -9.689294582542693490 ) ) ;
#2540=CARTESIAN_POINT ( 'NONE',  ( -14.72765650035312035, 19.61305159137336673, -16.65999048068721677 ) ) ;
#2544=CARTESIAN_POINT ( 'NONE',  ( 11.14342221288931967, 17.60014963584713499, -26.83212941470313240 ) ) ;
#2546=CARTESIAN_POINT ( 'NONE',  ( 11.07256710390411669, 17.50279746095967326, -27.44776494551611279 ) ) ;
#2548=CARTESIAN_POINT ( 'NONE',  ( -14.24127349493501526, 24.60312559476172467, -12.53936607505307776 ) ) ;
#2550=CARTESIAN_POINT ( 'NONE',  ( -9.705925585825449176, -18.43389087049540009, -26.82911780702928084 ) ) ;
#2554=CARTESIAN_POINT ( 'NONE',  ( -17.94496189389409579, -10.10876580532987390, -28.44359840047881249 ) ) ;
#2555=CARTESIAN_POINT ( 'NONE',  ( -8.614355843301860105, -20.92117845966354750, -20.81903466987984075 ) ) ;
#2556=DIRECTION ( 'NONE',  ( 0.000000000000000000, 0.000000000000000000, 1.000000000000000000 ) ) ;
#2557=CARTESIAN_POINT ( 'NONE',  ( 14.15128070507878633, 21.55177582895931465, -15.54190844270684302 ) ) ;
#2559=ORIENTED_EDGE ( 'NONE', *, *, #25538, .F. ) ;
#2560=CARTESIAN_POINT ( 'NONE',  ( 25.01923217006082112, 6.448405193624610732, -8.373492425512845116 ) ) ;
#2567=CARTESIAN_POINT ( 'NONE',  ( -30.68056625920112523, -0.7425512605776362074, -9.191107723028629550 ) ) ;
#2568=CARTESIAN_POINT ( 'NONE',  ( 30.85535809781197258, -0.09603343769173000588, -6.415643733099492430 ) ) ;
#2569=DIRECTION ( 'NONE',  ( 0.000000000000000000, 0.000000000000000000, 1.000000000000000000 ) ) ;
#2571=CARTESIAN_POINT ( 'NONE',  ( 37.62663912510992503, -8.659558992827964374, -5.000000000000018652 ) ) ;
#2573=ADVANCED_FACE ( 'NONE', ( #8829 ), #5968, .F. ) ;
#2576=CARTESIAN_POINT ( 'NONE',  ( 32.33143948541791701, 1.358872982501826865, -5.000000000000000000 ) ) ;
#2579=CARTESIAN_POINT ( 'NONE',  ( 32.33143948541783885, 1.358872982501748927, -5.000000000000000000 ) ) ;
#2580=CARTESIAN_POINT ( 'NONE',  ( 1.427212664744208492, 34.45065703016087610, -11.97499105156896881 ) ) ;
#2588=CARTESIAN_POINT ( 'NONE',  ( 11.74081726099163347, 22.30219342717537856, -18.27100175958907968 ) ) ;
#2591=CARTESIAN_POINT ( 'NONE',  ( -17.65798338100345788, 13.64237717712649811, -19.02918139907341910 ) ) ;
#2592=LINE ( 'NONE', #20687, #16816 ) ;
#2594=CARTESIAN_POINT ( 'NONE',  ( 10.54418320030637268, -19.57350299331167065, -22.73395184212085596 ) ) ;
#2595=CARTESIAN_POINT ( 'NONE',  ( 15.29107182738988158, 26.52751320015942937, -7.357832120508801310 ) ) ;
#2596=CARTESIAN_POINT ( 'NONE',  ( 11.04637056303654319, 17.52039979612685272, -27.44572375426643163 ) ) ;
#2601=CARTESIAN_POINT ( 'NONE',  ( -20.13935109294277481, -15.75254866237664153, -19.68832395494088772 ) ) ;
#2602=CARTESIAN_POINT ( 'NONE',  ( -0.2690799054783746258, -20.63332487587387121, -27.17690005459235181 ) ) ;
#2603=CARTESIAN_POINT ( 'NONE',  ( 11.21662988401310024, 17.21094317106729576, -28.71561903827853257 ) ) ;
#2604=CARTESIAN_POINT ( 'NONE',  ( 17.91334720694058902, 10.03521261366046069, -28.86326398646745872 ) ) ;
#2605=DIRECTION ( 'NONE',  ( -0.000000000000000000, -0.000000000000000000, 1.000000000000000000 ) ) ;
#2606=CARTESIAN_POINT ( 'NONE',  ( -3.472550923952060220, 20.28740512945706342, -28.47266432443047890 ) ) ;
#2608=CARTESIAN_POINT ( 'NONE',  ( -34.11471017283468399, -5.440626125914022282, -7.222970549378350036 ) ) ;
#2613=CARTESIAN_POINT ( 'NONE',  ( -29.40512185744006146, 0.2655052950593886907, -10.18551000707841503 ) ) ;
#2614=CARTESIAN_POINT ( 'NONE',  ( 35.28872890698186637, -12.99774170744852064, -6.288584514710181317 ) ) ;
#2618=ORIENTED_EDGE ( 'NONE', *, *, #10524, .T. ) ;
#2619=EDGE_CURVE ( 'NONE', #4159, #31948, #35256, .T. ) ;
#2628=CARTESIAN_POINT ( 'NONE',  ( 16.77110579274708968, -12.86178676763160134, -26.29076339887767233 ) ) ;
#2629=CARTESIAN_POINT ( 'NONE',  ( 19.05516563486750670, 15.43659885783165819, -10.86377891658857031 ) ) ;
#2630=CARTESIAN_POINT ( 'NONE',  ( 8.895693167633664800, 22.91615671184446867, -20.04609200397479540 ) ) ;
#2632=CARTESIAN_POINT ( 'NONE',  ( -22.31145927236271120, 10.79378405826409981, -6.938958974488863340 ) ) ;
#2635=CARTESIAN_POINT ( 'NONE',  ( 14.87691899169173659, -25.68218598931080976, -10.17324441562808701 ) ) ;
#2640=CARTESIAN_POINT ( 'NONE',  ( -14.83071926596090329, 25.63857572950853125, -10.17844402408916160 ) ) ;
#2641=CARTESIAN_POINT ( 'NONE',  ( -23.37310973299193151, -26.11789763318362745, -8.074212004804937948 ) ) ;
#2642=CARTESIAN_POINT ( 'NONE',  ( 9.006842323280976004, -18.63255999496335136, -27.49008004293749963 ) ) ;
#2647=CARTESIAN_POINT ( 'NONE',  ( -7.714721346952166492, 25.82618255026152454, -17.82262248225727674 ) ) ;
#2653=CARTESIAN_POINT ( 'NONE',  ( 29.98824418678894332, 0.03310433232545182541, -9.238498873535908373 ) ) ;
#2657=ORIENTED_EDGE ( 'NONE', *, *, #38722, .T. ) ;
#2658=CARTESIAN_POINT ( 'NONE',  ( -30.45863603936437869, 0.01568503498656502113, -7.827967170345961456 ) ) ;
#2661=CARTESIAN_POINT ( 'NONE',  ( 29.18684330182384912, -3.473580796607973920, -14.14225801422634632 ) ) ;
#2675=CARTESIAN_POINT ( 'NONE',  ( 7.188809461230587061, 31.68087858109696597, -12.96927761962711223 ) ) ;
#2679=CARTESIAN_POINT ( 'NONE',  ( 11.51504914472953267, -18.67855797424754627, -23.68894626656194546 ) ) ;
#2682=DIRECTION ( 'NONE',  ( 1.000000000000000000, 0.000000000000000000, 0.000000000000000000 ) ) ;
#2686=CARTESIAN_POINT ( 'NONE',  ( -15.34645457225791887, 26.58874063551486699, -6.887964196757459412 ) ) ;
#2688=CARTESIAN_POINT ( 'NONE',  ( 13.65468850750463936, -24.11061919912373597, -13.51576474134096273 ) ) ;
#2693=CARTESIAN_POINT ( 'NONE',  ( -14.33337269284760751, 29.34602042987353343, -6.833538065190099431 ) ) ;
#2694=DIRECTION ( 'NONE',  ( 1.000000000000000000, 0.000000000000000000, 0.000000000000000000 ) ) ;
#2695=CARTESIAN_POINT ( 'NONE',  ( -16.69208956396090926, -23.66209404026361796, -14.20132963311727714 ) ) ;
#2699=CARTESIAN_POINT ( 'NONE',  ( -28.05765197305022696, -9.635955780168286466, -15.75866516396918726 ) ) ;
#2700=CARTESIAN_POINT ( 'NONE',  ( -14.97948837623191132, -26.23672582955694921, -8.299150191911987662 ) ) ;
#2703=CARTESIAN_POINT ( 'NONE',  ( 28.88634399658755214, 1.998445312983448741, -6.421604194170203783 ) ) ;
#2707=CARTESIAN_POINT ( 'NONE',  ( -28.39807035044848860, 0.06794131916572514196, -12.54307312449454415 ) ) ;
#2709=CARTESIAN_POINT ( 'NONE',  ( 30.80942456744107005, -0.9143650800732036066, -9.182418516798353636 ) ) ;
#2714=CARTESIAN_POINT ( 'NONE',  ( -21.78239903333861349, 3.553677865574983663, -21.93178419694463344 ) ) ;
#2725=CARTESIAN_POINT ( 'NONE',  ( -19.95945058307471953, 5.721769224514986263, -26.53156390793591868 ) ) ;
#2726=CARTESIAN_POINT ( 'NONE',  ( 36.48557158514975640, -11.24999999999995559, 10.00000000000000000 ) ) ;
#2728=CARTESIAN_POINT ( 'NONE',  ( 14.69851482477425719, -14.40017170160419901, -28.50529416406689620 ) ) ;
#2730=CARTESIAN_POINT ( 'NONE',  ( 12.22522338894938088, 20.70977026341328653, -19.46168301453599625 ) ) ;
#2733=CARTESIAN_POINT ( 'NONE',  ( -16.03826714829968125, 24.67705000163143580, -5.474135182149290735 ) ) ;
#2737=CARTESIAN_POINT ( 'NONE',  ( 14.75231007449413312, 25.35299502146948925, -10.65417580594813174 ) ) ;
#2741=CARTESIAN_POINT ( 'NONE',  ( -10.90492496769149433, 17.35893878472046126, -29.34663910038763746 ) ) ;
#2742=DIRECTION ( 'NONE',  ( 0.000000000000000000, 0.000000000000000000, 1.000000000000000000 ) ) ;
#2743=CARTESIAN_POINT ( 'NONE',  ( -15.22980700598171211, -26.18112790717167826, -8.761347792469088347 ) ) ;
#2745=CARTESIAN_POINT ( 'NONE',  ( -21.52496464139200683, -12.12314022445560724, -20.68871519823034077 ) ) ;
#2746=CARTESIAN_POINT ( 'NONE',  ( -11.78551508893061417, -23.03824580411184186, -15.52955309715219023 ) ) ;
#2748=CARTESIAN_POINT ( 'NONE',  ( 12.28898657554147711, 17.72469657176861091, -23.97054147917551603 ) ) ;
#2750=CARTESIAN_POINT ( 'NONE',  ( 19.15330224686634963, 7.305649259636135540, -30.00000000000000000 ) ) ;
#2756=CARTESIAN_POINT ( 'NONE',  ( -25.04116001157528970, -0.6213440581654174899, -18.31437346914016828 ) ) ;
#2757=CARTESIAN_POINT ( 'NONE',  ( 23.36948692125722005, 0.4087503446080729130, -20.52222899045708715 ) ) ;
#2770=CARTESIAN_POINT ( 'NONE',  ( 3.295098241983883014, 32.08381273648824106, -13.82339927732507512 ) ) ;
#2778=CARTESIAN_POINT ( 'NONE',  ( 11.53528522782755417, 20.60494803806667008, -20.42540399034420773 ) ) ;
#2782=CARTESIAN_POINT ( 'NONE',  ( -19.34266190408123975, 15.30325114017860066, -9.874887699621096360 ) ) ;
#2785=CARTESIAN_POINT ( 'NONE',  ( 13.38383379236761961, -23.62348432274365351, -14.47560677120037731 ) ) ;
#2786=CARTESIAN_POINT ( 'NONE',  ( -22.16237596998683657, -26.26640487554014314, -8.538874403386357059 ) ) ;
#2789=CARTESIAN_POINT ( 'NONE',  ( 14.27584049633174246, 24.51164464966358025, -12.54715642964581157 ) ) ;
#2794=CARTESIAN_POINT ( 'NONE',  ( -28.22238894054767044, -23.52913000678562838, -8.433307499048945388 ) ) ;
#2795=CARTESIAN_POINT ( 'NONE',  ( -0.3713521775821578275, -24.14560739446480042, -10.88444230627014520 ) ) ;
#2796=CARTESIAN_POINT ( 'NONE',  ( 11.26908400546618871, 17.12495040990986794, -30.00000000000000355 ) ) ;
#2797=CARTESIAN_POINT ( 'NONE',  ( 19.58307402619674775, 12.02054371642003083, -15.94811493075723163 ) ) ;
#2798=EDGE_CURVE ( 'NONE', #8550, #34673, #11022, .T. ) ;
#2799=CARTESIAN_POINT ( 'NONE',  ( -3.563111756202009595, 20.80833165756875758, -26.31733160343138067 ) ) ;
#2801=CARTESIAN_POINT ( 'NONE',  ( -33.94661022151303342, -5.405014578827573857, -7.666919038779478335 ) ) ;
#2808=CARTESIAN_POINT ( 'NONE',  ( -29.94900022519512461, 0.8516863067260661557, -6.418642555037194164 ) ) ;
#2809=CARTESIAN_POINT ( 'NONE',  ( 19.23659220497393108, -7.112289578705962789, -30.00000000000000000 ) ) ;
#2822=CARTESIAN_POINT ( 'NONE',  ( -1.644293514239202558, 20.68013128552042446, -27.71419510687025323 ) ) ;
#2827=CARTESIAN_POINT ( 'NONE',  ( 29.14969154284566955, -23.82267159204295837, -6.287676784333006808 ) ) ;
#2828=CARTESIAN_POINT ( 'NONE',  ( 16.77886244865171150, 13.09686862389438211, -23.29364800532082569 ) ) ;
#2830=CARTESIAN_POINT ( 'NONE',  ( 10.66234920991248103, 30.15450380941021535, -12.15963120324809843 ) ) ;
#2832=CARTESIAN_POINT ( 'NONE',  ( -21.77806019913552404, 11.75179560353630848, -6.453505103389286290 ) ) ;
#2835=CARTESIAN_POINT ( 'NONE',  ( 12.38193221270099365, -22.02126375945465142, -17.42657776036095996 ) ) ;
#2837=CARTESIAN_POINT ( 'NONE',  ( 19.79815887584821610, 19.84782313723624370, -13.42901749168597192 ) ) ;
#2838=CARTESIAN_POINT ( 'NONE',  ( -15.40119896161133006, 26.83624744099596171, -5.473949411210034199 ) ) ;
#2840=CARTESIAN_POINT ( 'NONE',  ( -14.34583555374895525, -17.16037222123812356, -23.35150257132816876 ) ) ;
#2841=CARTESIAN_POINT ( 'NONE',  ( 10.66118309792825336, -25.49418724601090247, -7.379814460239313867 ) ) ;
#2847=CARTESIAN_POINT ( 'NONE',  ( -10.22043165594364034, 34.42610915102720526, -7.180433678547599285 ) ) ;
#2853=CARTESIAN_POINT ( 'NONE',  ( 22.21841090602945457, 0.6747637996796579385, -22.73641212969366876 ) ) ;
#2858=CARTESIAN_POINT ( 'NONE',  ( -26.47678993223912869, 0.3192213469539110227, -15.45381411608538968 ) ) ;
#2861=CARTESIAN_POINT ( 'NONE',  ( 24.34856821748838129, -4.279746131925105779, -19.99731643529021241 ) ) ;
#2873=DIRECTION ( 'NONE',  ( 0.000000000000000000, 0.000000000000000000, 1.000000000000000000 ) ) ;
#2876=CARTESIAN_POINT ( 'NONE',  ( 8.060800481109751559, 35.74480146002363767, -7.585522589778642910 ) ) ;
#2878=CARTESIAN_POINT ( 'NONE',  ( 14.68260282716209630, -21.83111036330549481, -17.17910696205039756 ) ) ;
#2884=CARTESIAN_POINT ( 'NONE',  ( -11.91667304890831680, 19.35618664243762765, -21.62132196524237671 ) ) ;
#2886=CARTESIAN_POINT ( 'NONE',  ( 14.88441567456970915, -26.21443660824652255, -8.299845255435092994 ) ) ;
#2890=CARTESIAN_POINT ( 'NONE',  ( -10.79837678754097574, 21.37684657782732245, -20.29484020400954236 ) ) ;
#2891=CARTESIAN_POINT ( 'NONE',  ( -12.22911246598414614, -17.74238687663815739, -24.74578340650955610 ) ) ;
#2892=CARTESIAN_POINT ( 'NONE',  ( 11.31392148919590923, 36.91540483778863546, -5.000000000000002665 ) ) ;
#2896=CARTESIAN_POINT ( 'NONE',  ( -34.27855427131117949, -9.549784089487717509, -8.912513341492028118 ) ) ;
#2897=CARTESIAN_POINT ( 'NONE',  ( -13.74267396692251531, -24.56729334661521946, -12.56146162201199878 ) ) ;
#2900=CARTESIAN_POINT ( 'NONE',  ( 30.42361321058833212, 0.1827335297003471470, -7.358803297337979998 ) ) ;
#2904=CARTESIAN_POINT ( 'NONE',  ( -29.67980999164576872, -0.04279675855848630306, -10.17325362659203414 ) ) ;
#2906=CARTESIAN_POINT ( 'NONE',  ( 21.43241828677356864, -0.7131419970486393423, -24.85227051139408516 ) ) ;
#2910=CARTESIAN_POINT ( 'NONE',  ( -25.82288576596329932, 3.514228647792512206, -12.69986980209609762 ) ) ;
#2924=CARTESIAN_POINT ( 'NONE',  ( -24.17774524110126322, 7.027723166510716268, -10.34013492986881744 ) ) ;
#2927=CARTESIAN_POINT ( 'NONE',  ( 14.10981997949339117, -15.61727850128731987, -26.45440405776506765 ) ) ;
#2929=CARTESIAN_POINT ( 'NONE',  ( 10.82808496700584477, 17.46135606781462712, -28.69954358548662299 ) ) ;
#2931=CARTESIAN_POINT ( 'NONE',  ( -15.87097346945386889, 23.44423284912781469, -9.272708727512497973 ) ) ;
#2934=CARTESIAN_POINT ( 'NONE',  ( 12.66836227548348326, 21.03152034328669018, -18.45485530985660461 ) ) ;
#2939=CARTESIAN_POINT ( 'NONE',  ( -12.82069841282840095, 21.83108406841477844, -17.41332505554854393 ) ) ;
#2942=CARTESIAN_POINT ( 'NONE',  ( -12.76993028032038602, -22.56078344509325007, -16.43107071015407783 ) ) ;
#2946=CARTESIAN_POINT ( 'NONE',  ( -26.35083455085015558, -14.83645574100917131, -15.67644099750071440 ) ) ;
#2947=CARTESIAN_POINT ( 'NONE',  ( -13.59131951343294276, -25.82231284968012019, -8.782825323748010504 ) ) ;
#2949=CARTESIAN_POINT ( 'NONE',  ( 15.68066481369410248, 23.61642061338914189, -9.744478434708410575 ) ) ;
#2951=CARTESIAN_POINT ( 'NONE',  ( 25.90794112815367356, 5.571130670237141480, -6.915715379737312318 ) ) ;
#2957=CARTESIAN_POINT ( 'NONE',  ( -20.64517791135504510, -0.4843551386664524672, -28.01037723252847655 ) ) ;
#2958=CARTESIAN_POINT ( 'NONE',  ( 31.05798941631825727, -0.2002603227334578129, -4.999999999999999112 ) ) ;
#2963=ORIENTED_EDGE ( 'NONE', *, *, #33839, .T. ) ;
#2964=CARTESIAN_POINT ( 'NONE',  ( 21.88444403592371756, 6.126538576424477966, -30.00000000000001066 ) ) ;
#2968=VERTEX_POINT ( 'NONE', #5923 ) ;
#2969=DIRECTION ( 'NONE',  ( -0.000000000000000000, -0.000000000000000000, -1.000000000000000000 ) ) ;
#2972=CARTESIAN_POINT ( 'NONE',  ( 1.462604112257996247, 20.70414128060931702, -27.71111028557563927 ) ) ;
#2980=CARTESIAN_POINT ( 'NONE',  ( 12.39613117785802920, 22.48878480139081759, -17.32547671766618791 ) ) ;
#2984=CARTESIAN_POINT ( 'NONE',  ( -17.84890069020828562, 18.10929763232169165, -10.32883059554979788 ) ) ;
#2989=CARTESIAN_POINT ( 'NONE',  ( 12.65230758151554014, -22.55754344927865063, -16.44404600518156201 ) ) ;
#2990=CARTESIAN_POINT ( 'NONE',  ( -20.38544652068658181, -25.64170277295648859, -10.37427513536433743 ) ) ;
#2992=CARTESIAN_POINT ( 'NONE',  ( 11.88256809692872729, 19.39247382671743480, -21.61519272832449445 ) ) ;
#2995=CARTESIAN_POINT ( 'NONE',  ( -13.64179698895352288, -24.10910305434091327, -13.51635134767616364 ) ) ;
#2997=CARTESIAN_POINT ( 'NONE',  ( -25.23528266485080707, -19.79492694554141607, -13.84032828069353194 ) ) ;
#2998=CARTESIAN_POINT ( 'NONE',  ( -0.2665898626985158115, -20.55074757747597758, -28.29937881637059505 ) ) ;
#2999=CARTESIAN_POINT ( 'NONE',  ( 15.19726048192972634, 25.40763732123437890, -9.245452804566358651 ) ) ;
#3000=CARTESIAN_POINT ( 'NONE',  ( 21.60539011535767528, 12.02606291333052368, -6.454038670498706054 ) ) ;
#3002=CARTESIAN_POINT ( 'NONE',  ( -4.822863700933563536, 33.73409833160523874, -12.00050471651474204 ) ) ;
#3004=CARTESIAN_POINT ( 'NONE',  ( -33.42954140234754590, -6.257036898190599494, -9.426039654913852317 ) ) ;
#3007=PLANE ( 'NONE',  #27811 ) ;
#3010=CARTESIAN_POINT ( 'NONE',  ( -23.70214251413468531, 1.055375858189379956, -19.56052323388921721 ) ) ;
#3011=CARTESIAN_POINT ( 'NONE',  ( 28.97475848703913925, -10.63545647045585874, -14.78716727546217946 ) ) ;
#3021=CARTESIAN_POINT ( 'NONE',  ( -1.624100677291493877, 20.43571491435562493, -30.00000000000000000 ) ) ;
#3025=CARTESIAN_POINT ( 'NONE',  ( 20.30746460111456742, -15.60079166006380724, -19.67824267733233157 ) ) ;
#3026=CARTESIAN_POINT ( 'NONE',  ( 19.69380245318583178, 14.63332033592687687, -9.880714762412520002 ) ) ;
#3027=CARTESIAN_POINT ( 'NONE',  ( 13.15697686552113588, 29.30913038656967018, -9.982777366939737718 ) ) ;
#3029=CARTESIAN_POINT ( 'NONE',  ( -17.64762046312857180, 10.49585427871703658, -28.86324443608691226 ) ) ;
#3031=CARTESIAN_POINT ( 'NONE',  ( 15.62075852780784047, -26.70067611967377985, -6.413895762741850248 ) ) ;
#3033=CARTESIAN_POINT ( 'NONE',  ( 20.55563217186196212, -29.52600041847795254, -5.000000000000015987 ) ) ;
#3034=CARTESIAN_POINT ( 'NONE',  ( 19.48557158514975285, -11.24999999999995737, 10.00000000000000000 ) ) ;
#3036=CARTESIAN_POINT ( 'NONE',  ( -15.22219195120841739, 26.44100515191062328, -7.826622911995333887 ) ) ;
#3037=VECTOR ( 'NONE', #17147, 1000.000000000000000 ) ;
#3038=CARTESIAN_POINT ( 'NONE',  ( -22.43675667947073293, -25.13256344364474160, -10.31126045143009051 ) ) ;
#3039=CARTESIAN_POINT ( 'NONE',  ( 10.20831112218712278, -21.62331746727261361, -18.60984041202089401 ) ) ;
#3043=CARTESIAN_POINT ( 'NONE',  ( -9.862325270099388419, 33.04988333219784380, -9.830511281312073635 ) ) ;
#3048=CARTESIAN_POINT ( 'NONE',  ( 24.55482339067931719, 0.4410777889133716823, -18.45331033963499223 ) ) ;
#3051=DIRECTION ( 'NONE',  ( 0.000000000000000000, 0.000000000000000000, -1.000000000000000000 ) ) ;
#3054=CARTESIAN_POINT ( 'NONE',  ( -27.12366736632709774, 0.2592640696602764305, -14.47817184671785817 ) ) ;
#3057=CARTESIAN_POINT ( 'NONE',  ( 20.52978982471044489, -3.550452485816113946, -27.17543462584250236 ) ) ;
#3075=CARTESIAN_POINT ( 'NONE',  ( 6.270378422840378718, 27.73110307447709744, -16.74549866864413517 ) ) ;
#3077=CARTESIAN_POINT ( 'NONE',  ( 11.37404163648363387, -17.38721229013356862, -27.31762905785370776 ) ) ;
#3082=CARTESIAN_POINT ( 'NONE',  ( -14.04545270995350670, 23.89835750463747743, -13.51489203531869521 ) ) ;
#3084=CARTESIAN_POINT ( 'NONE',  ( 10.06203327364132427, -19.22105317348337650, -23.87374111627889306 ) ) ;
#3088=CARTESIAN_POINT ( 'NONE',  ( -12.81438437627916294, 24.11148518490756842, -15.30534549235409614 ) ) ;
#3089=CARTESIAN_POINT ( 'NONE',  ( -20.01115666102352009, -26.54103525232406824, -8.595240658381658960 ) ) ;
#3095=CARTESIAN_POINT ( 'NONE',  ( -34.28623899043527956, -10.66410740567661897, -8.897208059971323024 ) ) ;
#3096=CARTESIAN_POINT ( 'NONE',  ( -15.07568792015453063, -26.56401150065150674, -6.417385571140632905 ) ) ;
#3099=CARTESIAN_POINT ( 'NONE',  ( 22.16878676813625049, 0.8754114111470541193, -22.76043277781719709 ) ) ;
#3104=CARTESIAN_POINT ( 'NONE',  ( -20.52801489595192308, 0.8352239444486609932, -28.70617517559551501 ) ) ;
#3106=CARTESIAN_POINT ( 'NONE',  ( 32.44839610264516239, -1.855716912065746627, -5.000000000000000000 ) ) ;
#3108=CARTESIAN_POINT ( 'NONE',  ( -10.99858019813223642, -17.35606952494162769, -30.00000000000001421 ) ) ;
#3111=CARTESIAN_POINT ( 'NONE',  ( -23.58591353912177624, 4.323729375759905125, -16.75487901750983966 ) ) ;
#3113=CARTESIAN_POINT ( 'NONE',  ( 19.48557158514982746, -11.25000000000009415, -5.000000000000000000 ) ) ;
#3121=CARTESIAN_POINT ( 'NONE',  ( -19.69137326279327027, 5.702251777040514114, -29.41124866415784567 ) ) ;
#3124=CARTESIAN_POINT ( 'NONE',  ( 22.74023349794498827, -25.07456572998067656, -10.30111323015509761 ) ) ;
#3127=CARTESIAN_POINT ( 'NONE',  ( 10.91336093707554333, 17.75825062284819467, -26.81050411434687675 ) ) ;
#3129=CARTESIAN_POINT ( 'NONE',  ( -15.43817069320426860, 22.63450057941196647, -11.66983478573951061 ) ) ;
#3132=CARTESIAN_POINT ( 'NONE',  ( 15.42533216934834250, 26.65747446338114557, -5.946092576581627931 ) ) ;
#3136=CARTESIAN_POINT ( 'NONE',  ( -15.00041699303972287, 26.46481294341050372, -8.753260597601569160 ) ) ;
#3138=CARTESIAN_POINT ( 'NONE',  ( -11.28598964761482470, -20.45078756188820535, -20.52814714296091836 ) ) ;
#3142=CARTESIAN_POINT ( 'NONE',  ( -33.84242992198449684, -16.42796269968979317, -7.975450335500420707 ) ) ;
#3143=CARTESIAN_POINT ( 'NONE',  ( -9.612297877367879551, -19.83582942224187207, -22.84230155296175369 ) ) ;
#3145=CARTESIAN_POINT ( 'NONE',  ( 13.63576238296606036, 20.52424253562647039, -17.54980119926154813 ) ) ;
#3148=CARTESIAN_POINT ( 'NONE',  ( 26.35199392063378099, 4.663862263929487995, -8.352515954957800304 ) ) ;
#3154=CARTESIAN_POINT ( 'NONE',  ( -30.06454056556724197, -0.2461126078811654294, -9.689261385093018930 ) ) ;
#3156=CARTESIAN_POINT ( 'NONE',  ( 27.92911499328061709, -0.05970110741965063694, -13.48672115538755278 ) ) ;
#3163=CARTESIAN_POINT ( 'NONE',  ( 13.47223693944937750, 18.09844039693851769, -21.24786896499729139 ) ) ;
#3165=ORIENTED_EDGE ( 'NONE', *, *, #15617, .T. ) ;
#3166=EDGE_CURVE ( 'NONE', #34935, #18367, #30408, .T. ) ;
#3172=CARTESIAN_POINT ( 'NONE',  ( 3.789724143065339224, 37.00233177767923110, -8.414891994916880336 ) ) ;
#3179=CARTESIAN_POINT ( 'NONE',  ( 14.18938711277078291, 25.87820699252437961, -11.53243986395856702 ) ) ;
#3183=CARTESIAN_POINT ( 'NONE',  ( -15.00437050688289986, 14.15087644790256682, -27.67883097521226787 ) ) ;
#3186=CARTESIAN_POINT ( 'NONE',  ( 12.66509161227769553, -22.55792390413381554, -16.44263127660910939 ) ) ;
#3187=CARTESIAN_POINT ( 'NONE',  ( -13.08565055680642786, -16.70549789365643178, -25.90368761856597146 ) ) ;
#3189=CARTESIAN_POINT ( 'NONE',  ( 11.02121864814410657, 17.43735474281069386, -28.07628969929118412 ) ) ;
#3191=ORIENTED_EDGE ( 'NONE', *, *, #10347, .T. ) ;
#3193=CARTESIAN_POINT ( 'NONE',  ( -9.901882729520171011, -18.83983749962000687, -25.02192390785083731 ) ) ;
#3196=ADVANCED_FACE ( 'NONE', ( #6001 ), #22998, .T. ) ;
#3197=CARTESIAN_POINT ( 'NONE',  ( -30.78128484184130187, -22.64136542128004592, -5.000000000000004441 ) ) ;
#3198=CARTESIAN_POINT ( 'NONE',  ( -0.3522767274228070788, -23.48013668842627766, -13.90457325883725659 ) ) ;
#3199=CARTESIAN_POINT ( 'NONE',  ( 15.53783880108225190, 26.09496515834549868, -6.417711193549261672 ) ) ;
#3201=CARTESIAN_POINT ( 'NONE',  ( 22.35343170176878402, 10.00543086905888934, -9.882773338075907077 ) ) ;
#3203=CARTESIAN_POINT ( 'NONE',  ( -2.860784471046919020, 20.39385230774454882, -28.46275780569326130 ) ) ;
#3205=CARTESIAN_POINT ( 'NONE',  ( -33.57168893143874300, -5.326829507069609448, -8.556972795487428840 ) ) ;
#3206=EDGE_CURVE ( 'NONE', #860, #31932, #12254, .T. ) ;
#3211=CARTESIAN_POINT ( 'NONE',  ( -28.80707638399428916, 0.7099290160774374137, -10.67124776689043841 ) ) ;
#3212=CARTESIAN_POINT ( 'NONE',  ( 28.79193172513320675, -11.56792772201013086, -14.76806894771908674 ) ) ;
#3222=CARTESIAN_POINT ( 'NONE',  ( -3.069715041284517110, 27.64360125249429601, -17.62585475904647225 ) ) ;
#3223=CARTESIAN_POINT ( 'NONE',  ( -33.51290647813895163, -3.280245463522580174, -4.999999999999997335 ) ) ;
#3227=CARTESIAN_POINT ( 'NONE',  ( 16.93876653066008586, 13.26377307663926963, -22.20805623995693168 ) ) ;
#3228=CARTESIAN_POINT ( 'NONE',  ( 9.509799170644791744, 22.48628651136178647, -20.11318651558298143 ) ) ;
#3230=CARTESIAN_POINT ( 'NONE',  ( -21.24184681333255753, 12.71378638656511484, -5.967672426067079705 ) ) ;
#3232=CARTESIAN_POINT ( 'NONE',  ( 9.633777947662931496, -18.14705080549017424, -28.70249247701261197 ) ) ;
#3234=CARTESIAN_POINT ( 'NONE',  ( 10.99485921934411081, 17.45463166253034260, -28.07471671999386942 ) ) ;
#3235=CARTESIAN_POINT ( 'NONE',  ( -8.937590682902627037, -20.71651963383551731, -30.00000000000000000 ) ) ;
#3237=CARTESIAN_POINT ( 'NONE',  ( -10.96701088540842761, 17.31978028264472513, -29.34797854174667364 ) ) ;
#3239=CARTESIAN_POINT ( 'NONE',  ( -23.78701751404137354, -26.53361121414976509, -6.322536473355526709 ) ) ;
#3240=CARTESIAN_POINT ( 'NONE',  ( 10.44141302741376798, -25.11139197116317590, -9.299239282066768197 ) ) ;
#3241=CARTESIAN_POINT ( 'NONE',  ( 11.19141198691837502, 17.56663717187159790, -26.83658983900039985 ) ) ;
#3243=CARTESIAN_POINT ( 'NONE',  ( 29.12903154260688154, -21.06488189102506681, -10.18399402962615596 ) ) ;
#3247=CARTESIAN_POINT ( 'NONE',  ( -11.11602857932560262, 33.89154083561517439, -6.322138485960394405 ) ) ;
#3252=CARTESIAN_POINT ( 'NONE',  ( 22.21294924997172515, 0.6970241196614612722, -22.73910473975576707 ) ) ;
#3256=CARTESIAN_POINT ( 'NONE',  ( -30.43251338895703739, 0.04316722816340590879, -7.828164403897452495 ) ) ;
#3259=CARTESIAN_POINT ( 'NONE',  ( 23.50560939881936662, -4.852381968592491823, -21.00978952430008562 ) ) ;
#3271=AXIS2_PLACEMENT_3D ( 'NONE', #29550, #14107, #2127 ) ;
#3273=CARTESIAN_POINT ( 'NONE',  ( 9.798388895788875175, 34.03070998536941261, -8.489266934394210651 ) ) ;
#3275=CARTESIAN_POINT ( 'NONE',  ( 17.12764558049190100, -26.53140043480064492, -8.684859237404365828 ) ) ;
#3279=CARTESIAN_POINT ( 'NONE',  ( -13.61578127026913698, 22.57276738262792648, -15.46832451228934069 ) ) ;
#3282=CARTESIAN_POINT ( 'NONE',  ( 10.35736673620512782, -19.62758828036890435, -22.75676071015052315 ) ) ;
#3287=CARTESIAN_POINT ( 'NONE',  ( -9.436104724621630524, 18.21145219648997227, -29.99999999999999289 ) ) ;
#3288=CARTESIAN_POINT ( 'NONE',  ( -19.44481637110248684, -27.25456932391892906, -5.912071530470661251 ) ) ;
#3291=CARTESIAN_POINT ( 'NONE',  ( -29.17235460288958393, -8.104917298035191564, -14.85913705212063718 ) ) ;
#3292=CARTESIAN_POINT ( 'NONE',  ( -9.537820998814829920, -18.38128399093912790, -27.45372482522294888 ) ) ;
#3295=CARTESIAN_POINT ( 'NONE',  ( 20.79851487167647406, 1.023505283316706205, -26.84526378395030832 ) ) ;
#3301=CARTESIAN_POINT ( 'NONE',  ( -20.61300406095988791, 0.8049965435648878120, -28.07524117914642403 ) ) ;
#3303=CARTESIAN_POINT ( 'NONE',  ( 32.71205163220476919, -2.303786481711429968, -5.920339140041507520 ) ) ;
#3304=CARTESIAN_POINT ( 'NONE',  ( 1.082866184310819824, -20.47455923100120856, -30.00000000000001066 ) ) ;
#3307=CARTESIAN_POINT ( 'NONE',  ( -24.01388090513056994, 4.332455551302775376, -15.73336986319053388 ) ) ;
#3318=CARTESIAN_POINT ( 'NONE',  ( -19.51080979133228510, 6.405414381276935742, -28.83855153441879438 ) ) ;
#3322=CARTESIAN_POINT ( 'NONE',  ( 13.88564487354877031, -15.37443428294943537, -27.83446942326135343 ) ) ;
#3325=CARTESIAN_POINT ( 'NONE',  ( 15.30622479779250256, 27.07165865151032591, -5.942729527624186936 ) ) ;
#3327=CARTESIAN_POINT ( 'NONE',  ( -16.22408403259154852, 24.10865257618694102, -5.474343353774658638 ) ) ;
#3330=CARTESIAN_POINT ( 'NONE',  ( 15.42009615191692085, 26.67611678986924062, -5.946089587727700021 ) ) ;
#3332=CARTESIAN_POINT ( 'NONE',  ( -36.48557158514989140, -11.24999999999987743, 6.000000000000000000 ) ) ;
#3334=CARTESIAN_POINT ( 'NONE',  ( -10.83390719878747355, 17.40340976726015398, -29.34510724894995093 ) ) ;
#3336=CARTESIAN_POINT ( 'NONE',  ( -12.82118876533016838, -22.56181011573424300, -16.42547678194880945 ) ) ;
#3339=CARTESIAN_POINT ( 'NONE',  ( -18.15436357158603897, -9.522238560471441460, -29.21298683338178037 ) ) ;
#3340=CARTESIAN_POINT ( 'NONE',  ( -10.98011883110523712, -24.81730312888366186, -10.73332943874482659 ) ) ;
#3341=DIRECTION ( 'NONE',  ( 1.000000000000000000, 0.000000000000000000, 0.000000000000000000 ) ) ;
#3342=CARTESIAN_POINT ( 'NONE',  ( 12.73900707961357170, 16.26579194631107228, -27.56360065120206571 ) ) ;
#3344=CARTESIAN_POINT ( 'NONE',  ( 22.23426282729013792, 5.324047925142390447, -18.87963228197226329 ) ) ;
#3351=CARTESIAN_POINT ( 'NONE',  ( -30.99844456375071289, -0.3171783591690320869, -6.879640249969712684 ) ) ;
#3352=CARTESIAN_POINT ( 'NONE',  ( 21.75224751592035588, 0.4974273606728234487, -23.82583798890098592 ) ) ;
#3356=CARTESIAN_POINT ( 'NONE',  ( -35.36940577612494963, -20.42053594592269761, -4.999999999999990230 ) ) ;
#3360=ADVANCED_FACE ( 'NONE', ( #40080 ), #8612, .T. ) ;
#3361=APPLICATION_CONTEXT ( 'automotive_design' ) ;
#3364=CARTESIAN_POINT ( 'NONE',  ( 3.871220829879935099, 38.02450267464935507, -5.000000000000000000 ) ) ;
#3372=CARTESIAN_POINT ( 'NONE',  ( 14.92380366935343972, 27.88910720575894686, -6.861436071230456513 ) ) ;
#3375=CARTESIAN_POINT ( 'NONE',  ( -15.08898831634408744, 14.27233443605820540, -26.54181874479749226 ) ) ;
#3379=CARTESIAN_POINT ( 'NONE',  ( 11.51930939957287059, -20.97998600509406586, -19.49970475651661417 ) ) ;
#3380=CARTESIAN_POINT ( 'NONE',  ( -17.40676172239622588, -21.99313558790002787, -16.01693467188644959 ) ) ;
#3381=CARTESIAN_POINT ( 'NONE',  ( 15.10367708458470126, 26.13036639895321045, -8.767987560003460246 ) ) ;
#3382=CARTESIAN_POINT ( 'NONE',  ( 11.02561053197542407, 17.43447018294412487, -28.07655181465922567 ) ) ;
#3385=CARTESIAN_POINT ( 'NONE',  ( -10.48080051920513611, -19.59187828654420116, -22.74178688489114819 ) ) ;
#3388=CARTESIAN_POINT ( 'NONE',  ( -29.96597079672651631, -20.69995294692298415, -9.731940980083196635 ) ) ;
#3389=CARTESIAN_POINT ( 'NONE',  ( 1.364045841937116643, -21.42539740769312928, -22.25265589050333404 ) ) ;
#3390=CARTESIAN_POINT ( 'NONE',  ( 11.35751580965241914, 17.11731054519655970, -28.72129911532366364 ) ) ;
#3391=CARTESIAN_POINT ( 'NONE',  ( 22.79531528405124163, 10.15988774222570434, -5.482352800657483094 ) ) ;
#3394=CARTESIAN_POINT ( 'NONE',  ( -26.51515768098519743, -2.574357228626084293, -17.10477876855104284 ) ) ;
#3398=VERTEX_POINT ( 'NONE', #10205 ) ;
#3401=CARTESIAN_POINT ( 'NONE',  ( -20.45512865215935960, 1.365572444264179452, -29.35734819944713081 ) ) ;
#3402=CARTESIAN_POINT ( 'NONE',  ( 35.06506416243693280, -12.90429163527686285, -7.138145798991673452 ) ) ;
#3415=CARTESIAN_POINT ( 'NONE',  ( -2.404449847303043786, 21.86890924017041016, -24.25077898173865520 ) ) ;
#3416=CARTESIAN_POINT ( 'NONE',  ( -35.48557158208988938, -9.180432008922831955, -4.999999999999999112 ) ) ;
#3420=CARTESIAN_POINT ( 'NONE',  ( 19.48557158514975285, -11.24999999999995737, 10.00000000000000000 ) ) ;
#3421=CARTESIAN_POINT ( 'NONE',  ( 9.798481364371980362, 21.31715715824844892, -21.26624317740214209 ) ) ;
#3422=ORIENTED_EDGE ( 'NONE', *, *, #639, .T. ) ;
#3424=CARTESIAN_POINT ( 'NONE',  ( -20.53340956023616215, 13.54976128206928188, -8.407384701756129175 ) ) ;
#3426=CARTESIAN_POINT ( 'NONE',  ( 9.684276948513423022, -18.21592224580517794, -28.07104506456108695 ) ) ;
#3428=CARTESIAN_POINT ( 'NONE',  ( 14.00096064495863857, 24.00543594118468249, -13.50663270117560266 ) ) ;
#3429=CARTESIAN_POINT ( 'NONE',  ( 15.72991998290128990, -16.18894361744929000, -29.99999999999998579 ) ) ;
#3432=CARTESIAN_POINT ( 'NONE',  ( -25.47853931120452131, -25.38973540270632512, -8.036541765355776690 ) ) ;
#3433=CARTESIAN_POINT ( 'NONE',  ( 12.61343103759603324, -25.39092838429157695, -9.744532428759812959 ) ) ;
#3434=CARTESIAN_POINT ( 'NONE',  ( 11.05718465110185988, 17.26235906992462787, -29.34992143215759697 ) ) ;
#3435=CARTESIAN_POINT ( 'NONE',  ( 30.70013347194538511, -22.17214586171431989, -7.124165660199366812 ) ) ;
#3440=CARTESIAN_POINT ( 'NONE',  ( -10.57541166117252729, 32.01915677600736387, -10.30941365822858202 ) ) ;
#3441=EDGE_CURVE ( 'NONE', #19220, #4159, #8599, .T. ) ;
#3448=CARTESIAN_POINT ( 'NONE',  ( 30.58188266183778836, 0.01734648026565401360, -7.358011334378191215 ) ) ;
#3452=CARTESIAN_POINT ( 'NONE',  ( -29.56002673421212634, 0.09025702458776063697, -10.18136869063499894 ) ) ;
#3456=CARTESIAN_POINT ( 'NONE',  ( 33.58038907436841214, -6.003017191285483278, -8.986547828497519319 ) ) ;
#3469=CARTESIAN_POINT ( 'NONE',  ( -6.675012889388576731, 19.39409273962604985, -29.99999999999996803 ) ) ;
#3472=CARTESIAN_POINT ( 'NONE',  ( 16.23240241217962065, 17.80559144519626003, -15.77666076426317154 ) ) ;
#3473=CARTESIAN_POINT ( 'NONE',  ( 9.133087869482302779, 35.68701272469542829, -5.442357614005382871 ) ) ;
#3475=CARTESIAN_POINT ( 'NONE',  ( 16.53758848021426076, -26.97586464850826005, -5.000000000000002665 ) ) ;
#3476=CARTESIAN_POINT ( 'NONE',  ( 30.90412082983250741, -0.04211290444289771118, -5.000000000000000000 ) ) ;
#3479=CARTESIAN_POINT ( 'NONE',  ( -14.30582960071693321, 24.43380170945625096, -12.55177947368377467 ) ) ;
#3482=CARTESIAN_POINT ( 'NONE',  ( 14.34480155068720286, -25.40677281950577537, -10.65920629769117411 ) ) ;
#3486=CARTESIAN_POINT ( 'NONE',  ( -11.60722801024130746, 21.49292312996424315, -19.33865458767208168 ) ) ;
#3487=CARTESIAN_POINT ( 'NONE',  ( -11.95652123975070324, -18.48273786211390401, -23.63287802302393814 ) ) ;
#3491=CARTESIAN_POINT ( 'NONE',  ( -35.33786424633182577, -8.799366064169335644, -5.000000000000002665 ) ) ;
#3492=CARTESIAN_POINT ( 'NONE',  ( -15.22285490720163459, -26.55223875496663055, -6.888230830752624101 ) ) ;
#3495=CARTESIAN_POINT ( 'NONE',  ( 20.73556080916292998, 1.704149916198021142, -26.89632919872368788 ) ) ;
#3500=CARTESIAN_POINT ( 'NONE',  ( -22.22587217777541468, 0.6446291972866406983, -22.73257526237749104 ) ) ;
#3502=CARTESIAN_POINT ( 'NONE',  ( 21.94068861260580405, -0.7738519978160267598, -23.67308330514575943 ) ) ;
#3504=CARTESIAN_POINT ( 'NONE',  ( 0.7366931383309426318, -20.49029098293467754, -30.00000000000001066 ) ) ;
#3507=CARTESIAN_POINT ( 'NONE',  ( -21.18796512248286490, 4.297847109112478137, -23.09674402144054994 ) ) ;
#3511=CARTESIAN_POINT ( 'NONE',  ( -20.57924982997939622, -27.21273881503329051, -4.999999999999998224 ) ) ;
#3517=CARTESIAN_POINT ( 'NONE',  ( -24.28809745169647627, 7.043314632023327526, -9.848050643796884884 ) ) ;
#3519=CARTESIAN_POINT ( 'NONE',  ( 22.96737774831856882, -25.31542735044140358, -9.848476247948095619 ) ) ;
#3521=CARTESIAN_POINT ( 'NONE',  ( 14.63926748296054292, 25.68772099636430895, -10.63428425608140593 ) ) ;
#3524=CARTESIAN_POINT ( 'NONE',  ( -12.71522534069617372, 17.33000003956545498, -24.02735807176059168 ) ) ;
#3527=CARTESIAN_POINT ( 'NONE',  ( 11.09886981330870626, 17.48507009481504682, -27.44980206485566399 ) ) ;
#3531=CARTESIAN_POINT ( 'NONE',  ( -11.16200477833207039, 18.15270254736048372, -24.99421180247795604 ) ) ;
#3533=CARTESIAN_POINT ( 'NONE',  ( -15.01611103430922256, -25.86512146738518680, -9.701370320124519608 ) ) ;
#3535=ORIENTED_EDGE ( 'NONE', *, *, #21959, .T. ) ;
#3536=CARTESIAN_POINT ( 'NONE',  ( -21.85483727830508016, -11.45635712499663050, -20.69655747118709854 ) ) ;
#3537=CARTESIAN_POINT ( 'NONE',  ( -14.53723555501347064, -26.50432973120043911, -5.474040766214040232 ) ) ;
#3539=CARTESIAN_POINT ( 'NONE',  ( 13.63685500492499436, 18.84978013948070341, -19.69852935831276852 ) ) ;
#3541=CARTESIAN_POINT ( 'NONE',  ( 20.84739969530572878, 5.252202929258718456, -23.16050360519607665 ) ) ;
#3547=CARTESIAN_POINT ( 'NONE',  ( -20.54032332987920029, 0.5213581391517280172, -28.69511755839404543 ) ) ;
#3549=CARTESIAN_POINT ( 'NONE',  ( 20.49022872340270851, 0.6388713974194965006, -30.00000000000000355 ) ) ;
#3555=CARTESIAN_POINT ( 'NONE',  ( 20.55563217186196212, -29.52600041847795254, -5.000000000000015987 ) ) ;
#3562=CARTESIAN_POINT ( 'NONE',  ( 5.356590097018567143, 32.51922113974988804, -12.93011007245527466 ) ) ;
#3572=CARTESIAN_POINT ( 'NONE',  ( 10.13018406787138304, 17.82246755199521360, -30.00000000000000000 ) ) ;
#3575=CARTESIAN_POINT ( 'NONE',  ( -18.24281883325805609, 17.05300135009716556, -10.83830628367119253 ) ) ;
#3578=CARTESIAN_POINT ( 'NONE',  ( 15.17886553297244845, -26.37689987109310152, -7.828163835162226469 ) ) ;
#3579=CARTESIAN_POINT ( 'NONE',  ( -12.82987974443481960, -16.39774487402648973, -27.21081390613418449 ) ) ;
#3580=CARTESIAN_POINT ( 'NONE',  ( 11.03878455726499652, 17.42581041319601809, -28.07733810068035041 ) ) ;
#3581=CARTESIAN_POINT ( 'NONE',  ( 11.16609885640999345, 17.76953549359777895, -26.22290328359227018 ) ) ;
#3585=CARTESIAN_POINT ( 'NONE',  ( -10.45876699675547705, -19.59826614722239313, -22.74446902591430586 ) ) ;
#3589=CARTESIAN_POINT ( 'NONE',  ( -16.22333673333531578, -12.66904231271439052, -28.46359972832643237 ) ) ;
#3590=CARTESIAN_POINT ( 'NONE',  ( -2.045961664570402849, -21.89947875929911447, -20.11636488654603028 ) ) ;
#3591=CARTESIAN_POINT ( 'NONE',  ( 15.67016653301135243, 25.89419373281741343, -5.474054512165222874 ) ) ;
#3593=CARTESIAN_POINT ( 'NONE',  ( 18.66638796832185676, 8.717581921939480338, -27.73010582896804976 ) ) ;
#3597=CARTESIAN_POINT ( 'NONE',  ( -32.09187415237648366, -4.172230308094091455, -10.40323351268730612 ) ) ;
#3603=CARTESIAN_POINT ( 'NONE',  ( -29.38781521346863101, 0.8835198419403300640, -8.779238543596127542 ) ) ;
#3604=CARTESIAN_POINT ( 'NONE',  ( 34.82234124989187052, -15.26616710914089303, -6.281458105108273848 ) ) ;
#3615=CARTESIAN_POINT ( 'NONE',  ( -2.850469738011612186, 35.13561800352367470, -11.07553433454840608 ) ) ;
#3622=CARTESIAN_POINT ( 'NONE',  ( 12.66562804284446919, 30.43173330721926462, -9.488869335771161317 ) ) ;
#3624=CARTESIAN_POINT ( 'NONE',  ( -17.99203688690355207, 9.826896140120286560, -29.42929808537602554 ) ) ;
#3626=CARTESIAN_POINT ( 'NONE',  ( 14.66907916930347255, -25.47038735071629034, -10.65037209538542662 ) ) ;
#3628=CARTESIAN_POINT ( 'NONE',  ( 14.99026664428914835, 26.05970091075412043, -9.233774695591788984 ) ) ;
#3629=CARTESIAN_POINT ( 'NONE',  ( -17.81784622497958281, -13.85677843414106292, -19.80438750953545579 ) ) ;
#3631=CARTESIAN_POINT ( 'NONE',  ( -14.12328112852335593, -14.97420427305475599, -28.52411008509453438 ) ) ;
#3632=CARTESIAN_POINT ( 'NONE',  ( 6.600279139084632263, -21.58199846485096529, -19.93465999699473912 ) ) ;
#3633=CARTESIAN_POINT ( 'NONE',  ( 11.14430626115242795, 17.35594636426317550, -28.08358351451018109 ) ) ;
#3634=CARTESIAN_POINT ( 'NONE',  ( 30.37984583882173339, -21.95053059032868958, -7.980260795864960066 ) ) ;
#3638=CARTESIAN_POINT ( 'NONE',  ( -9.111610322594222211, 34.24256388952155561, -8.919200168974919407 ) ) ;
#3642=AXIS2_PLACEMENT_3D ( 'NONE', #20643, #32636, #17602 ) ;
#3645=CARTESIAN_POINT ( 'NONE',  ( 20.52762855279893373, 0.8436669142239806574, -28.70647179655530579 ) ) ;
#3647=CARTESIAN_POINT ( 'NONE',  ( -14.95151364724921628, 28.45442998384966415, -4.999999999999998224 ) ) ;
#3651=CARTESIAN_POINT ( 'NONE',  ( -30.29894305497524698, 0.05251066091225892185, -8.298239616989643963 ) ) ;
#3652=CARTESIAN_POINT ( 'NONE',  ( -18.07439750081194418, -24.11643431694279727, -13.20271803662888743 ) ) ;
#3654=CARTESIAN_POINT ( 'NONE',  ( 34.73099849614892065, -6.268898363069737911, -5.449674842175516787 ) ) ;
#3655=ADVANCED_FACE ( 'NONE', ( #25839, #32145 ), #4309, .F. ) ;
#3664=CARTESIAN_POINT ( 'NONE',  ( 10.43479426945577693, 17.65763441714259940, -30.00000000000000711 ) ) ;
#3670=CARTESIAN_POINT ( 'NONE',  ( 13.75357712579410574, 15.21937127477098350, -29.39846290653906280 ) ) ;
#3671=CARTESIAN_POINT ( 'NONE',  ( 5.439076474902442726, 21.17935537869283991, -24.39656225441747495 ) ) ;
#3674=CARTESIAN_POINT ( 'NONE',  ( 15.98625244049591743, -26.19102206502670072, -9.191584109855959639 ) ) ;
#3677=CARTESIAN_POINT ( 'NONE',  ( -15.40280205795104074, 26.73783614089730420, -5.946216223248560695 ) ) ;
#3679=CARTESIAN_POINT ( 'NONE',  ( 9.545480319410255987, -18.37756454525665362, -27.45318142481432844 ) ) ;
#3683=CARTESIAN_POINT ( 'NONE',  ( -9.682888305682462615, 22.34984673401176991, -20.13486359021646521 ) ) ;
#3687=CARTESIAN_POINT ( 'NONE',  ( -19.75415558344636580, -5.512529345569482153, -30.00000000000000711 ) ) ;
#3688=CARTESIAN_POINT ( 'NONE',  ( -9.420974396635585890, -18.25674641473842286, -28.71086228043621347 ) ) ;
#3691=CARTESIAN_POINT ( 'NONE',  ( 29.62904701965947396, 0.2356813439005103483, -9.712952148242360195 ) ) ;
#3696=CARTESIAN_POINT ( 'NONE',  ( -20.97191788603130647, 0.7853576264891806158, -26.22290328094025824 ) ) ;
#3698=CARTESIAN_POINT ( 'NONE',  ( 32.44839610264516239, -1.855716912065746182, -5.464228481487916511 ) ) ;
#3699=CIRCLE ( 'NONE', #26403, 57.00000000000006395 ) ;
#3711=CARTESIAN_POINT ( 'NONE',  ( -23.40191561818073396, 8.913894316990450761, -7.907414655062425801 ) ) ;
#3712=CARTESIAN_POINT ( 'NONE',  ( 15.07134127176065164, -16.65659448856922609, -23.27637504703555038 ) ) ;
#3714=CARTESIAN_POINT ( 'NONE',  ( 15.36998952511977912, 26.94570423236723755, -5.473408146588083056 ) ) ;
#3717=CARTESIAN_POINT ( 'NONE',  ( -12.82656864439730171, 18.37706610567507326, -21.77094397810654769 ) ) ;
#3718=VECTOR ( 'NONE', #2605, 1000.000000000000000 ) ;
#3721=CARTESIAN_POINT ( 'NONE',  ( 11.14778535039169505, 17.59710828856957932, -26.83253580513521186 ) ) ;
#3726=CARTESIAN_POINT ( 'NONE',  ( -14.19928107862582323, 24.71232503731138763, -12.53013223596171244 ) ) ;
#3728=CARTESIAN_POINT ( 'NONE',  ( -9.913802546424228979, -17.94660116923212456, -30.00000000000000000 ) ) ;
#3731=ORIENTED_EDGE ( 'NONE', *, *, #16535, .T. ) ;
#3732=CARTESIAN_POINT ( 'NONE',  ( -33.10183492075854161, -16.06006169670122929, -9.286424115536252799 ) ) ;
#3733=CARTESIAN_POINT ( 'NONE',  ( -8.865215912320328684, -18.48469441140770542, -29.99999999999999645 ) ) ;
#3735=CARTESIAN_POINT ( 'NONE',  ( 15.07825382683082971, 21.60216847466018208, -13.62695226071541121 ) ) ;
#3737=CARTESIAN_POINT ( 'NONE',  ( 23.00984832986303985, 5.371918940450665758, -16.81477143931289220 ) ) ;
#3738=DIRECTION ( 'NONE',  ( 0.000000000000000000, 0.000000000000000000, 1.000000000000000000 ) ) ;
#3741=EDGE_LOOP ( 'NONE', ( #14548, #10987 ) ) ;
#3742=CARTESIAN_POINT ( 'NONE',  ( -31.14387024364657108, -0.3288088905222038560, -5.942067004542767705 ) ) ;
#3743=CARTESIAN_POINT ( 'NONE',  ( 27.99670244976675804, -0.1511120543668041383, -13.47709887780296611 ) ) ;
#3747=CARTESIAN_POINT ( 'NONE',  ( -15.72991998290134141, -16.18894361744923316, -30.00000000000001421 ) ) ;
#3756=CARTESIAN_POINT ( 'NONE',  ( 6.063463481279891987, 37.09571784679343409, -6.711698804117649075 ) ) ;
#3762=CARTESIAN_POINT ( 'NONE',  ( 25.46646149454646491, -19.62346392400056772, -13.83418298888276965 ) ) ;
#3766=CARTESIAN_POINT ( 'NONE',  ( 15.16389459841380116, 27.51912694620480337, -5.938229366125038489 ) ) ;
#3769=CARTESIAN_POINT ( 'NONE',  ( -17.11581301909970421, 15.65337108435191027, -16.89279340584462119 ) ) ;
#3773=CARTESIAN_POINT ( 'NONE',  ( 15.21573614595498647, -26.38579844286377707, -7.827967313425957308 ) ) ;
#3776=CARTESIAN_POINT ( 'NONE',  ( 14.03396390992467779, 23.92513025192832998, -13.51357501533718697 ) ) ;
#3778=CARTESIAN_POINT ( 'NONE',  ( 15.41110799979362511, 26.80090896191098793, -5.474125546455649527 ) ) ;
#3781=CARTESIAN_POINT ( 'NONE',  ( -11.10104332229198221, -20.48357726655720157, -20.55124491515338647 ) ) ;
#3784=CARTESIAN_POINT ( 'NONE',  ( -17.73645540159148482, -13.01725682536783424, -24.25077156562453240 ) ) ;
#3785=CARTESIAN_POINT ( 'NONE',  ( -1.783775571689018902, -20.56493600434025026, -27.73431482934296355 ) ) ;
#3786=CARTESIAN_POINT ( 'NONE',  ( 15.75662360411219787, 25.59993261007102561, -5.474038466411062842 ) ) ;
#3788=CARTESIAN_POINT ( 'NONE',  ( 21.98254353505891601, 9.874900589700915887, -11.87314829681821138 ) ) ;
#3793=CARTESIAN_POINT ( 'NONE',  ( -25.68856216064254383, -2.472509833716490579, -18.10827930001592634 ) ) ;
#3799=FACE_BOUND ( 'NONE', #26332, .T. ) ;
#3801=CARTESIAN_POINT ( 'NONE',  ( -27.13564390634777368, 1.007537100714265277, -13.55923196749210291 ) ) ;
#3802=CARTESIAN_POINT ( 'NONE',  ( 34.02878622761630822, -14.89681383196699294, -8.416776523781875241 ) ) ;
#3807=CARTESIAN_POINT ( 'NONE',  ( -16.42808373348810846, 23.48417063542603955, -5.000000000000001776 ) ) ;
#3812=CARTESIAN_POINT ( 'NONE',  ( -0.7453837511599995524, 37.93422878730011405, -7.543976147524814380 ) ) ;
#3820=CARTESIAN_POINT ( 'NONE',  ( 9.818323868757666162, 23.26050863160002535, -19.07506069204259092 ) ) ;
#3823=CARTESIAN_POINT ( 'NONE',  ( -18.05228600792142046, 10.74605824565360201, -24.41647870628840877 ) ) ;
#3826=CARTESIAN_POINT ( 'NONE',  ( 9.863624987970052160, -18.52888242359477289, -26.21732557761542282 ) ) ;
#3827=EDGE_CURVE ( 'NONE', #7027, #7392, #4915, .T. ) ;
#3829=CARTESIAN_POINT ( 'NONE',  ( 14.99499369208347233, 26.04445448530989182, -9.234529751571013634 ) ) ;
#3830=CARTESIAN_POINT ( 'NONE',  ( -7.289639608743041066, -27.06962010326280321, -5.000000000000000000 ) ) ;
#3832=CARTESIAN_POINT ( 'NONE',  ( -25.99994897708846864, -25.85974776871800884, -5.874774900483986428 ) ) ;
#3833=CARTESIAN_POINT ( 'NONE',  ( 6.264040290701674785, -20.94110484306758124, -22.06492468031074239 ) ) ;
#3834=CARTESIAN_POINT ( 'NONE',  ( 13.01827371381056864, 21.50808331926381101, -17.45255298520018172 ) ) ;
#3835=CARTESIAN_POINT ( 'NONE',  ( 31.44183620580527716, -21.28341506558783180, -7.121041165608909651 ) ) ;
#3838=EDGE_LOOP ( 'NONE', ( #19364, #23269 ) ) ;
#3839=CARTESIAN_POINT ( 'NONE',  ( -6.015615027858057573, 25.61324666952316420, -18.76221355029760929 ) ) ;
#3844=CARTESIAN_POINT ( 'NONE',  ( 30.73988743330639295, -0.04538756457274935319, -6.887853167781535113 ) ) ;
#3852=CARTESIAN_POINT ( 'NONE',  ( -20.52497589132623546, 0.8981380531211777818, -28.70837990097334114 ) ) ;
#3853=CARTESIAN_POINT ( 'NONE',  ( 34.47241746879583957, 3.460351812918713854, 0.000000000000000000 ) ) ;
#3855=CARTESIAN_POINT ( 'NONE',  ( 22.67047725821499427, -5.391315940321618427, -22.09846031373282926 ) ) ;
#3868=CARTESIAN_POINT ( 'NONE',  ( 14.42591706986332944, 14.96404800320749473, -26.50133422042014786 ) ) ;
#3869=CARTESIAN_POINT ( 'NONE',  ( 10.00952708242434319, 34.92643930758972459, -5.878487041382220113 ) ) ;
#3872=CARTESIAN_POINT ( 'NONE',  ( 15.61960274502122736, -25.98614172846138004, -9.670060679591365727 ) ) ;
#3877=CARTESIAN_POINT ( 'NONE',  ( -15.23583419380056014, 26.39386630455032545, -7.828192486749263601 ) ) ;
#3879=CARTESIAN_POINT ( 'NONE',  ( 13.81758775394617444, -24.97846941233739670, -11.61434847950435234 ) ) ;
#3882=ORIENTED_EDGE ( 'NONE', *, *, #16004, .F. ) ;
#3883=CARTESIAN_POINT ( 'NONE',  ( -11.26877388990210704, 26.23917836842477769, -15.09852949179583348 ) ) ;
#3884=CARTESIAN_POINT ( 'NONE',  ( -15.01668848176030480, -20.19012063094625020, -19.09890700315882128 ) ) ;
#3886=CARTESIAN_POINT ( 'NONE',  ( -30.95311370318828281, -7.619573582569746151, -13.02312855672049707 ) ) ;
#3889=CARTESIAN_POINT ( 'NONE',  ( 30.81169820973430973, 0.05224243800113870240, -4.999999999999999112 ) ) ;
#3893=CARTESIAN_POINT ( 'NONE',  ( -23.94792893277753265, 0.4690917673518810727, -19.49405232091567441 ) ) ;
#3898=CARTESIAN_POINT ( 'NONE',  ( 24.84710857777880832, -2.152420164953839254, -19.17158435834083718 ) ) ;
#3899=CARTESIAN_POINT ( 'NONE',  ( 13.71288650290049560, 15.24265236820024683, -30.00000000000001066 ) ) ;
#3904=CARTESIAN_POINT ( 'NONE',  ( -18.71275814301062823, -29.33771053242124793, -4.999999999999998224 ) ) ;
#3913=CARTESIAN_POINT ( 'NONE',  ( -21.66698873614936360, 9.458035595798465422, -13.88965424940386839 ) ) ;
#3914=CARTESIAN_POINT ( 'NONE',  ( 22.01692992093476775, -27.08823313053303750, -5.000000000000004441 ) ) ;
#3917=CARTESIAN_POINT ( 'NONE',  ( 12.57305715050316408, 21.17289748902732072, -18.43455663015607016 ) ) ;
#3919=CARTESIAN_POINT ( 'NONE',  ( -15.30439135265882378, 25.08127062006494157, -9.249767499845980012 ) ) ;
#3923=CARTESIAN_POINT ( 'NONE',  ( 11.51364707597612380, 18.41203290593636410, -23.85841619709769645 ) ) ;
#3925=CARTESIAN_POINT ( 'NONE',  ( 28.86970498031842780, -14.78348567515910794, -13.80807807713542879 ) ) ;
#3929=CARTESIAN_POINT ( 'NONE',  ( -13.02858025086399785, 22.56370760927372032, -16.40322947727175062 ) ) ;
#3931=CARTESIAN_POINT ( 'NONE',  ( -15.94649114141366830, -25.87861724480484327, -10.11375243002179936 ) ) ;
#3932=DIRECTION ( 'NONE',  ( 1.000000000000000000, 0.000000000000000000, 0.000000000000000000 ) ) ;
#3934=CARTESIAN_POINT ( 'NONE',  ( -18.43967439804336550, -8.978407292334223300, -29.21425099581027851 ) ) ;
#3935=CARTESIAN_POINT ( 'NONE',  ( -9.285084774773752159, -18.78246842825664942, -26.27069818453050587 ) ) ;
#3937=CARTESIAN_POINT ( 'NONE',  ( 15.52188586741623944, 21.55406148401431210, -12.66412526168250530 ) ) ;
#3939=CARTESIAN_POINT ( 'NONE',  ( 27.41035584056263374, 3.779750892310774990, -5.951374944377225695 ) ) ;
#3943=EDGE_CURVE ( 'NONE', #26001, #17093, #5260, .T. ) ;
#3944=CARTESIAN_POINT ( 'NONE',  ( -29.20369560020293065, -0.2713287649291702963, -11.56506784693800327 ) ) ;
#3946=CARTESIAN_POINT ( 'NONE',  ( 31.24124332302707785, -0.3963250197696455146, -5.471922067842784010 ) ) ;
#3950=CARTESIAN_POINT ( 'NONE',  ( -11.41987377193683528, -19.41918266173334828, -30.00000000000000000 ) ) ;
#3957=ADVANCED_FACE ( 'NONE', ( #8764, #5908 ), #5709, .T. ) ;
#3962=CARTESIAN_POINT ( 'NONE',  ( 26.39312466668815560, -24.39732993984534914, -8.895862594080151453 ) ) ;
#3965=CARTESIAN_POINT ( 'NONE',  ( 14.82073388239109768, 26.57690641049478586, -9.208629837656934214 ) ) ;
#3969=CARTESIAN_POINT ( 'NONE',  ( -17.81838900191993247, 19.71268737054005982, -5.955960509222737009 ) ) ;
#3973=CARTESIAN_POINT ( 'NONE',  ( 15.39214080485340475, -26.69224274047939360, -5.946089343969266139 ) ) ;
#3975=CARTESIAN_POINT ( 'NONE',  ( 11.48395950158329804, 18.43760140489433041, -23.85392656665083777 ) ) ;
#3976=VERTEX_POINT ( 'NONE', #2273 ) ;
#3977=CARTESIAN_POINT ( 'NONE',  ( 11.88635790708222295, 19.38841407910786785, -21.61592131405399542 ) ) ;
#3979=CARTESIAN_POINT ( 'NONE',  ( -15.36654411751621119, 26.86631301760015234, -5.944861291199306841 ) ) ;
#3981=CARTESIAN_POINT ( 'NONE',  ( -15.41413216001110165, -26.64907402180547891, -6.417196768553821151 ) ) ;
#3983=CARTESIAN_POINT ( 'NONE',  ( -30.13941039663480126, -22.19442074003340792, -7.981896383023998176 ) ) ;
#3984=CARTESIAN_POINT ( 'NONE',  ( -3.346448692850797713, -20.50037512799487160, -26.59278566100418928 ) ) ;
#3985=CARTESIAN_POINT ( 'NONE',  ( 15.28834851042550547, 25.12984405973253388, -9.249120326217479260 ) ) ;
#3987=CARTESIAN_POINT ( 'NONE',  ( 19.09019219243798560, 9.727682261722398138, -22.24254973901808796 ) ) ;
#3992=CARTESIAN_POINT ( 'NONE',  ( -33.95211651047912937, -4.501248717685172984, -5.902678725086724754 ) ) ;
#3996=DIRECTION ( 'NONE',  ( 0.000000000000000000, 0.000000000000000000, 1.000000000000000000 ) ) ;
#3997=EDGE_CURVE ( 'NONE', #4159, #34227, #38164, .T. ) ;
#3998=CARTESIAN_POINT ( 'NONE',  ( 18.84397998463681034, -8.285884587795221634, -28.45626337791865623 ) ) ;
#4002=ORIENTED_EDGE ( 'NONE', *, *, #639, .F. ) ;
#4004=CARTESIAN_POINT ( 'NONE',  ( -15.75423571344012785, 25.60460891297588049, -5.000000000000002665 ) ) ;
#4007=CARTESIAN_POINT ( 'NONE',  ( -0.6823421560338360781, 34.50290607385087327, -11.97315373814747019 ) ) ;
#4008=DIRECTION ( 'NONE',  ( 1.000000000000000000, 0.000000000000000000, 0.000000000000000000 ) ) ;
#4014=CARTESIAN_POINT ( 'NONE',  ( 9.933663752171780104, 19.02636276575347551, -24.83125579025524132 ) ) ;
#4017=CARTESIAN_POINT ( 'NONE',  ( -20.20272705719804307, 13.30714020733546299, -10.88308809810277289 ) ) ;
#4021=CARTESIAN_POINT ( 'NONE',  ( 15.55330811712816796, -26.75926366330655881, -5.000000000000000888 ) ) ;
#4023=CARTESIAN_POINT ( 'NONE',  ( 10.95101281418289219, 17.32990059288363582, -29.34763338141241462 ) ) ;
#4024=CARTESIAN_POINT ( 'NONE',  ( 6.023418944065099367, 39.81932404830325112, -4.999999999999995559 ) ) ;
#4026=CARTESIAN_POINT ( 'NONE',  ( -25.92870434171245364, -25.79656239075070445, -6.305900231137221645 ) ) ;
#4028=CARTESIAN_POINT ( 'NONE',  ( 8.448443376098214941, -25.22526105246425132, -6.914809992635317037 ) ) ;
#4029=CARTESIAN_POINT ( 'NONE',  ( 11.22630306440229120, 17.54214173034566215, -26.83981274308017007 ) ) ;
#4030=CARTESIAN_POINT ( 'NONE',  ( 17.75521226434697653, -11.99623302150457071, -25.58889124899400258 ) ) ;
#4034=CARTESIAN_POINT ( 'NONE',  ( -9.224180078094502022, 34.72823754788878148, -8.037642107661440605 ) ) ;
#4037=CARTESIAN_POINT ( 'NONE',  ( 29.39456445034288734, 0.02916568486956336997, -10.65018324265741967 ) ) ;
#4043=CARTESIAN_POINT ( 'NONE',  ( -27.63060058548921916, 0.3335000238941912554, -13.52159836282129568 ) ) ;
#4045=CARTESIAN_POINT ( 'NONE',  ( -19.86157371036397024, -26.35897367596445307, -9.048130446679126138 ) ) ;
#4047=CARTESIAN_POINT ( 'NONE',  ( 32.53700013911068112, -7.740585582578115798, -11.18790742163261598 ) ) ;
#4050=EDGE_LOOP ( 'NONE', ( #8322, #8178, #2265, #11305 ) ) ;
#4058=CARTESIAN_POINT ( 'NONE',  ( -11.63102264767868022, 16.88415827355038346, -29.99999999999999289 ) ) ;
#4062=CARTESIAN_POINT ( 'NONE',  ( 17.71502384555986964, 18.39420983132613330, -10.32349406737177411 ) ) ;
#4064=CARTESIAN_POINT ( 'NONE',  ( 10.89528107728888884, 34.21469084972675034, -5.883532326481708985 ) ) ;
#4070=CARTESIAN_POINT ( 'NONE',  ( 14.39497424806422110, -24.19987066023631073, -13.45455450271301068 ) ) ;
#4074=CARTESIAN_POINT ( 'NONE',  ( -15.33606198554360489, 26.62522709554853861, -6.887829150642375886 ) ) ;
#4077=CARTESIAN_POINT ( 'NONE',  ( 14.54843269636342207, -25.89572241968321720, -9.243644732761685745 ) ) ;
#4081=CARTESIAN_POINT ( 'NONE',  ( -12.92904967086177592, 30.39550629362422640, -9.046739157839594370 ) ) ;
#4082=CARTESIAN_POINT ( 'NONE',  ( -12.29725306327712708, -16.76881849169811645, -27.24954791152431355 ) ) ;
#4085=CARTESIAN_POINT ( 'NONE',  ( -20.37871563014435949, -4.364548208266203488, -27.13438481043609585 ) ) ;
#4089=CARTESIAN_POINT ( 'NONE',  ( 23.86586618233766188, 0.6644085514824049632, -19.51682805881153016 ) ) ;
#4093=CARTESIAN_POINT ( 'NONE',  ( -21.27703557833525849, 0.7712986363537081003, -25.01410140241630842 ) ) ;
#4097=CARTESIAN_POINT ( 'NONE',  ( 33.89061681622978028, -4.196143601155450931, -5.000000000000000888 ) ) ;
#4099=CARTESIAN_POINT ( 'NONE',  ( 10.98647152928294446, 17.30743895948372213, -29.99999999999999289 ) ) ;
#4111=CARTESIAN_POINT ( 'NONE',  ( -21.34187245812352529, 8.386113929568535852, -16.94052806468766548 ) ) ;
#4113=CARTESIAN_POINT ( 'NONE',  ( 12.90178368060855263, -16.18855991010415352, -27.88622185041034029 ) ) ;
#4116=CARTESIAN_POINT ( 'NONE',  ( 15.18601210727193518, 26.56355505085192448, -7.822568326478698708 ) ) ;
#4119=CARTESIAN_POINT ( 'NONE',  ( -12.11973687156280732, 16.88561127307271548, -26.91797464023488473 ) ) ;
#4122=CARTESIAN_POINT ( 'NONE',  ( 14.32550604534909944, 24.38408524461923932, -12.55371337434965540 ) ) ;
#4124=CARTESIAN_POINT ( 'NONE',  ( 18.24555790293216972, -9.366475481951450632, -29.21293379095443754 ) ) ;
#4127=CARTESIAN_POINT ( 'NONE',  ( -13.31479659943831528, 23.16958864656041328, -15.41030129701651141 ) ) ;
#4129=CARTESIAN_POINT ( 'NONE',  ( -10.68831967236590863, -19.00044293756837988, -23.79478829776460458 ) ) ;
#4133=CARTESIAN_POINT ( 'NONE',  ( -24.40510592067864337, -10.95802276781445350, -18.63885804247661682 ) ) ;
#4134=CARTESIAN_POINT ( 'NONE',  ( -11.02229136415891375, -21.55589928887741280, -18.53673214569949934 ) ) ;
#4136=CARTESIAN_POINT ( 'NONE',  ( 12.78138401561641757, 16.34997449607922704, -26.96911998264180355 ) ) ;
#4138=CARTESIAN_POINT ( 'NONE',  ( 22.55500308376087659, 3.759694506050656138, -19.82441702495482616 ) ) ;
#4142=CARTESIAN_POINT ( 'NONE',  ( -30.17172327769580065, -0.1653024818763443871, -9.226241714221277590 ) ) ;
#4144=CARTESIAN_POINT ( 'NONE',  ( 28.13187736273904349, -0.3339339482611098364, -13.45785432263379278 ) ) ;
#4148=CARTESIAN_POINT ( 'NONE',  ( -37.49625565938783467, -14.69322820095472792, -14.45070082761207964 ) ) ;
#4157=CARTESIAN_POINT ( 'NONE',  ( -19.48557158514998022, -11.24999999999982414, 0.000000000000000000 ) ) ;
#4159=VERTEX_POINT ( 'NONE', #37786 ) ;
#4162=CARTESIAN_POINT ( 'NONE',  ( 28.31258885558161253, -24.58735582524956342, -5.865897150960025286 ) ) ;
#4168=CARTESIAN_POINT ( 'NONE',  ( 13.53694675301034778, 23.90144292339553189, -14.42396455730128579 ) ) ;
#4171=CARTESIAN_POINT ( 'NONE',  ( -17.39859292866695029, 20.78101578164080010, -5.953700940668370301 ) ) ;
#4174=CARTESIAN_POINT ( 'NONE',  ( 12.63794253860312011, -22.55737441791748310, -16.44513747313600405 ) ) ;
#4176=CARTESIAN_POINT ( 'NONE',  ( 14.74027134064697364, 25.38771306981656650, -10.65372674069893755 ) ) ;
#4178=CARTESIAN_POINT ( 'NONE',  ( 15.17059102029336159, 26.29451859012213077, -8.297644773194724266 ) ) ;
#4181=CARTESIAN_POINT ( 'NONE',  ( -14.91084233014961669, 25.87661791010822654, -9.704681488575104709 ) ) ;
#4183=CARTESIAN_POINT ( 'NONE',  ( -14.04223362003087772, -24.61107474274603035, -12.55102269148551208 ) ) ;
#4186=CARTESIAN_POINT ( 'NONE',  ( -17.76475877421862748, -11.46159631620098374, -26.26136342777560273 ) ) ;
#4187=CARTESIAN_POINT ( 'NONE',  ( -7.027774925259491212, -25.12514353486302809, -6.439637200144365359 ) ) ;
#4188=CARTESIAN_POINT ( 'NONE',  ( 15.01879182178246630, 24.59331309867435067, -10.67126001090663756 ) ) ;
#4190=CARTESIAN_POINT ( 'NONE',  ( 23.27440278483144454, 9.195899915927737922, -7.420906811853504870 ) ) ;
#4191=CARTESIAN_POINT ( 'NONE',  ( 25.06933603554838541, -26.29324009030829146, -4.999999999999998224 ) ) ;
#4196=CARTESIAN_POINT ( 'NONE',  ( -30.02427499008684464, -3.855426316731294989, -13.18754434558245592 ) ) ;
#4204=CARTESIAN_POINT ( 'NONE',  ( 33.47631770321904554, -15.86963776861158948, -8.848939542670445135 ) ) ;
#4208=CARTESIAN_POINT ( 'NONE',  ( 40.48557158514985588, -11.25000000000009415, 0.000000000000000000 ) ) ;
#4210=AXIS2_PLACEMENT_3D ( 'NONE', #34070, #8487, #24325 ) ;
#4213=CARTESIAN_POINT ( 'NONE',  ( -0.4811758688950815710, 24.69766440587928003, -20.68953053046281809 ) ) ;
#4221=CARTESIAN_POINT ( 'NONE',  ( 14.48331725184759478, 29.32085274443433676, -4.999999999999998224 ) ) ;
#4225=CARTESIAN_POINT ( 'NONE',  ( -17.36159938413227266, 12.22522946688932421, -23.31441648596737437 ) ) ;
#4229=CARTESIAN_POINT ( 'NONE',  ( 9.646859339673033773, -18.23494634657538427, -28.07314365168607395 ) ) ;
#4231=CARTESIAN_POINT ( 'NONE',  ( 11.15752963301387624, 17.77571695416434849, -26.22197368321889144 ) ) ;
#4232=CARTESIAN_POINT ( 'NONE',  ( -9.163310636333559245, 20.63632441393290762, -20.55760979252981357 ) ) ;
#4234=CARTESIAN_POINT ( 'NONE',  ( -18.52376316179034177, -18.47445435019549720, -18.80462721719711539 ) ) ;
#4235=CARTESIAN_POINT ( 'NONE',  ( 7.081546805360019903, -19.44107384363185531, -27.60223205082446540 ) ) ;
#4236=CARTESIAN_POINT ( 'NONE',  ( 15.35505396563912406, 26.30757089143959604, -7.358616479543964140 ) ) ;
#4237=CARTESIAN_POINT ( 'NONE',  ( 17.50379027647891661, 11.61388887901797062, -24.40646131754820658 ) ) ;
#4241=CARTESIAN_POINT ( 'NONE',  ( -8.515066977056928721, 31.87126067055270795, -12.07705369524776629 ) ) ;
#4246=CARTESIAN_POINT ( 'NONE',  ( 27.17627001547444721, 0.1857076255850063362, -14.47139429581891434 ) ) ;
#4251=CARTESIAN_POINT ( 'NONE',  ( -20.52288541691031298, 0.9400963243053366281, -28.70984508064821839 ) ) ;
#4253=CARTESIAN_POINT ( 'NONE',  ( 34.53482489673403677, -8.269556898348005447, -8.054871878447405820 ) ) ;
#4262=CARTESIAN_POINT ( 'NONE',  ( -1.829593030691901284E-15, 22.50000000000001066, 0.000000000000000000 ) ) ;
#4264=CARTESIAN_POINT ( 'NONE',  ( -2.841037392928961403, 20.34467916404557286, -29.99999999999997158 ) ) ;
#4267=CARTESIAN_POINT ( 'NONE',  ( 14.14988989334844938, 15.91125535861774232, -24.19556275385872368 ) ) ;
#4268=CARTESIAN_POINT ( 'NONE',  ( 5.706445963761894724, 19.68930810918331531, -30.00000000000000000 ) ) ;
#4272=EDGE_CURVE ( 'NONE', #2217, #40031, #17634, .T. ) ;
#4273=CARTESIAN_POINT ( 'NONE',  ( 14.26185647276075663, -23.69475499396387264, -14.39420442332849603 ) ) ;
#4278=CARTESIAN_POINT ( 'NONE',  ( -15.17696341410569971, 26.27296005008451374, -8.298199770649093310 ) ) ;
#4281=CARTESIAN_POINT ( 'NONE',  ( 12.66313389477882190, -23.07460945457045653, -15.47333642705567947 ) ) ;
#4288=CARTESIAN_POINT ( 'NONE',  ( -13.38346974784127674, 29.27610552289402079, -9.538682096344105688 ) ) ;
#4291=CARTESIAN_POINT ( 'NONE',  ( -27.20639438528821330, -6.708910503866349906, -16.82195059597296805 ) ) ;
#4294=CARTESIAN_POINT ( 'NONE',  ( 30.63300256406853350, 0.06511367122978951871, -6.888153787381024351 ) ) ;
#4298=CARTESIAN_POINT ( 'NONE',  ( -20.48235837767022716, 0.8503560580662928858, -30.00000000000000000 ) ) ;
#4301=CARTESIAN_POINT ( 'NONE',  ( 29.81191106377080047, -1.966456811352005563, -12.36848069294839725 ) ) ;
#4309=PLANE ( 'NONE',  #9174 ) ;
#4317=CARTESIAN_POINT ( 'NONE',  ( -23.18566882249501049, 8.858897760092389717, -9.378430886998033955 ) ) ;
#4318=CARTESIAN_POINT ( 'NONE',  ( 20.90254793926122900, -27.22588555765620555, -5.454512999748705404 ) ) ;
#4319=CARTESIAN_POINT ( 'NONE',  ( -29.81236060003349664, -23.63427143558772414, -4.999999999999999112 ) ) ;
#4322=CARTESIAN_POINT ( 'NONE',  ( 14.76369794107131561, 25.84371132707958907, -10.16615331278799239 ) ) ;
#4324=CARTESIAN_POINT ( 'NONE',  ( -15.48761799580068477, 24.52726732821879807, -9.257161483001100422 ) ) ;
#4327=CARTESIAN_POINT ( 'NONE',  ( 11.94259084243876856, 19.32869477811282977, -21.62580263860968444 ) ) ;
#4329=CARTESIAN_POINT ( 'NONE',  ( 33.06617957498816907, -16.93606499636205598, -8.844916697856577414 ) ) ;
#4332=CARTESIAN_POINT ( 'NONE',  ( -10.72725030361012521, 17.46952664121795351, -29.34280788466693579 ) ) ;
#4334=CARTESIAN_POINT ( 'NONE',  ( -9.913527807423552218, -18.50616620477535790, -26.21249535246115414 ) ) ;
#4337=AXIS2_PLACEMENT_3D ( 'NONE', #26273, #37966, #2694 ) ;
#4339=CARTESIAN_POINT ( 'NONE',  ( -19.27950440941545551, -8.679414676085837499, -26.27594640052829433 ) ) ;
#4340=CARTESIAN_POINT ( 'NONE',  ( -13.28943834162129711, -24.06829275115873656, -13.53237098977819386 ) ) ;
#4342=CARTESIAN_POINT ( 'NONE',  ( 17.28126569830730475, 21.10767333569910065, -5.000000000000001776 ) ) ;
#4344=CARTESIAN_POINT ( 'NONE',  ( 27.51428991693143189, 2.898098800209003123, -9.288493378121359001 ) ) ;
#4345=CARTESIAN_POINT ( 'NONE',  ( 0.000000000000000000, 22.50000000000000355, 10.00000000000000000 ) ) ;
#4348=CARTESIAN_POINT ( 'NONE',  ( -30.27520739190695309, -0.08482538932227430550, -8.762168245153070245 ) ) ;
#4349=CARTESIAN_POINT ( 'NONE',  ( 22.33442608700813281, 0.1860125554426316219, -22.67341905481720232 ) ) ;
#4353=CARTESIAN_POINT ( 'NONE',  ( -35.84808252048276955, -3.038699442442197807, -13.99876745781545218 ) ) ;
#4365=CARTESIAN_POINT ( 'NONE',  ( 25.15787673397105451, -23.28870960197653162, -11.13244146939240764 ) ) ;
#4366=AXIS2_PLACEMENT_3D ( 'NONE', #26553, #29797, #38939 ) ;
#4370=CARTESIAN_POINT ( 'NONE',  ( 14.86216115821774331, 26.87648892286942726, -8.735628851188740995 ) ) ;
#4373=CARTESIAN_POINT ( 'NONE',  ( -14.47038813004304991, 14.64214536189450122, -28.23916130782108880 ) ) ;
#4377=CARTESIAN_POINT ( 'NONE',  ( 13.29078025355574155, -23.61538305050886422, -14.48073411885799544 ) ) ;
#4379=CARTESIAN_POINT ( 'NONE',  ( 11.69518638600979621, 18.90277557641397266, -22.73667561340743859 ) ) ;
#4381=CARTESIAN_POINT ( 'NONE',  ( 11.11294864066589483, 17.62134810521215655, -26.82927740383777504 ) ) ;
#4383=CARTESIAN_POINT ( 'NONE',  ( -14.26202392583869027, 24.54848877817957487, -12.54400935092919944 ) ) ;
#4385=CARTESIAN_POINT ( 'NONE',  ( -12.24423225742669885, -22.02408646944725845, -17.44156587861991170 ) ) ;
#4388=CARTESIAN_POINT ( 'NONE',  ( -17.22654052972206173, -11.11309616262812838, -29.21339801432243988 ) ) ;
#4389=CARTESIAN_POINT ( 'NONE',  ( -2.347924344150951192, -23.48319297452375309, -13.90098067855863029 ) ) ;
#4390=CARTESIAN_POINT ( 'NONE',  ( 15.01671707947095769, 23.68701959088559406, -11.63761327091711095 ) ) ;
#4392=CARTESIAN_POINT ( 'NONE',  ( 23.39763224849028234, 9.229310415396369649, -5.481604761177553797 ) ) ;
#4393=CARTESIAN_POINT ( 'NONE',  ( 30.24562352346015714, -23.15372967338634780, -5.000000000000000000 ) ) ;
#4394=CARTESIAN_POINT ( 'NONE',  ( -15.44574896850336287, -26.73167447641225536, -4.999999999999999112 ) ) ;
#4397=CARTESIAN_POINT ( 'NONE',  ( -20.48034806427134313, -1.125288817275917008, -29.31181698211635833 ) ) ;
#4404=CIRCLE ( 'NONE', #25166, 18.00000000000002842 ) ;
#4407=CARTESIAN_POINT ( 'NONE',  ( 19.23661869638189970, -7.777357332202925022, -27.73122278007569719 ) ) ;
#4416=CARTESIAN_POINT ( 'NONE',  ( -1.011306241801401606, 20.48440008317826511, -29.21294264354560966 ) ) ;
#4417=CARTESIAN_POINT ( 'NONE',  ( 19.48557158514988075, -11.24999999999998224, 3.000000000000000000 ) ) ;
#4423=CARTESIAN_POINT ( 'NONE',  ( 14.43593167022227952, 29.20741364694840314, -6.379814831040929946 ) ) ;
#4424=CARTESIAN_POINT ( 'NONE',  ( 35.07906678349414165, -7.111640533860041913, -4.999999999999997335 ) ) ;
#4427=CARTESIAN_POINT ( 'NONE',  ( -20.20456973212974106, 14.66708349146731827, -4.999999999999997335 ) ) ;
#4431=CARTESIAN_POINT ( 'NONE',  ( 14.81584271249959883, -25.66902196032313554, -10.17682674198090709 ) ) ;
#4433=CARTESIAN_POINT ( 'NONE',  ( 13.46442396743949210, 22.87082214237680944, -15.44440089725282839 ) ) ;
#4435=CARTESIAN_POINT ( 'NONE',  ( -35.36940577612494963, -20.42053594592269761, -4.999999999999990230 ) ) ;
#4438=CARTESIAN_POINT ( 'NONE',  ( -19.80406076264881321, -17.52161466429418724, -18.72497143683012411 ) ) ;
#4439=CARTESIAN_POINT ( 'NONE',  ( 8.142828335362517933, -24.61856252981078441, -10.30834616846729546 ) ) ;
#4440=CARTESIAN_POINT ( 'NONE',  ( 14.62685016563947116, 24.71383867966243386, -11.60661454720508345 ) ) ;
#4441=CARTESIAN_POINT ( 'NONE',  ( 17.36173719094433210, 11.50338824233619661, -25.50370862539636363 ) ) ;
#4442=FACE_OUTER_BOUND ( 'NONE', #7359, .T. ) ;
#4445=CARTESIAN_POINT ( 'NONE',  ( -5.424629926632633214, 20.35751203620437266, -26.39731167115077781 ) ) ;
#4447=CARTESIAN_POINT ( 'NONE',  ( -9.439731518140417776, -18.24720977618391515, -28.71013559075634802 ) ) ;
#4450=CARTESIAN_POINT ( 'NONE',  ( 29.84386241824243768, -0.001863274244196008950, -9.706340305527046297 ) ) ;
#4454=CARTESIAN_POINT ( 'NONE',  ( -30.70419509168079841, 0.1269851510385121840, -5.946116814806951645 ) ) ;
#4456=CARTESIAN_POINT ( 'NONE',  ( 34.88440358479222425, -8.370710937437479515, -7.181291740870185514 ) ) ;
#4469=CARTESIAN_POINT ( 'NONE',  ( 0.000000000000000000, 0.000000000000000000, 0.000000000000000000 ) ) ;
#4473=CARTESIAN_POINT ( 'NONE',  ( 16.97505978179442110, 15.88883797548840526, -16.88581435752053039 ) ) ;
#4474=CARTESIAN_POINT ( 'NONE',  ( 6.476106366349275056, 22.41237707052495409, -22.08317005786570775 ) ) ;
#4479=CARTESIAN_POINT ( 'NONE',  ( 13.07819759976932694, -21.99233217153179609, -17.34750951402496000 ) ) ;
#4484=CARTESIAN_POINT ( 'NONE',  ( -11.48643516040400669, 18.43546103647281953, -23.85432110392739347 ) ) ;
#4487=CARTESIAN_POINT ( 'NONE',  ( 10.18006096829566332, -19.67814488976349452, -22.77776888065764638 ) ) ;
#4489=ORIENTED_EDGE ( 'NONE', *, *, #8305, .F. ) ;
#4492=CARTESIAN_POINT ( 'NONE',  ( -13.01238674544895169, 30.61633392914591667, -8.594047575497109293 ) ) ;
#4493=CARTESIAN_POINT ( 'NONE',  ( -14.02522277065907019, -18.92975099516724313, -21.21400967010290373 ) ) ;
#4495=CARTESIAN_POINT ( 'NONE',  ( -33.66249016428778873, -7.316504645895227199, -9.400858107290300580 ) ) ;
#4498=CARTESIAN_POINT ( 'NONE',  ( 28.77352987854749600, 0.2413197295406705467, -11.60410763981559867 ) ) ;
#4503=CARTESIAN_POINT ( 'NONE',  ( -30.90411674721317326, -0.04211297212934830836, -4.999999999999999112 ) ) ;
#4506=CARTESIAN_POINT ( 'NONE',  ( 27.24177960840210133, -2.437714896029509415, -16.14381839494960857 ) ) ;
#4518=DIRECTION ( 'NONE',  ( 1.000000000000000000, 0.000000000000000000, 0.000000000000000000 ) ) ;
#4521=CARTESIAN_POINT ( 'NONE',  ( 4.392928914044564870, 32.84871041364772282, -12.91564532669888443 ) ) ;
#4524=CARTESIAN_POINT ( 'NONE',  ( -21.91691631266333218, 8.533117302549259264, -14.88445492063216058 ) ) ;
#4525=CARTESIAN_POINT ( 'NONE',  ( 20.45602243971594802, -26.70709334009890412, -8.136195482540582447 ) ) ;
#4527=CARTESIAN_POINT ( 'NONE',  ( 14.65949890303364711, 25.62925135841399182, -10.63803580328918130 ) ) ;
#4529=CARTESIAN_POINT ( 'NONE',  ( -11.73368784223909600, 16.86169632780890026, -28.73611812094127060 ) ) ;
#4532=CARTESIAN_POINT ( 'NONE',  ( -75.15099915297791711, 43.38844959084113384, 0.000000000000000000 ) ) ;
#4533=CARTESIAN_POINT ( 'NONE',  ( 15.05161315844539693, 25.86266507323037800, -9.239641103395126009 ) ) ;
#4534=ORIENTED_EDGE ( 'NONE', *, *, #27652, .F. ) ;
#4535=CARTESIAN_POINT ( 'NONE',  ( 21.61405347744884153, -11.92327965266493983, -20.69245384154366363 ) ) ;
#4537=CARTESIAN_POINT ( 'NONE',  ( -10.79835490039502410, 17.42544872524608479, -29.34434079418894470 ) ) ;
#4539=CARTESIAN_POINT ( 'NONE',  ( -15.79675373760014523, -26.30866209883446771, -8.737002122218552103 ) ) ;
#4543=CARTESIAN_POINT ( 'NONE',  ( -33.91942916316902057, -12.79638493585070869, -9.310156918177783680 ) ) ;
#4544=CARTESIAN_POINT ( 'NONE',  ( -14.61288958351504164, -26.24343134248350040, -7.831338513189715300 ) ) ;
#4546=CARTESIAN_POINT ( 'NONE',  ( 14.31707047546269607, 16.20057490539070955, -23.09683113071953997 ) ) ;
#4547=ORIENTED_EDGE ( 'NONE', *, *, #34823, .T. ) ;
#4548=CARTESIAN_POINT ( 'NONE',  ( 22.12115478089299714, 3.764118972416656828, -20.87897183709134197 ) ) ;
#4553=CARTESIAN_POINT ( 'NONE',  ( -28.49039815446405299, -0.04531349955599923290, -12.53146938658677456 ) ) ;
#4554=CARTESIAN_POINT ( 'NONE',  ( 21.01377214067982280, 0.3319268877385900818, -26.18275839778970848 ) ) ;
#4558=CARTESIAN_POINT ( 'NONE',  ( -27.68563775692442874, 0.9759262997041426857, -12.58874013869143482 ) ) ;
#4559=CARTESIAN_POINT ( 'NONE',  ( 2.927345865710861972E-15, 22.57051819516765789, -19.69475445967420768 ) ) ;
#4572=CARTESIAN_POINT ( 'NONE',  ( 20.10367939777714597, -18.56949155725344625, -17.72620543299270679 ) ) ;
#4576=CARTESIAN_POINT ( 'NONE',  ( 12.61634089041212192, 22.15519939570359043, -17.36970231665867104 ) ) ;
#4579=CARTESIAN_POINT ( 'NONE',  ( -14.67830838625119760, 14.96923418678847462, -25.37387372424442944 ) ) ;
#4582=CARTESIAN_POINT ( 'NONE',  ( 12.93205350682161026, -23.08767904844866337, -15.45577339185666155 ) ) ;
#4585=CARTESIAN_POINT ( 'NONE',  ( 15.42600414702388001, 26.74738280129588475, -5.000000000000002665 ) ) ;
#4587=CARTESIAN_POINT ( 'NONE',  ( 12.64961623683766412, 21.05878950761225354, -18.45162358594998153 ) ) ;
#4589=CARTESIAN_POINT ( 'NONE',  ( -15.39213581000993436, 26.86843326188214576, -5.000000000000001776 ) ) ;
#4590=DIRECTION ( 'NONE',  ( -0.000000000000000000, -0.000000000000000000, -1.000000000000000000 ) ) ;
#4591=CARTESIAN_POINT ( 'NONE',  ( -9.613986047678359625, -18.34424821771797198, -27.44831228072173346 ) ) ;
#4593=VECTOR ( 'NONE', #37937, 1000.000000000000000 ) ;
#4594=CARTESIAN_POINT ( 'NONE',  ( -17.22680934732288449, -11.86017600268841576, -26.97611126009332594 ) ) ;
#4595=CARTESIAN_POINT ( 'NONE',  ( -8.692887668960288750, -24.30300274338556932, -11.76202580396936703 ) ) ;
#4596=CARTESIAN_POINT ( 'NONE',  ( 13.77818766908856496, 21.23702865708559528, -16.52942667850394898 ) ) ;
#4598=CARTESIAN_POINT ( 'NONE',  ( 22.26820236916659468, 7.937833278018120886, -14.86918834064916339 ) ) ;
#4604=CARTESIAN_POINT ( 'NONE',  ( -21.48125279631567608, -1.916317976078901753, -24.72592479754959172 ) ) ;
#4612=CARTESIAN_POINT ( 'NONE',  ( 21.43836447692151737, -10.19457909919293748, -21.85517601310809965 ) ) ;
#4616=LINE ( 'NONE', #10924, #4593 ) ;
#4620=CARTESIAN_POINT ( 'NONE',  ( -0.7148412076571604157, 36.18692081534198479, -10.17225141934236277 ) ) ;
#4627=CARTESIAN_POINT ( 'NONE',  ( 14.40481049750849785, 29.13314888007769810, -6.837637242531308779 ) ) ;
#4628=CARTESIAN_POINT ( 'NONE',  ( 35.48557158208991069, -9.180432008922032594, -4.999999999999999112 ) ) ;
#4630=CARTESIAN_POINT ( 'NONE',  ( -20.02443676921326698, 14.51187564404416719, -8.402881453741647633 ) ) ;
#4633=CARTESIAN_POINT ( 'NONE',  ( 15.11688860189568295, -26.15468757429319169, -8.766268934131305812 ) ) ;
#4635=CARTESIAN_POINT ( 'NONE',  ( 15.15954330274506923, 26.33225921297029970, -8.295889340952182778 ) ) ;
#4636=CARTESIAN_POINT ( 'NONE',  ( -13.47223693944937040, 18.09844039693852125, -21.24786896499725231 ) ) ;
#4639=CARTESIAN_POINT ( 'NONE',  ( -16.49540125530320722, -15.47634539844835011, -23.14752693098630942 ) ) ;
#4640=CARTESIAN_POINT ( 'NONE',  ( 3.412941554391075716, -22.67929815799855220, -16.95258892673083295 ) ) ;
#4641=CARTESIAN_POINT ( 'NONE',  ( 15.49509892345262330, 26.24234491965495764, -6.417516081753649182 ) ) ;
#4642=CARTESIAN_POINT ( 'NONE',  ( 21.05838016133584389, 12.97903285513515925, -6.453896350353760525 ) ) ;
#4644=ORIENTED_EDGE ( 'NONE', *, *, #35287, .T. ) ;
#4645=CARTESIAN_POINT ( 'NONE',  ( -5.935793614171071653, 34.20645656082695041, -11.10577846936933000 ) ) ;
#4656=CARTESIAN_POINT ( 'NONE',  ( -30.56378389754250335, 0.1368832906204832112, -6.888355321334826087 ) ) ;
#4659=CARTESIAN_POINT ( 'NONE',  ( 33.99017495331719374, -9.144035213149372510, -9.360703722008313576 ) ) ;
#4665=DIRECTION ( 'NONE',  ( 0.000000000000000000, 0.000000000000000000, -1.000000000000000000 ) ) ;
#4673=CARTESIAN_POINT ( 'NONE',  ( 18.55918025685463846, 17.91805357396305354, -6.442381077251955190 ) ) ;
#4674=CARTESIAN_POINT ( 'NONE',  ( 10.59284826014176240, 33.08844111058793658, -8.954051444611645039 ) ) ;
#4679=CARTESIAN_POINT ( 'NONE',  ( 16.00895768845574096, -26.86996021029318626, -5.471689731333394313 ) ) ;
#4682=DIRECTION ( 'NONE',  ( 0.000000000000000000, 0.000000000000000000, 1.000000000000000000 ) ) ;
#4685=CARTESIAN_POINT ( 'NONE',  ( -10.97587534684186927, 17.31416389292776614, -29.34816979712976348 ) ) ;
#4687=CARTESIAN_POINT ( 'NONE',  ( 14.33171430583705330, -25.57000458597046588, -10.18806973492949908 ) ) ;
#4688=CIRCLE ( 'NONE', #9873, 18.00000000000000000 ) ;
#4692=CARTESIAN_POINT ( 'NONE',  ( -11.80206329693653267, 32.84136598961480757, -7.211666007103653797 ) ) ;
#4696=CARTESIAN_POINT ( 'NONE',  ( -29.01561123397027941, -6.266648261260574060, -14.93538031197087790 ) ) ;
#4699=CARTESIAN_POINT ( 'NONE',  ( 25.14345260446027552, 0.5055508715397122321, -17.45113365086313806 ) ) ;
#4703=UNCERTAINTY_MEASURE_WITH_UNIT (LENGTH_MEASURE( 1.000000000000000082E-05 ), #37207, 'distance_accuracy_value', 'NONE');
#4705=CARTESIAN_POINT ( 'NONE',  ( -25.86155482627544444, 0.3215476971549391383, -16.44404694673128375 ) ) ;
#4709=CARTESIAN_POINT ( 'NONE',  ( 22.58427089344845129, -1.187563055018421299, -22.50445793986171950 ) ) ;
#4721=CARTESIAN_POINT ( 'NONE',  ( 2.151556361536091089, 21.31112605819426165, -25.60121844493111709 ) ) ;
#4725=CARTESIAN_POINT ( 'NONE',  ( 22.01692992093476775, -27.08823313053303750, -5.451586861850059584 ) ) ;
#4730=CARTESIAN_POINT ( 'NONE',  ( 14.97126155631352340, 26.12067504759210834, -9.230760338622234329 ) ) ;
#4732=CARTESIAN_POINT ( 'NONE',  ( -11.62347246686722357, 17.43168280077985699, -26.27056211956100285 ) ) ;
#4735=CARTESIAN_POINT ( 'NONE',  ( 15.20036834786406565, 26.19538653648924864, -8.298372456229270000 ) ) ;
#4737=CARTESIAN_POINT ( 'NONE',  ( 28.26220087632740885, -17.92022017449335536, -12.89082178051953598 ) ) ;
#4740=CARTESIAN_POINT ( 'NONE',  ( -15.15816994429180120, 27.21337269842945972, -6.875229718665281986 ) ) ;
#4742=CARTESIAN_POINT ( 'NONE',  ( -10.51723664951211923, -17.65706093263121090, -28.66670352760397833 ) ) ;
#4744=CIRCLE ( 'NONE', #13846, 15.99999999999999645 ) ;
#4746=CARTESIAN_POINT ( 'NONE',  ( -20.79469271605055880, -9.355953883521966219, -23.01360647773964629 ) ) ;
#4747=CARTESIAN_POINT ( 'NONE',  ( -9.088232624166426632, -18.50880257564897491, -28.10325226193693737 ) ) ;
#4749=CARTESIAN_POINT ( 'NONE',  ( 15.52097626904955874, 19.85846508565274959, -14.68172677917668878 ) ) ;
#4751=CARTESIAN_POINT ( 'NONE',  ( 20.09308256140095139, 4.507873197570775758, -28.22047126094187774 ) ) ;
#4756=CARTESIAN_POINT ( 'NONE',  ( -30.97995496863966380, -0.2256375777535584437, -6.412869061000700199 ) ) ;
#4757=CARTESIAN_POINT ( 'NONE',  ( 30.06298335927989740, -0.4822708793880832734, -10.14075447114801420 ) ) ;
#4761=CARTESIAN_POINT ( 'NONE',  ( -28.27971916306745470, 2.627406427308467851, -6.898641429403003400 ) ) ;
#4762=CARTESIAN_POINT ( 'NONE',  ( -19.69645987729884595, 11.37175641224114919, -21.56489709563623691 ) ) ;
#4770=ORIENTED_EDGE ( 'NONE', *, *, #15113, .T. ) ;
#4771=CARTESIAN_POINT ( 'NONE',  ( -22.69455887956607754, 5.944439957561778343, -16.84495653843570651 ) ) ;
#4774=CARTESIAN_POINT ( 'NONE',  ( 27.89879264781504276, -24.25791139881312120, -7.574806088488642786 ) ) ;
#4777=CARTESIAN_POINT ( 'NONE',  ( 12.67051716736391498, 22.07145339077409929, -17.38087975008689057 ) ) ;
#4780=CARTESIAN_POINT ( 'NONE',  ( -17.53063491166886578, 19.28413246547140503, -9.334923713665935097 ) ) ;
#4783=CARTESIAN_POINT ( 'NONE',  ( 9.439680310844765998, -18.19733056428809803, -29.34954212647691563 ) ) ;
#4785=CARTESIAN_POINT ( 'NONE',  ( 15.11232028572299946, 26.10242263575024424, -8.767989562428970984 ) ) ;
#4787=CARTESIAN_POINT ( 'NONE',  ( 15.33430753556601722, 26.63135885691745486, -6.887879096180697047 ) ) ;
#4789=CARTESIAN_POINT ( 'NONE',  ( -12.09709384379045005, 19.96450846454217043, -20.53406412358028277 ) ) ;
#4791=CARTESIAN_POINT ( 'NONE',  ( -14.96743987807556842, -25.98747055160875874, -9.238933126925131134 ) ) ;
#4793=CARTESIAN_POINT ( 'NONE',  ( -32.07387720787730956, -20.72040958422635981, -6.698075182882634593 ) ) ;
#4795=CARTESIAN_POINT ( 'NONE',  ( -4.727911438284216672, -20.01714751873747744, -28.25398441486722589 ) ) ;
#4796=CARTESIAN_POINT ( 'NONE',  ( 11.60051960103743873, 17.04428010164728136, -28.10970223773723120 ) ) ;
#4799=CARTESIAN_POINT ( 'NONE',  ( 19.95678360488982861, 7.462870846925651058, -23.27266411727370254 ) ) ;
#4805=CARTESIAN_POINT ( 'NONE',  ( -22.00238895739720490, -1.313321433655290971, -23.60997353844526359 ) ) ;
#4809=CARTESIAN_POINT ( 'NONE',  ( -24.56921341014758653, -25.93758952935236906, -7.617217473784200443 ) ) ;
#4811=CARTESIAN_POINT ( 'NONE',  ( 22.27145313233416957, -10.58722233873939444, -20.70863184773896037 ) ) ;
#4821=CARTESIAN_POINT ( 'NONE',  ( 0.2168302826061950517, 20.49890265953407109, -30.00000000000000711 ) ) ;
#4824=CARTESIAN_POINT ( 'NONE',  ( -17.34253826592568970, 27.32041144456614390, -5.000000000000000000 ) ) ;
#4827=CARTESIAN_POINT ( 'NONE',  ( 14.11763978891951687, 27.49014883721196156, -10.07373652601078007 ) ) ;
#4830=CARTESIAN_POINT ( 'NONE',  ( -18.80845520939411486, 12.28582799405812587, -18.01515471683427450 ) ) ;
#4833=CARTESIAN_POINT ( 'NONE',  ( 9.514046198846664026, -18.15855281542499000, -29.34801595497529547 ) ) ;
#4835=CARTESIAN_POINT ( 'NONE',  ( 11.86360577746352973, 19.41276117560862957, -21.61155111211224877 ) ) ;
#4836=CARTESIAN_POINT ( 'NONE',  ( -30.41237130417910706, 3.314011747244096195, -5.000000000000000000 ) ) ;
#4839=CARTESIAN_POINT ( 'NONE',  ( -21.40755417942576244, -20.13335966822008061, -15.79869096137255546 ) ) ;
#4840=CARTESIAN_POINT ( 'NONE',  ( 3.865693630706900308, -24.30145578791679029, -10.37003140332352480 ) ) ;
#4841=CARTESIAN_POINT ( 'NONE',  ( 15.46458721040396078, 26.18010667664744417, -6.888852476684097503 ) ) ;
#4842=CARTESIAN_POINT ( 'NONE',  ( 17.84088086924548122, 11.87538515410224527, -22.23966607540548068 ) ) ;
#4845=CARTESIAN_POINT ( 'NONE',  ( -6.380476842507320612, 37.12010437673579588, -5.863956392860120381 ) ) ;
#4846=ORIENTED_EDGE ( 'NONE', *, *, #8910, .T. ) ;
#4852=CARTESIAN_POINT ( 'NONE',  ( -29.79950855980051827, 0.2397400637421467640, -9.241859429830270756 ) ) ;
#4854=CARTESIAN_POINT ( 'NONE',  ( 35.47190708691255168, -11.90251233358380212, -5.000000000000003553 ) ) ;
#4858=EDGE_CURVE ( 'NONE', #19220, #2217, #4616, .T. ) ;
#4860=AXIS2_PLACEMENT_3D ( 'NONE', #23059, #19610, #26519 ) ;
#4869=CARTESIAN_POINT ( 'NONE',  ( 18.17512370925090792, 17.42502396823083899, -10.34031744549918308 ) ) ;
#4870=CARTESIAN_POINT ( 'NONE',  ( 5.926286245021443300, 20.46757980983786851, -25.76132644253925719 ) ) ;
#4875=CARTESIAN_POINT ( 'NONE',  ( 15.76324282396835486, -26.51440755082071732, -7.811281871053155967 ) ) ;
#4882=CARTESIAN_POINT ( 'NONE',  ( -12.13347509736119889, 19.92089084820641176, -20.54147204449933994 ) ) ;
#4884=CARTESIAN_POINT ( 'NONE',  ( 12.18486585843677972, -23.95081470295607318, -13.58225421544179667 ) ) ;
#4890=CARTESIAN_POINT ( 'NONE',  ( -12.29079644195909005, 31.26159447669306246, -9.015097560565573431 ) ) ;
#4895=EDGE_CURVE ( 'NONE', #5646, #860, #7001, .T. ) ;
#4896=CARTESIAN_POINT ( 'NONE',  ( -28.69299338070981875, -4.470963161381146911, -15.02617031471227627 ) ) ;
#4900=CARTESIAN_POINT ( 'NONE',  ( 29.91352946887046826, 0.1146846962358806787, -9.239818586298255809 ) ) ;
#4905=CARTESIAN_POINT ( 'NONE',  ( -23.31796685322062501, 0.5495358244031924855, -20.54176272741512221 ) ) ;
#4908=CARTESIAN_POINT ( 'NONE',  ( 32.78999465087354537, -4.002307633261452224, -9.046564716739682765 ) ) ;
#4915=LINE ( 'NONE', #11214, #13046 ) ;
#4923=CARTESIAN_POINT ( 'NONE',  ( 2.065624757052793914, 20.48161944704045823, -28.45443914133164753 ) ) ;
#4928=CARTESIAN_POINT ( 'NONE',  ( 19.11282184975060972, -26.40045450798872295, -9.072278811920540420 ) ) ;
#4931=CARTESIAN_POINT ( 'NONE',  ( 2.485571585149743523, -11.24999999999995737, 10.00000000000000000 ) ) ;
#4934=CARTESIAN_POINT ( 'NONE',  ( 15.30043618030332553, 26.74953473181076902, -6.885117079756076564 ) ) ;
#4936=CARTESIAN_POINT ( 'NONE',  ( -12.10739415485800841, 18.50350219561722653, -22.80206802353507101 ) ) ;
#4939=DIRECTION ( 'NONE',  ( 1.000000000000000000, 0.000000000000000000, 0.000000000000000000 ) ) ;
#4940=CARTESIAN_POINT ( 'NONE',  ( 11.11640272627978021, 17.47322625280633801, -27.45115658143717141 ) ) ;
#4942=CARTESIAN_POINT ( 'NONE',  ( 32.02639718292716964, -18.95205052879796526, -8.842390373194950470 ) ) ;
#4944=CARTESIAN_POINT ( 'NONE',  ( -12.13084903553365557, 20.83183464748637093, -19.44244853017589492 ) ) ;
#4946=CARTESIAN_POINT ( 'NONE',  ( -16.83103474447717574, -26.46333433132708279, -8.697577348884802717 ) ) ;
#4949=CARTESIAN_POINT ( 'NONE',  ( -18.77890958615538608, -8.456140786848550306, -28.45356751116922567 ) ) ;
#4950=CARTESIAN_POINT ( 'NONE',  ( -14.98552525403816205, -26.61491965241963342, -5.000000000000000888 ) ) ;
#4952=CARTESIAN_POINT ( 'NONE',  ( 16.61617810080481661, 21.74609680309975346, -8.817940406396488129 ) ) ;
#4954=CARTESIAN_POINT ( 'NONE',  ( 29.78831017271203763, 1.106291696078458120, -4.999999999999999112 ) ) ;
#4958=ORIENTED_EDGE ( 'NONE', *, *, #25517, .F. ) ;
#4959=CARTESIAN_POINT ( 'NONE',  ( -20.83595133204223515, 0.5720877597900050349, -26.81050348232703229 ) ) ;
#4960=CARTESIAN_POINT ( 'NONE',  ( 27.63112615685908935, -0.4701152805647206279, -14.39745280081397283 ) ) ;
#4965=CARTESIAN_POINT ( 'NONE',  ( -25.48370164714067343, 1.883020324448871463, -15.57262912828922552 ) ) ;
#4966=CARTESIAN_POINT ( 'NONE',  ( 16.84920187454417828, 29.09530251867925443, -13.79123840944734880 ) ) ;
#4969=CYLINDRICAL_SURFACE ( 'NONE', #3271, 18.00000000000002487 ) ;
#4973=CARTESIAN_POINT ( 'NONE',  ( -25.21997133566067006, 6.187216884184454813, -8.370264087233126205 ) ) ;
#4976=CARTESIAN_POINT ( 'NONE',  ( 26.14537312525837010, -25.55590668144287747, -6.734860050313713487 ) ) ;
#4979=CARTESIAN_POINT ( 'NONE',  ( 15.11844294575625014, 26.78304985304260555, -7.815403913362212407 ) ) ;
#4983=CARTESIAN_POINT ( 'NONE',  ( -16.89125701550774394, 21.69970515213497109, -7.382923725449230368 ) ) ;
#4985=CARTESIAN_POINT ( 'NONE',  ( 11.13486383234526400, -20.47745619191486099, -20.54734414695593259 ) ) ;
#4987=CARTESIAN_POINT ( 'NONE',  ( 12.94181704842254454, 21.63114967576204961, -17.44000072231445486 ) ) ;
#4989=CARTESIAN_POINT ( 'NONE',  ( 11.12160456634176953, 17.61533166272543482, -26.83009323505504184 ) ) ;
#4991=CARTESIAN_POINT ( 'NONE',  ( -11.05928181430064861, 17.65851141523520340, -26.82422181314475296 ) ) ;
#4993=CARTESIAN_POINT ( 'NONE',  ( -11.19645373508086195, -20.46641504268867351, -20.53998934932196363 ) ) ;
#4995=CARTESIAN_POINT ( 'NONE',  ( -32.24083685196362836, -20.82486095561948503, -5.856421537953417911 ) ) ;
#4996=CARTESIAN_POINT ( 'NONE',  ( -6.503947451768620880, -20.28793242900468385, -24.22034738830593881 ) ) ;
#4997=CARTESIAN_POINT ( 'NONE',  ( 15.80018706099420633, 25.22022683934922682, -6.419152679462878375 ) ) ;
#4999=CARTESIAN_POINT ( 'NONE',  ( 22.54818472930890039, 7.997166754206832096, -13.85798304266238645 ) ) ;
#5004=CARTESIAN_POINT ( 'NONE',  ( -23.24856704062857915, -1.463813097875870550, -21.34811639290027685 ) ) ;
#5020=CARTESIAN_POINT ( 'NONE',  ( 0.2168302826061956068, 20.49890265953407109, -29.21218655438333656 ) ) ;
#5027=CARTESIAN_POINT ( 'NONE',  ( 11.97830265401803729, 21.99462655053814331, -18.31500106451969856 ) ) ;
#5030=CARTESIAN_POINT ( 'NONE',  ( -19.40296131254754641, 15.36279795482867883, -9.381991658370749221 ) ) ;
#5033=CARTESIAN_POINT ( 'NONE',  ( 9.815459356401843749, -18.55056478758831062, -26.22197369305180459 ) ) ;
#5034=CARTESIAN_POINT ( 'NONE',  ( -19.48557158514985588, -11.25000000000002309, 6.000000000000000000 ) ) ;
#5035=CARTESIAN_POINT ( 'NONE',  ( 14.27839713554442902, 24.50480966180208142, -12.54774083478067226 ) ) ;
#5036=CARTESIAN_POINT ( 'NONE',  ( 15.29245034862073283, 32.56469986092002955, -4.999999999999995559 ) ) ;
#5040=CARTESIAN_POINT ( 'NONE',  ( -28.06200121101475986, -24.80525908879649322, -5.439734138379792583 ) ) ;
#5041=CARTESIAN_POINT ( 'NONE',  ( 3.177462754434345449, -21.84557965789944234, -20.09034133618861873 ) ) ;
#5042=CARTESIAN_POINT ( 'NONE',  ( 13.65169929130708759, 22.50395429108296241, -15.47332144221692296 ) ) ;
#5043=CARTESIAN_POINT ( 'NONE',  ( 20.53490407377033833, 13.94885239385593678, -6.452535063080207856 ) ) ;
#5047=CARTESIAN_POINT ( 'NONE',  ( -4.882102130403945139, 28.26406243695034348, -16.69742253351011740 ) ) ;
#5056=CARTESIAN_POINT ( 'NONE',  ( -28.01095669528613286, 0.5552823997827627256, -12.56944446269342031 ) ) ;
#5058=CARTESIAN_POINT ( 'NONE',  ( 19.98763201709199322, -6.042670552197736633, -27.05847892281659028 ) ) ;
#5076=CARTESIAN_POINT ( 'NONE',  ( 19.05816791551096401, 16.93792299125899348, -5.962097903736426119 ) ) ;
#5078=CARTESIAN_POINT ( 'NONE',  ( 9.191611640655853677, 25.94598456426656696, -16.91844301956545138 ) ) ;
#5082=CARTESIAN_POINT ( 'NONE',  ( 9.998379901438696038, -18.29407794464048109, -26.80397355526891801 ) ) ;
#5083=DIRECTION ( 'NONE',  ( -0.000000000000000000, 0.000000000000000000, -1.000000000000000000 ) ) ;
#5084=CARTESIAN_POINT ( 'NONE',  ( 35.84808252048253507, -3.038699442442316379, -13.99876745781542553 ) ) ;
#5085=CARTESIAN_POINT ( 'NONE',  ( -15.41023552481722447, 26.80405844223972522, -5.000000000000001776 ) ) ;
#5087=CARTESIAN_POINT ( 'NONE',  ( 14.07774217773769898, -26.11933264415325340, -7.834443513061088105 ) ) ;
#5093=CARTESIAN_POINT ( 'NONE',  ( -11.80160148247466978, 29.89982266266324729, -11.28701977302258541 ) ) ;
#5097=CARTESIAN_POINT ( 'NONE',  ( -26.13677174093514566, -4.840508227981996647, -17.91196310124766455 ) ) ;
#5098=CARTESIAN_POINT ( 'NONE',  ( 18.00000000000002487, 22.50000000000001421, 3.000000000000000000 ) ) ;
#5100=CARTESIAN_POINT ( 'NONE',  ( 22.20747034583386892, 0.7192958970858360779, -22.74178951375157354 ) ) ;
#5106=CARTESIAN_POINT ( 'NONE',  ( -20.48192033757745278, 0.8608427067432721236, -29.34839852770058499 ) ) ;
#5109=CARTESIAN_POINT ( 'NONE',  ( 21.05756235747694305, -2.325109266878002678, -25.95433224628644098 ) ) ;
#5110=CIRCLE ( 'NONE', #10946, 18.00000000000000000 ) ;
#5121=CARTESIAN_POINT ( 'NONE',  ( 19.48557158514982746, -11.25000000000009415, 0.000000000000000000 ) ) ;
#5122=AXIS2_PLACEMENT_3D ( 'NONE', #3034, #22118, #19265 ) ;
#5123=CARTESIAN_POINT ( 'NONE',  ( 3.938319053363494859, 24.20383553360720796, -20.77087860374098938 ) ) ;
#5127=CARTESIAN_POINT ( 'NONE',  ( 19.65700424793906009, -25.74060475042004015, -10.40124817034949167 ) ) ;
#5133=CARTESIAN_POINT ( 'NONE',  ( 12.33829340598856916, 20.56101506373660470, -19.48517987220360226 ) ) ;
#5135=CARTESIAN_POINT ( 'NONE',  ( -13.45522894562555116, 21.80059734131468474, -16.48174157838437281 ) ) ;
#5138=CARTESIAN_POINT ( 'NONE',  ( 14.59096746045820581, 24.81100808824554704, -11.60372034950707842 ) ) ;
#5140=CARTESIAN_POINT ( 'NONE',  ( 31.64230937557188739, -20.05769974086166130, -8.405444945822866387 ) ) ;
#5142=CARTESIAN_POINT ( 'NONE',  ( -10.67558526762242188, 17.55646416338892735, -28.69320066300005934 ) ) ;
#5144=CARTESIAN_POINT ( 'NONE',  ( -18.17112659014724230, -26.98930163720866560, -7.288977103906384869 ) ) ;
#5148=CARTESIAN_POINT ( 'NONE',  ( -22.09523395385413380, -8.380097828030171669, -21.91654685885929155 ) ) ;
#5149=CARTESIAN_POINT ( 'NONE',  ( -14.83609535436326432, -26.57805634534657102, -5.000000000000000888 ) ) ;
#5152=CARTESIAN_POINT ( 'NONE',  ( 28.80506163160762512, 1.156882464205359007, -9.731288915196888212 ) ) ;
#5156=CARTESIAN_POINT ( 'NONE',  ( -22.24152314221094784, 0.5810505375398892225, -22.72432294289647103 ) ) ;
#5157=CARTESIAN_POINT ( 'NONE',  ( 24.27527364323341175, -0.3479384314849937043, -19.38528656166962705 ) ) ;
#5161=CARTESIAN_POINT ( 'NONE',  ( -21.85307150740203141, 2.101201123924372194, -22.89954997427944505 ) ) ;
#5163=CARTESIAN_POINT ( 'NONE',  ( -9.163310636333559245, 20.63632441393290762, -20.55760979252981357 ) ) ;
#5173=CARTESIAN_POINT ( 'NONE',  ( -20.62745669879552324, 5.024763284673062991, -24.24502725807042580 ) ) ;
#5176=CARTESIAN_POINT ( 'NONE',  ( 14.64330500336448004, -14.34584279044560162, -29.24371549410482274 ) ) ;
#5179=CARTESIAN_POINT ( 'NONE',  ( 10.63104621300768216, 17.52826713075782905, -29.34073607691351526 ) ) ;
#5183=CARTESIAN_POINT ( 'NONE',  ( -16.44336537299682988, 20.94030426362907704, -10.75757732011587109 ) ) ;
#5186=CARTESIAN_POINT ( 'NONE',  ( 15.10958474974925636, 26.11133633985198443, -8.767902982274385693 ) ) ;
#5190=ORIENTED_EDGE ( 'NONE', *, *, #8305, .T. ) ;
#5191=CARTESIAN_POINT ( 'NONE',  ( -10.92267213224567968, 17.34778819946280493, -29.34702194411721266 ) ) ;
#5194=CARTESIAN_POINT ( 'NONE',  ( -15.25928708397310096, -26.30311034880537235, -8.294554573284210974 ) ) ;
#5197=CARTESIAN_POINT ( 'NONE',  ( -17.86905274512871244, -10.06606982860865784, -29.21172267095328223 ) ) ;
#5198=CARTESIAN_POINT ( 'NONE',  ( -5.097925932147637340, -20.80854798773387770, -23.20461931772074138 ) ) ;
#5200=CARTESIAN_POINT ( 'NONE',  ( 15.82933155468543518, 25.27777941642500537, -5.946733502468819488 ) ) ;
#5202=CARTESIAN_POINT ( 'NONE',  ( 24.82669879306046212, 6.427578836846941535, -9.348943503324091964 ) ) ;
#5207=CARTESIAN_POINT ( 'NONE',  ( -30.07554202086022954, -1.447249947434508854, -11.47170067724066733 ) ) ;
#5208=CARTESIAN_POINT ( 'NONE',  ( 28.46466429971498968, -0.01335223302803286403, -12.53469640236253824 ) ) ;
#5216=ORIENTED_EDGE ( 'NONE', *, *, #39843, .T. ) ;
#5221=CARTESIAN_POINT ( 'NONE',  ( 0.3120762500772759629, 29.08244079073152477, -16.62608502115921993 ) ) ;
#5222=CARTESIAN_POINT ( 'NONE',  ( -16.00000000000000000, 22.50000000000000355, 10.00000000000000000 ) ) ;
#5228=CARTESIAN_POINT ( 'NONE',  ( 14.88818521422670571, 28.28006465736570618, -5.930970288686092218 ) ) ;
#5232=CARTESIAN_POINT ( 'NONE',  ( -18.87212912419562016, 14.83998797668345659, -12.86572329467758458 ) ) ;
#5236=CARTESIAN_POINT ( 'NONE',  ( 15.52090202525632279, -26.75102145164868972, -5.000000000000000888 ) ) ;
#5239=CARTESIAN_POINT ( 'NONE',  ( 15.32791351282358505, 26.65397767157460507, -6.887199522823470588 ) ) ;
#5242=CARTESIAN_POINT ( 'NONE',  ( -16.07603441159168867, -13.35307911771159972, -27.01628995842852987 ) ) ;
#5243=CARTESIAN_POINT ( 'NONE',  ( 1.676194954344619292, -23.72096887343614924, -12.89182188841930454 ) ) ;
#5244=CARTESIAN_POINT ( 'NONE',  ( 12.29335586182468631, 19.73195647831804678, -20.56948206563339454 ) ) ;
#5245=CARTESIAN_POINT ( 'NONE',  ( 17.63004972000715753, 10.74884895982777522, -27.17813552644222241 ) ) ;
#5249=CARTESIAN_POINT ( 'NONE',  ( -4.870223975577004261, 20.79813088136934240, -25.69976142956964438 ) ) ;
#5256=CARTESIAN_POINT ( 'NONE',  ( -28.17636587710437368, 0.3453695044007577541, -12.55976439041781312 ) ) ;
#5258=CARTESIAN_POINT ( 'NONE',  ( 30.05582894924074111, -10.02326609248156331, -13.87827096244793879 ) ) ;
#5260=CIRCLE ( 'NONE', #10451, 18.00000000000000000 ) ;
#5273=CARTESIAN_POINT ( 'NONE',  ( 18.50304859244888789, 17.84556192672934927, -7.408648105292232167 ) ) ;
#5274=CARTESIAN_POINT ( 'NONE',  ( 7.149399299886240122, 20.02420714680316394, -25.84280504995552619 ) ) ;
#5276=CARTESIAN_POINT ( 'NONE',  ( -18.35172899305704064, 9.167379654309337766, -29.99999999999999645 ) ) ;
#5279=CARTESIAN_POINT ( 'NONE',  ( 15.58925272520251148, -26.26116752309117786, -8.745968726765523726 ) ) ;
#5281=CARTESIAN_POINT ( 'NONE',  ( 17.34253826539385201, 27.32041144647958575, -5.000000000000000000 ) ) ;
#5282=CARTESIAN_POINT ( 'NONE',  ( -13.20200830158507443, 22.24945722037973184, -16.44235390662751328 ) ) ;
#5285=CARTESIAN_POINT ( 'NONE',  ( 13.83190959151879618, -25.74325333655491121, -9.252723044361745863 ) ) ;
#5291=CARTESIAN_POINT ( 'NONE',  ( -12.43868061211408005, 31.69022611209930318, -8.118098891794449656 ) ) ;
#5297=CARTESIAN_POINT ( 'NONE',  ( 20.47975215921984216, 0.9111364859620189049, -29.34931494995705847 ) ) ;
#5304=CARTESIAN_POINT ( 'NONE',  ( -29.78514619038734068, 0.06227709271290194498, -9.709532440474664128 ) ) ;
#5307=CARTESIAN_POINT ( 'NONE',  ( 33.96295552133759088, -5.157459216464866714, -7.229003133675814929 ) ) ;
#5320=CARTESIAN_POINT ( 'NONE',  ( 3.344107530154690977, 20.63130717731051789, -27.01118353652808679 ) ) ;
#5324=CARTESIAN_POINT ( 'NONE',  ( 18.80843487349309839, -26.01514764349690978, -9.984653526650497213 ) ) ;
#5327=CARTESIAN_POINT ( 'NONE',  ( 37.57549957648898697, 32.94422479542058824, 3.000000000000000000 ) ) ;
#5329=CARTESIAN_POINT ( 'NONE',  ( 15.06417566331624336, 26.26151533851359332, -8.762166468963160426 ) ) ;
#5331=CARTESIAN_POINT ( 'NONE',  ( -15.46686712649010254, 26.33727822508064875, -6.417365845589783291 ) ) ;
#5334=CARTESIAN_POINT ( 'NONE',  ( 20.23296131041715640, 28.12381335138032412, 3.000000000000000000 ) ) ;
#5335=CARTESIAN_POINT ( 'NONE',  ( 11.20885904078801687, 17.55440590958596658, -26.83820411716370913 ) ) ;
#5337=CARTESIAN_POINT ( 'NONE',  ( 18.45928777744525817, -10.91947781374027926, -25.57488933213381088 ) ) ;
#5338=ORIENTED_EDGE ( 'NONE', *, *, #20021, .T. ) ;
#5339=CARTESIAN_POINT ( 'NONE',  ( -11.32776516902169206, 19.24857545329237496, -22.67347498135675821 ) ) ;
#5341=CARTESIAN_POINT ( 'NONE',  ( -17.74186490489988444, -26.41810987378744002, -9.118522922409818321 ) ) ;
#5345=CARTESIAN_POINT ( 'NONE',  ( -24.05107439686812398, -8.291669621499529796, -19.73756104527254962 ) ) ;
#5346=CARTESIAN_POINT ( 'NONE',  ( -9.780434648196228764, -18.88852710088067610, -25.03561068106941079 ) ) ;
#5350=CARTESIAN_POINT ( 'NONE',  ( 27.98159544772139995, 1.197522363590045602, -11.63887822456392840 ) ) ;
#5354=CARTESIAN_POINT ( 'NONE',  ( -29.44376907024975765, -0.02629414463411203565, -10.64560707404265116 ) ) ;
#5356=CARTESIAN_POINT ( 'NONE',  ( 22.91868624822824074, -0.04345034985262812705, -21.52910780376702249 ) ) ;
#5360=CARTESIAN_POINT ( 'NONE',  ( -27.46442853353828184, 3.518614321624921715, -7.380921586237230159 ) ) ;
#5365=EDGE_CURVE ( 'NONE', #31289, #39512, #6515, .T. ) ;
#5370=CARTESIAN_POINT ( 'NONE',  ( -25.46978366468587041, 6.210661816339332120, -6.438542239147753143 ) ) ;
#5373=CARTESIAN_POINT ( 'NONE',  ( 20.09942049894790728, -20.92583357156711799, -15.85785305014610458 ) ) ;
#5376=CARTESIAN_POINT ( 'NONE',  ( 10.96925589186059113, 18.29886720915252241, -24.96787355622415561 ) ) ;
#5380=CARTESIAN_POINT ( 'NONE',  ( -14.49113235944208355, 19.17988935812739371, -17.67406450707707322 ) ) ;
#5384=CARTESIAN_POINT ( 'NONE',  ( 11.32792303687276991, 18.02407018003295747, -25.01698112430106846 ) ) ;
#5388=CARTESIAN_POINT ( 'NONE',  ( -10.97556112068393652, 17.46725186558634846, -28.07356528432091025 ) ) ;
#5390=CARTESIAN_POINT ( 'NONE',  ( -15.33514102452888039, -26.41503892009194132, -7.825054394630688748 ) ) ;
#5394=CARTESIAN_POINT ( 'NONE',  ( -29.61831833031994066, -15.50338790811805545, -12.89226513978680444 ) ) ;
#5395=CARTESIAN_POINT ( 'NONE',  ( -9.262515494080826528, -25.37554028901857350, -6.432242585004741109 ) ) ;
#5397=CARTESIAN_POINT ( 'NONE',  ( 12.48130235025789503, 18.13369772704632865, -22.85847515466027247 ) ) ;
#5400=CARTESIAN_POINT ( 'NONE',  ( 25.26210396730482444, 6.474115558529597081, -6.439678367293860894 ) ) ;
#5405=CARTESIAN_POINT ( 'NONE',  ( -31.59685791085809115, -0.8232729786593077081, -5.935614622407810792 ) ) ;
#5407=CARTESIAN_POINT ( 'NONE',  ( 22.23423511320995161, 0.6107731265070599491, -22.72817852523589011 ) ) ;
#5411=CARTESIAN_POINT ( 'NONE',  ( 19.69645987729881043, 11.37175641224107814, -29.99999999999998579 ) ) ;
#5414=STYLED_ITEM ( 'NONE', ( #13404 ), #23086 ) ;
#5419=B_SPLINE_CURVE_WITH_KNOTS ( 'NONE', 3,
 ( #403, #26335, #22673, #4394, #23488, #20451, #35077, #22874, #28222, #7231, #20249, #1352, #28977, #25923, #38322, #16799, #13736, #26126, #38522, #35483 ),
 .UNSPECIFIED., .F., .F.,
 ( 4, 2, 1, 1, 1, 1, 1, 1, 2, 2, 2, 2, 4 ),
 ( 0.000000000000000000, 0.0009765625000000845678, 0.001953125000000169136, 0.003906250000000261943, 0.007812500000000300107, 0.01562500000000022551, 0.03125000000000022898, 0.06250000000000023592, 0.1250000000000001388, 0.2500000000000001665, 0.5000000000000001110, 0.7500000000000001110, 1.000000000000000000 ),
 .UNSPECIFIED. ) ;
#5424=CARTESIAN_POINT ( 'NONE',  ( 0.2421583011816821618, 22.82788874588058547, -22.98502890671374033 ) ) ;
#5431=CARTESIAN_POINT ( 'NONE',  ( 13.25098614097699823, 25.59540253443141822, -13.36463472324928858 ) ) ;
#5434=CARTESIAN_POINT ( 'NONE',  ( -19.07024319634674825, 16.49937253695148343, -7.903667226272353297 ) ) ;
#5438=CARTESIAN_POINT ( 'NONE',  ( 13.04810291801232047, -23.09410372734021877, -15.44714336548847911 ) ) ;
#5440=CARTESIAN_POINT ( 'NONE',  ( 10.95987886464238059, 17.32429135621979555, -29.34782466777161858 ) ) ;
#5445=CARTESIAN_POINT ( 'NONE',  ( -19.34051520155174941, -15.12089003882966054, -20.75336540952627118 ) ) ;
#5446=CARTESIAN_POINT ( 'NONE',  ( 5.013169528391580698, -22.01313204235280452, -18.95530368308426716 ) ) ;
#5447=CARTESIAN_POINT ( 'NONE',  ( 11.12785985892924678, 17.21691741209329862, -29.35143107680136865 ) ) ;
#5449=CARTESIAN_POINT ( 'NONE',  ( 21.64434010710703404, 12.04703973602239842, -5.483094818529050229 ) ) ;
#5451=CARTESIAN_POINT ( 'NONE',  ( -6.164342072519281679, 35.60899897206203235, -9.314755791877534108 ) ) ;
#5457=CARTESIAN_POINT ( 'NONE',  ( -30.58060419123731677, 0.1872796535314501520, -6.417327285377274926 ) ) ;
#5458=CARTESIAN_POINT ( 'NONE',  ( 34.93334028802587454, -11.69476465809384358, -7.578579032868311138 ) ) ;
#5470=CARTESIAN_POINT ( 'NONE',  ( 20.04635827611367205, 14.95022894506133859, -5.482161707068185841 ) ) ;
#5471=CARTESIAN_POINT ( 'NONE',  ( 12.41906572600498926, 32.58765353250298347, -5.451709377992093764 ) ) ;
#5473=CARTESIAN_POINT ( 'NONE',  ( -22.38085876145960640, 10.82216326969894737, -5.000000000000000000 ) ) ;
#5476=CARTESIAN_POINT ( 'NONE',  ( 9.791560039807741589, -18.01123673837627592, -30.00000000000000000 ) ) ;
#5478=CARTESIAN_POINT ( 'NONE',  ( 22.45323650136968396, -2.382502413133517738, -20.55760979252983134 ) ) ;
#5479=CARTESIAN_POINT ( 'NONE',  ( -12.39277014389930720, 20.48808981389291972, -19.49672617547258113 ) ) ;
#5480=CARTESIAN_POINT ( 'NONE',  ( -13.95730328712268253, -15.73161065168129191, -26.46684035671119872 ) ) ;
#5481=CARTESIAN_POINT ( 'NONE',  ( 9.465041007626510350, -19.87709408547213030, -22.85921428194744109 ) ) ;
#5486=CARTESIAN_POINT ( 'NONE',  ( -8.292854476136895414, 20.68584148307280657, -23.41493881702373869 ) ) ;
#5491=CARTESIAN_POINT ( 'NONE',  ( 25.18250945046685985, 0.4325523370485113706, -17.44396110470962213 ) ) ;
#5496=CARTESIAN_POINT ( 'NONE',  ( -30.17422560392139630, 0.02279020665480178606, -8.767816438049354844 ) ) ;
#5499=CARTESIAN_POINT ( 'NONE',  ( 20.36542025373884002, -2.868257021092958325, -28.57874933910315107 ) ) ;
#5513=CARTESIAN_POINT ( 'NONE',  ( 3.643761437349164023, 22.44536600252848402, -23.06246887300423154 ) ) ;
#5518=CARTESIAN_POINT ( 'NONE',  ( 18.39798444451995607, -26.88534991441762756, -7.737902397617890671 ) ) ;
#5524=CARTESIAN_POINT ( 'NONE',  ( 12.09121274333381990, 19.97150667970398530, -20.53287558875649665 ) ) ;
#5527=CARTESIAN_POINT ( 'NONE',  ( -11.97496251553392277, 18.63315434291826378, -22.78159754204189724 ) ) ;
#5531=CARTESIAN_POINT ( 'NONE',  ( 11.09322631748854526, 17.29180187222242893, -28.71057073618882782 ) ) ;
#5533=CARTESIAN_POINT ( 'NONE',  ( 26.99793250668803779, -15.97657516354929896, -14.72900161456918156 ) ) ;
#5535=CARTESIAN_POINT ( 'NONE',  ( -10.99303974619111379, 18.28104912796820258, -24.97110850915958835 ) ) ;
#5537=CARTESIAN_POINT ( 'NONE',  ( -17.22232769333860958, -27.00279332920328201, -6.390812999317612153 ) ) ;
#5540=CARTESIAN_POINT ( 'NONE',  ( -22.93034800799257766, -8.692403048024743839, -20.77076282677819208 ) ) ;
#5541=CARTESIAN_POINT ( 'NONE',  ( -9.270452999807254457, -18.33270093331148232, -28.71663414965336614 ) ) ;
#5544=CARTESIAN_POINT ( 'NONE',  ( 20.26233914688108229, 3.111977874782128506, -29.38369824820663467 ) ) ;
#5550=CARTESIAN_POINT ( 'NONE',  ( -20.82302739279173664, 0.7399220483990450736, -26.82356524530285569 ) ) ;
#5552=CARTESIAN_POINT ( 'NONE',  ( 31.66461267357289344, -1.371321637605815491, -7.774225005612001027 ) ) ;
#5555=CARTESIAN_POINT ( 'NONE',  ( -20.30511407948876013, 2.906241227738919353, -29.38143097496937273 ) ) ;
#5567=CARTESIAN_POINT ( 'NONE',  ( -25.37084529744385364, 6.201493023855051412, -7.401802512559587655 ) ) ;
#5570=CARTESIAN_POINT ( 'NONE',  ( 24.58474773790242551, -25.53886705254056366, -8.487929553482985057 ) ) ;
#5572=CARTESIAN_POINT ( 'NONE',  ( 14.36733273649021037, 25.42688099805458535, -11.56502463518844870 ) ) ;
#5575=CARTESIAN_POINT ( 'NONE',  ( -16.67043351861327949, 21.32468196532498794, -9.304548275486963504 ) ) ;
#5578=CARTESIAN_POINT ( 'NONE',  ( 15.11505727992676817, 26.09351122695967717, -8.768076250299181140 ) ) ;
#5580=CARTESIAN_POINT ( 'NONE',  ( 11.00500201062596517, 17.34882336543230252, -28.70691125584463421 ) ) ;
#5583=CARTESIAN_POINT ( 'NONE',  ( -15.27621298814653805, 26.83222824197973111, -6.883326331195013026 ) ) ;
#5585=CARTESIAN_POINT ( 'NONE',  ( -12.66759234962441205, -22.55799813172369284, -16.44235456654224592 ) ) ;
#5589=CARTESIAN_POINT ( 'NONE',  ( -33.45162411266466762, -18.83634436166192572, -6.275798148608882521 ) ) ;
#5590=CARTESIAN_POINT ( 'NONE',  ( -7.472041749460323068, -19.13836991950213928, -30.00000000000000000 ) ) ;
#5591=CARTESIAN_POINT ( 'NONE',  ( 19.48557158514982746, -11.25000000000009415, 0.000000000000000000 ) ) ;
#5592=CARTESIAN_POINT ( 'NONE',  ( 13.37849741503627321, 20.00359433874854886, -18.57205045318708514 ) ) ;
#5594=CARTESIAN_POINT ( 'NONE',  ( 19.15330224686634963, 7.305649259636135540, -29.42185863855868178 ) ) ;
#5602=CARTESIAN_POINT ( 'NONE',  ( -31.20810765349570559, -1.166897260341405396, -8.705153276337458834 ) ) ;
#5603=CARTESIAN_POINT ( 'NONE',  ( 23.33830534371964660, 0.4941299462022573086, -20.53406551574947159 ) ) ;
#5606=CARTESIAN_POINT ( 'NONE',  ( 18.07620401364302865, 24.68088026512193522, -5.000000000000000000 ) ) ;
#5612=DIRECTION ( 'NONE',  ( -0.000000000000000000, 0.000000000000000000, -1.000000000000000000 ) ) ;
#5613=CARTESIAN_POINT ( 'NONE',  ( 1.522946860592270912, 36.84862743726508683, -9.282692509776795831 ) ) ;
#5622=CARTESIAN_POINT ( 'NONE',  ( 14.70740557672079518, 28.82247346305062408, -4.999999999999998224 ) ) ;
#5625=CARTESIAN_POINT ( 'NONE',  ( -15.95094248367131051, 12.99020724966809226, -28.27984824884035220 ) ) ;
#5628=CARTESIAN_POINT ( 'NONE',  ( 14.62380663947432424, -25.46090403646468658, -10.65324618990382000 ) ) ;
#5629=CARTESIAN_POINT ( 'NONE',  ( 13.20924685295715939, 22.23599012058760138, -16.44404666642637380 ) ) ;
#5630=CARTESIAN_POINT ( 'NONE',  ( 11.28552181379516917, 18.05715790883359162, -25.01120835586647217 ) ) ;
#5632=CARTESIAN_POINT ( 'NONE',  ( -25.71436706254305449, 9.015208126564347779, -5.000000000000000000 ) ) ;
#5634=CARTESIAN_POINT ( 'NONE',  ( -21.80912045058639137, -17.07601322584738668, -17.64863767831755226 ) ) ;
#5635=CARTESIAN_POINT ( 'NONE',  ( -0.3892639042814902139, -24.76257045605676765, -5.967383921424669779 ) ) ;
#5636=CARTESIAN_POINT ( 'NONE',  ( 14.28419796674242903, 23.34865556538064624, -13.54193682566124224 ) ) ;
#5637=CARTESIAN_POINT ( 'NONE',  ( 21.09080728949390959, 11.74853788546874611, -10.88613492565143659 ) ) ;
#5639=CARTESIAN_POINT ( 'NONE',  ( -5.048995700102136830, 35.35551730485902766, -10.19541838177800308 ) ) ;
#5646=VERTEX_POINT ( 'NONE', #12014 ) ;
#5649=CARTESIAN_POINT ( 'NONE',  ( -29.60162710802623565, 0.4573586862140032183, -9.245429160158396442 ) ) ;
#5650=CARTESIAN_POINT ( 'NONE',  ( 35.51876124919839839, -10.74978321004375559, -5.441203547717361033 ) ) ;
#5665=CARTESIAN_POINT ( 'NONE',  ( 28.80350438480166630, -23.56000536320865990, -7.566454254401802082 ) ) ;
#5666=CARTESIAN_POINT ( 'NONE',  ( 19.54635772746084399, 15.94078878846792335, -5.000000000000000888 ) ) ;
#5668=CARTESIAN_POINT ( 'NONE',  ( 11.32514681141933544, 29.41259196502597462, -12.20161796427938405 ) ) ;
#5672=CARTESIAN_POINT ( 'NONE',  ( -19.01626305010417539, 9.437311419952862934, -23.32612332779064701 ) ) ;
#5675=CARTESIAN_POINT ( 'NONE',  ( 11.68354902705863019, -20.96014224807484538, -19.47927830206757704 ) ) ;
#5678=CARTESIAN_POINT ( 'NONE',  ( 19.69645987729881043, 11.37175641224107814, -29.99999999999998579 ) ) ;
#5680=CARTESIAN_POINT ( 'NONE',  ( -11.45389309739204897, 18.46357293444315317, -23.84913706035775149 ) ) ;
#5681=CARTESIAN_POINT ( 'NONE',  ( -24.27663368075341310, -25.65399678531768757, -8.493885956241761903 ) ) ;
#5682=CARTESIAN_POINT ( 'NONE',  ( 12.06583107040341929, -23.04759528289364923, -15.51202566005124162 ) ) ;
#5686=CARTESIAN_POINT ( 'NONE',  ( -10.75718172855884802, 32.61644780836525115, -9.406819691704866315 ) ) ;
#5693=CARTESIAN_POINT ( 'NONE',  ( 29.53845057008524577, 0.1145761312098864948, -10.18194101559443077 ) ) ;
#5698=CARTESIAN_POINT ( 'NONE',  ( -20.52651921773533417, 0.8666805026383144206, -28.70727906677954877 ) ) ;
#5701=CARTESIAN_POINT ( 'NONE',  ( 20.38971234282849565, -2.225416161360934897, -29.99999999999998579 ) ) ;
#5702=CIRCLE ( 'NONE', #15417, 21.00000000000002842 ) ;
#5705=ORIENTED_EDGE ( 'NONE', *, *, #17970, .T. ) ;
#5709=PLANE ( 'NONE',  #18260 ) ;
#5717=CARTESIAN_POINT ( 'NONE',  ( 4.160566904805777178, 21.52518878017418658, -24.32380698736195512 ) ) ;
#5720=CARTESIAN_POINT ( 'NONE',  ( 19.48118952213373234, -26.85980758568562266, -7.713377719299291613 ) ) ;
#5721=FILL_AREA_STYLE_COLOUR ( '', #25548 ) ;
#5725=CARTESIAN_POINT ( 'NONE',  ( 11.43919839650344450, 18.47623239142585660, -23.84679931570577338 ) ) ;
#5728=CARTESIAN_POINT ( 'NONE',  ( -15.40861458322169852, 26.71707234346735049, -5.946083594750080081 ) ) ;
#5731=CARTESIAN_POINT ( 'NONE',  ( 15.27508919949933386, -26.56523461522311180, -6.888122384594280945 ) ) ;
#5733=CARTESIAN_POINT ( 'NONE',  ( 14.35017349371148221, 24.32190247689503337, -12.55613400241091959 ) ) ;
#5735=CARTESIAN_POINT ( 'NONE',  ( 31.27850618055397192, -21.17625281506686719, -7.548661271228884750 ) ) ;
#5738=CARTESIAN_POINT ( 'NONE',  ( -10.65603027360134902, 17.51308114404589844, -29.34127381359134290 ) ) ;
#5740=CARTESIAN_POINT ( 'NONE',  ( -14.89315407779151101, -22.48991538682484048, -16.21632406099578105 ) ) ;
#5741=CARTESIAN_POINT ( 'NONE',  ( -11.31392148919591811, 36.91540483778867099, -5.000000000000009770 ) ) ;
#5744=CARTESIAN_POINT ( 'NONE',  ( -35.26882099528151571, -12.14860974803371008, -6.718074511898288748 ) ) ;
#5745=CARTESIAN_POINT ( 'NONE',  ( -9.602157984762992982, -18.64544031278391856, -26.24206618660978307 ) ) ;
#5748=CARTESIAN_POINT ( 'NONE',  ( 29.69046389894461413, 1.111644899601798020, -6.418887305067702442 ) ) ;
#5753=CARTESIAN_POINT ( 'NONE',  ( -30.55268131219984795, -0.08272631737051794332, -7.824640561139657891 ) ) ;
#5755=CARTESIAN_POINT ( 'NONE',  ( 26.35789183837046323, -0.5391633472264854010, -16.33873335832168294 ) ) ;
#5758=CARTESIAN_POINT ( 'NONE',  ( -27.36767439016168169, 3.518543689082064496, -7.859504197288676330 ) ) ;
#5765=AXIS2_PLACEMENT_3D ( 'NONE', #2522, #14912, #33609 ) ;
#5771=CARTESIAN_POINT ( 'NONE',  ( -22.98333746671406175, 7.800124279482834488, -12.84308237461532087 ) ) ;
#5775=CARTESIAN_POINT ( 'NONE',  ( 25.76273642380879991, -25.21432076522168941, -8.033030049480178292 ) ) ;
#5777=CARTESIAN_POINT ( 'NONE',  ( 14.92263478618264294, 26.27297000776338365, -9.223291497026121277 ) ) ;
#5780=CARTESIAN_POINT ( 'NONE',  ( -15.86769938419567083, 19.96447385803967123, -13.70337137721306497 ) ) ;
#5783=CARTESIAN_POINT ( 'NONE',  ( 15.03495856122551189, 25.91540030226262914, -9.238980687715695694 ) ) ;
#5787=CARTESIAN_POINT ( 'NONE',  ( -11.61453560076544633, 18.98021450145642675, -22.72268002348484117 ) ) ;
#5788=CARTESIAN_POINT ( 'NONE',  ( 0.000000000000000000, 22.50000000000000355, 6.000000000000000000 ) ) ;
#5789=CARTESIAN_POINT ( 'NONE',  ( -14.70220195220311687, -25.47735308124121900, -10.64826642331331463 ) ) ;
#5793=CARTESIAN_POINT ( 'NONE',  ( -33.36586913699030532, -18.78766072402438780, -6.696109138991947596 ) ) ;
#5794=CARTESIAN_POINT ( 'NONE',  ( -13.49893695621550016, -25.67936680625057377, -9.257259980528091958 ) ) ;
#5796=CARTESIAN_POINT ( 'NONE',  ( 16.29902410653496148, 23.87181549541910641, -5.474405017214732716 ) ) ;
#5798=CARTESIAN_POINT ( 'NONE',  ( 24.44976066607466336, 7.357379235516989802, -7.896790638060003253 ) ) ;
#5805=CARTESIAN_POINT ( 'NONE',  ( -29.80098406382914078, -1.038879420582270008, -11.50085024836739400 ) ) ;
#5806=CARTESIAN_POINT ( 'NONE',  ( 23.99938430216166552, 0.3490643838479008942, -19.47749761754171516 ) ) ;
#5818=CARTESIAN_POINT ( 'NONE',  ( 1.749742296866609426, 24.60707399529504613, -20.70440855371920819 ) ) ;
#5828=CARTESIAN_POINT ( 'NONE',  ( 10.29438980144439419, 17.78647955463217301, -28.67741383145057199 ) ) ;
#5831=CARTESIAN_POINT ( 'NONE',  ( -18.73768915581330674, 17.66930787322032259, -4.999999999999999112 ) ) ;
#5834=CARTESIAN_POINT ( 'NONE',  ( 15.32796092042050340, -26.50622118238649350, -7.357831815769672268 ) ) ;
#5835=CARTESIAN_POINT ( 'NONE',  ( -22.76616367233569349, -26.90916104157130917, -5.891115712074672217 ) ) ;
#5837=CARTESIAN_POINT ( 'NONE',  ( 14.92356852104117770, 25.83598546049896783, -9.706920252742902377 ) ) ;
#5839=CARTESIAN_POINT ( 'NONE',  ( 9.163310636333564574, 20.63632441393291117, -29.99999999999999645 ) ) ;
#5841=CARTESIAN_POINT ( 'NONE',  ( -16.34560159223972065, -12.76520082579527404, -27.73245455758713618 ) ) ;
#5842=CARTESIAN_POINT ( 'NONE',  ( 1.248574341839781221, -20.60364275570908532, -27.73818904947963304 ) ) ;
#5843=CARTESIAN_POINT ( 'NONE',  ( 11.40065244407918144, 17.41857868398212972, -26.85574052250835919 ) ) ;
#5844=CARTESIAN_POINT ( 'NONE',  ( 22.17839790455657933, 11.08535783459926094, -6.452902206156526432 ) ) ;
#5846=CARTESIAN_POINT ( 'NONE',  ( -3.429749143149385837, 24.32645949754238046, -20.75053988368563651 ) ) ;
#5848=CARTESIAN_POINT ( 'NONE',  ( -34.46511719672074747, -5.518907050001597092, -5.000000000000002665 ) ) ;
#5855=CARTESIAN_POINT ( 'NONE',  ( -26.72518533667481577, 0.8341530811610744500, -14.51637089005181203 ) ) ;
#5856=CARTESIAN_POINT ( 'NONE',  ( 31.62610052856013709, -12.69311474474635482, -12.00053912072756646 ) ) ;
#5865=CARTESIAN_POINT ( 'NONE',  ( -1.676223514573964568, 21.07032463922739751, -26.26967824088364267 ) ) ;
#5870=CARTESIAN_POINT ( 'NONE',  ( 29.22772011238637901, -23.88113300063707811, -5.863119439596483851 ) ) ;
#5872=CARTESIAN_POINT ( 'NONE',  ( 19.51189016592634218, 15.90513825914224100, -6.448676663417378663 ) ) ;
#5873=CARTESIAN_POINT ( 'NONE',  ( 11.78623425354685850, 30.69510100094851168, -10.36589696378858072 ) ) ;
#5875=CARTESIAN_POINT ( 'NONE',  ( -18.53681031552473968, 9.242445014795279690, -26.61823075656795723 ) ) ;
#5877=CARTESIAN_POINT ( 'NONE',  ( 15.61814132907574759, -26.77569883083870650, -5.000000000000000888 ) ) ;
#5881=CARTESIAN_POINT ( 'NONE',  ( -14.27740247628202397, 24.50748436584751744, -12.54751161500794510 ) ) ;
#5882=CARTESIAN_POINT ( 'NONE',  ( -18.41842359106007265, -20.67470506895122995, -16.88471669450193957 ) ) ;
#5883=CARTESIAN_POINT ( 'NONE',  ( 12.78458593907057050, -25.66269547989402611, -8.791706781336175780 ) ) ;
#5887=CARTESIAN_POINT ( 'NONE',  ( -6.900714968323537590, 23.11544720565516187, -20.95321129010784844 ) ) ;
#5893=CARTESIAN_POINT ( 'NONE',  ( 30.85552734886118031, -0.02813967135195542812, -5.946081206346901737 ) ) ;
#5896=CARTESIAN_POINT ( 'NONE',  ( 1.732915686479641781, 38.50000000000001421, -5.000000000000000000 ) ) ;
#5897=DIRECTION ( 'NONE',  ( -1.000000000000000000, 0.000000000000000000, 0.000000000000000000 ) ) ;
#5899=CARTESIAN_POINT ( 'NONE',  ( -27.14151991403504738, 0.2337522234014248468, -14.47646250802335288 ) ) ;
#5902=CARTESIAN_POINT ( 'NONE',  ( 32.37911471581676182, -6.707950149574112508, -11.21564572321703324 ) ) ;
#5908=FACE_BOUND ( 'NONE', #32186, .T. ) ;
#5917=CARTESIAN_POINT ( 'NONE',  ( 8.159785424745114923, 36.31054560068550785, -5.000000000000000000 ) ) ;
#5921=CARTESIAN_POINT ( 'NONE',  ( 18.30297387338707082, -26.76169866048132562, -8.193128520525432279 ) ) ;
#5923=CARTESIAN_POINT ( 'NONE',  ( 37.48538792151179422, -11.24999995791135809, -5.000000000000002665 ) ) ;
#5925=EDGE_LOOP ( 'NONE', ( #38579, #33830 ) ) ;
#5926=CARTESIAN_POINT ( 'NONE',  ( -11.34638386317097414, 17.63893688852765251, -26.24216709345637710 ) ) ;
#5928=CARTESIAN_POINT ( 'NONE',  ( 15.10518904483066116, -26.35922348767928014, -7.828561976387642396 ) ) ;
#5933=CARTESIAN_POINT ( 'NONE',  ( -10.07426590969644309, 18.03558095023054975, -28.02002322309929028 ) ) ;
#5934=CARTESIAN_POINT ( 'NONE',  ( -13.81792096330566544, -19.81716108706868340, -20.21201242374250739 ) ) ;
#5935=EDGE_CURVE ( 'NONE', #7759, #14281, #9172, .T. ) ;
#5938=CARTESIAN_POINT ( 'NONE',  ( -19.92632346219155437, -6.217451167954449964, -27.05300979642112935 ) ) ;
#5939=CARTESIAN_POINT ( 'NONE',  ( -13.41747663621706899, -24.08286238317321093, -13.52655550282949726 ) ) ;
#5941=ORIENTED_EDGE ( 'NONE', *, *, #9645, .T. ) ;
#5942=CARTESIAN_POINT ( 'NONE',  ( 30.37118094322071116, 0.2378720938948036268, -7.359078499018228747 ) ) ;
#5947=CARTESIAN_POINT ( 'NONE',  ( -30.97418125221157226, -0.1138930278413792935, -5.473725232278036756 ) ) ;
#5949=CARTESIAN_POINT ( 'NONE',  ( 31.47160406948570355, -0.9748322044563902944, -7.325666882419753279 ) ) ;
#5950=CIRCLE ( 'NONE', #12414, 17.00000000000000000 ) ;
#5951=CARTESIAN_POINT ( 'NONE',  ( 8.689152191311208639, -18.57991728069408310, -30.00000000000000711 ) ) ;
#5954=CARTESIAN_POINT ( 'NONE',  ( -22.49929938967337151, 2.786806827506322470, -20.78965617405635413 ) ) ;
#5955=DIRECTION ( 'NONE',  ( -0.000000000000000000, -0.000000000000000000, 1.000000000000000000 ) ) ;
#5963=CARTESIAN_POINT ( 'NONE',  ( -24.38549669577123780, 7.057000079732201669, -9.358091487992030721 ) ) ;
#5966=CARTESIAN_POINT ( 'NONE',  ( 16.73819527976525734, -18.47801620150503155, -19.92011894488071277 ) ) ;
#5968=CYLINDRICAL_SURFACE ( 'NONE', #39070, 16.00000000000000000 ) ;
#5969=CARTESIAN_POINT ( 'NONE',  ( 12.49158913934741655, 21.29194851371496355, -18.41699628959158019 ) ) ;
#5970=ORIENTED_EDGE ( 'NONE', *, *, #19001, .F. ) ;
#5971=CARTESIAN_POINT ( 'NONE',  ( -13.25082632412080486, 16.82596296396004831, -24.09658587792272399 ) ) ;
#5975=CARTESIAN_POINT ( 'NONE',  ( 11.49677055501553724, 18.42658349193868972, -23.85584982804179432 ) ) ;
#5979=CARTESIAN_POINT ( 'NONE',  ( -11.19568584489086049, 18.12681501478423840, -24.99883673433283704 ) ) ;
#5981=CARTESIAN_POINT ( 'NONE',  ( -15.59933896205200377, -26.64557334028585345, -6.883330346584703108 ) ) ;
#5983=CARTESIAN_POINT ( 'NONE',  ( -22.44268735423172245, -12.63924686016724941, -19.62614582209359426 ) ) ;
#5984=CARTESIAN_POINT ( 'NONE',  ( -7.472041749460323068, -19.13836991950213928, -29.38556132742408877 ) ) ;
#5986=CARTESIAN_POINT ( 'NONE',  ( 16.18953844785700724, 23.66664093688779857, -7.370953813631154539 ) ) ;
#5988=CARTESIAN_POINT ( 'NONE',  ( 19.95141399716809971, 5.213180036295102404, -27.65625233026011642 ) ) ;
#5992=CYLINDRICAL_SURFACE ( 'NONE', #496, 16.00000000000000000 ) ;
#5994=CARTESIAN_POINT ( 'NONE',  ( -29.19917547237594135, -0.9871674563434781335, -12.44351941946414186 ) ) ;
#5996=CARTESIAN_POINT ( 'NONE',  ( 27.19236210036768853, 0.1635435777650698363, -14.46877011068446883 ) ) ;
#6001=FACE_OUTER_BOUND ( 'NONE', #32292, .T. ) ;
#6005=CARTESIAN_POINT ( 'NONE',  ( 1.485571585149874529, -11.25000000000009415, 6.000000000000000000 ) ) ;
#6009=CARTESIAN_POINT ( 'NONE',  ( 19.48557158514982746, -11.25000000000009415, 0.000000000000000000 ) ) ;
#6010=CARTESIAN_POINT ( 'NONE',  ( 2.480770198683128314, 34.31368165843753104, -11.97966601863191727 ) ) ;
#6013=CARTESIAN_POINT ( 'NONE',  ( 15.41558956984165363, 26.78481017248027740, -5.000000000000000000 ) ) ;
#6019=CARTESIAN_POINT ( 'NONE',  ( 12.50798833650853581, 22.32269140556257625, -17.34734744980223553 ) ) ;
#6022=CARTESIAN_POINT ( 'NONE',  ( -15.42551642139064327, 13.50153766309080616, -29.41782492588997400 ) ) ;
#6026=CARTESIAN_POINT ( 'NONE',  ( 9.980411694245088228, -18.80811517553802403, -25.01294378247454731 ) ) ;
#6028=CARTESIAN_POINT ( 'NONE',  ( -19.01564406110544780, -23.98128217660448769, -13.15021722355371558 ) ) ;
#6029=CARTESIAN_POINT ( 'NONE',  ( 15.41558956916362000, 26.78481017491965233, -5.474206059968302895 ) ) ;
#6030=CARTESIAN_POINT ( 'NONE',  ( 13.20015681812674835, 22.25288346174406939, -16.44192407539625478 ) ) ;
#6033=CARTESIAN_POINT ( 'NONE',  ( -9.477158523855607086, -18.22807322462275437, -28.70867440543207749 ) ) ;
#6036=CARTESIAN_POINT ( 'NONE',  ( -29.27466627731137905, -22.93577986743095209, -7.990066130726534155 ) ) ;
#6038=CARTESIAN_POINT ( 'NONE',  ( -0.2746841415255591445, -20.81937890219735010, -25.51001604958610969 ) ) ;
#6039=CARTESIAN_POINT ( 'NONE',  ( 13.97835894188113670, 22.95206721622837520, -14.50284002566557895 ) ) ;
#6040=CARTESIAN_POINT ( 'NONE',  ( 21.44614852998417831, 11.94023807127892489, -8.409193133933671405 ) ) ;
#6042=CARTESIAN_POINT ( 'NONE',  ( -5.242313593671260818, 36.85818054513828912, -7.989178582980050791 ) ) ;
#6044=CARTESIAN_POINT ( 'NONE',  ( -26.02705243619845632, -4.035687289529959365, -17.97140994698204253 ) ) ;
#6053=CARTESIAN_POINT ( 'NONE',  ( -26.86592998902107254, 0.6294921843772121051, -14.50286829985886605 ) ) ;
#6054=CARTESIAN_POINT ( 'NONE',  ( 35.02898577490625343, -14.10520536695887017, -6.707743114419838726 ) ) ;
#6061=DIRECTION ( 'NONE',  ( -0.000000000000000000, -0.000000000000000000, -1.000000000000000000 ) ) ;
#6063=CARTESIAN_POINT ( 'NONE',  ( -2.610469631123839118, 32.22098028545256199, -13.81657025006366446 ) ) ;
#6068=CARTESIAN_POINT ( 'NONE',  ( 28.23949170197633052, -23.12056504026590886, -8.871261226031361247 ) ) ;
#6069=CARTESIAN_POINT ( 'NONE',  ( 19.81566870575805694, 14.74257314966800081, -8.893701821489321091 ) ) ;
#6070=CARTESIAN_POINT ( 'NONE',  ( 9.295215493701698861, 20.08986732679136011, -23.53424964172802092 ) ) ;
#6072=CARTESIAN_POINT ( 'NONE',  ( -20.87549224088685662, 12.48772020076265754, -9.890582243910099436 ) ) ;
#6075=CARTESIAN_POINT ( 'NONE',  ( 14.47998696515340100, -25.09368029485889906, -11.59030300758524135 ) ) ;
#6077=CARTESIAN_POINT ( 'NONE',  ( 5.636483973512840251, -22.01575377102106046, -21.50719306941234876 ) ) ;
#6078=CARTESIAN_POINT ( 'NONE',  ( -15.08663340856853452, 26.18740194786823494, -8.765449597887428723 ) ) ;
#6080=CARTESIAN_POINT ( 'NONE',  ( -24.80212611030263758, -26.15951744203449181, -6.747544335008610616 ) ) ;
#6081=CARTESIAN_POINT ( 'NONE',  ( 8.268557591513960858, -18.75831942629880444, -29.37103518859555606 ) ) ;
#6084=VERTEX_POINT ( 'NONE', #25994 ) ;
#6085=CARTESIAN_POINT ( 'NONE',  ( -7.081591661052613951, 19.23835092891137322, -29.99999999999998579 ) ) ;
#6091=CARTESIAN_POINT ( 'NONE',  ( 29.58630078773897054, 0.06066663492363379151, -10.18067296547992129 ) ) ;
#6097=CARTESIAN_POINT ( 'NONE',  ( -24.53661879515770750, 0.4792651036289722333, -18.45743660045788559 ) ) ;
#6100=CARTESIAN_POINT ( 'NONE',  ( 34.20650232967010851, -6.142903936528047559, -7.652713872589724353 ) ) ;
#6109=DIRECTION ( 'NONE',  ( 1.000000000000000000, 0.000000000000000000, 0.000000000000000000 ) ) ;
#6113=CARTESIAN_POINT ( 'NONE',  ( 9.588950291932912151, 33.22059306543958712, -9.825194817494050881 ) ) ;
#6117=CARTESIAN_POINT ( 'NONE',  ( 17.48038917147502147, -27.01406049274763177, -6.846127207748655685 ) ) ;
#6121=VECTOR ( 'NONE', #34118, 1000.000000000000000 ) ;
#6123=CARTESIAN_POINT ( 'NONE',  ( -15.18846824274939245, 26.23493944448462045, -8.298081003141406953 ) ) ;
#6126=CARTESIAN_POINT ( 'NONE',  ( 9.421039322076820710, -18.20697522973744498, -30.00000000000000000 ) ) ;
#6130=CARTESIAN_POINT ( 'NONE',  ( -13.84628348882036875, 30.44941459812471862, -5.912304033329754738 ) ) ;
#6131=CARTESIAN_POINT ( 'NONE',  ( -18.93965825742197850, -26.62254513501367015, -8.625561435589691683 ) ) ;
#6135=CARTESIAN_POINT ( 'NONE',  ( -32.71841739113132519, -9.086232289925607830, -11.15351681095390113 ) ) ;
#6137=CARTESIAN_POINT ( 'NONE',  ( -9.245064759184387526, -18.29713783020200424, -29.35345081433765202 ) ) ;
#6140=CARTESIAN_POINT ( 'NONE',  ( 22.97385260750274227, 1.506209697923000634, -20.65583506744320985 ) ) ;
#6146=CARTESIAN_POINT ( 'NONE',  ( -30.64193714844549632, -0.04498350152496895238, -7.356955191584997777 ) ) ;
#6149=CARTESIAN_POINT ( 'NONE',  ( 27.27533884161622524, -0.9703114432050143900, -15.30757276055655858 ) ) ;
#6150=DIRECTION ( 'NONE',  ( -1.000000000000000000, 0.000000000000000000, 0.000000000000000000 ) ) ;
#6153=CARTESIAN_POINT ( 'NONE',  ( -20.18092276982249444, 3.603208870470906433, -29.38994685194823830 ) ) ;
#6167=CARTESIAN_POINT ( 'NONE',  ( -22.41340355653765570, 7.689513575958383029, -14.86466521002182617 ) ) ;
#6170=CARTESIAN_POINT ( 'NONE',  ( 17.99568451041676553, -19.86586605508433934, -17.85764876952420011 ) ) ;
#6172=CARTESIAN_POINT ( 'NONE',  ( 15.07891375406595458, 26.59690363730253893, -8.285697586515082591 ) ) ;
#6174=CARTESIAN_POINT ( 'NONE',  ( -16.02335522834232506, 24.64807312034000120, -5.947261321558910296 ) ) ;
#6177=CARTESIAN_POINT ( 'NONE',  ( 11.10763664444189658, 17.47915243980666844, -27.45047991706941559 ) ) ;
#6181=CARTESIAN_POINT ( 'NONE',  ( -14.63305198900928517, 25.70517243738389368, -10.63317628927790537 ) ) ;
#6183=CARTESIAN_POINT ( 'NONE',  ( -13.84764258250596747, -24.13586365878463624, -13.50143806034850513 ) ) ;
#6187=CARTESIAN_POINT ( 'NONE',  ( -18.80552062130275459, -9.155266005175258570, -26.97371384924871407 ) ) ;
#6188=CARTESIAN_POINT ( 'NONE',  ( -9.109430062626294955, -21.71362431508917012, -18.71139059627909162 ) ) ;
#6190=CARTESIAN_POINT ( 'NONE',  ( 12.12791028434681628, 17.37686543642602288, -25.11892433193763097 ) ) ;
#6192=CARTESIAN_POINT ( 'NONE',  ( 19.64403038794415224, 5.908213622717613411, -30.00000000000000355 ) ) ;
#6195=CARTESIAN_POINT ( 'NONE',  ( -17.60052849889713400, -23.51059660007622298, -14.14515744745198056 ) ) ;
#6197=CARTESIAN_POINT ( 'NONE',  ( -20.54774503203363878, -0.4733492751199910309, -28.65983527903481942 ) ) ;
#6199=CARTESIAN_POINT ( 'NONE',  ( 31.03926838894173557, -0.2887660594600527375, -6.411557450838987648 ) ) ;
#6212=CARTESIAN_POINT ( 'NONE',  ( 1.681520345111361392, 23.68660416203806918, -21.85099733736959138 ) ) ;
#6220=CARTESIAN_POINT ( 'NONE',  ( 14.41569929962465046, 26.78900097671579772, -10.11187186520563053 ) ) ;
#6224=CARTESIAN_POINT ( 'NONE',  ( -15.18347379343816961, 14.40797193047226621, -25.41007734764195902 ) ) ;
#6229=CARTESIAN_POINT ( 'NONE',  ( 9.581194254144730138, -18.26805462278531778, -28.07681392454611213 ) ) ;
#6230=CARTESIAN_POINT ( 'NONE',  ( -15.01668844516655099, -20.19012064364629566, -19.09890700679492426 ) ) ;
#6232=CARTESIAN_POINT ( 'NONE',  ( 15.39471021437465659, 26.76682412655927124, -5.945909211790922910 ) ) ;
#6235=CARTESIAN_POINT ( 'NONE',  ( -12.55455296433269297, -22.55646857384590120, -16.45145699756288593 ) ) ;
#6237=CARTESIAN_POINT ( 'NONE',  ( -22.95124643118037611, -15.83345570903163946, -17.61049383489315900 ) ) ;
#6238=CARTESIAN_POINT ( 'NONE',  ( -0.3452383396824790784, -23.23425136565043658, -14.92058295406784296 ) ) ;
#6239=CARTESIAN_POINT ( 'NONE',  ( 15.62693799746092971, 26.04132429419060557, -5.474062535042302002 ) ) ;
#6240=CARTESIAN_POINT ( 'NONE',  ( 18.23997498585743671, 9.357756550322328337, -29.99999999999999645 ) ) ;
#6242=CARTESIAN_POINT ( 'NONE',  ( -2.977953329932500726, 21.20713377630406526, -25.62141012599427725 ) ) ;
#6244=CARTESIAN_POINT ( 'NONE',  ( -20.68522708307276048, -3.774204554019940705, -26.49279175686798382 ) ) ;
#6251=CARTESIAN_POINT ( 'NONE',  ( -30.08948457124776255, 0.6343089663011560742, -6.889917026222691199 ) ) ;
#6253=CARTESIAN_POINT ( 'NONE',  ( 31.79918597258268775, -11.65814279501285533, -12.01434721810185202 ) ) ;
#6263=CARTESIAN_POINT ( 'NONE',  ( -2.983151718949377695, 36.88695972035834103, -8.849962576356613653 ) ) ;
#6265=DIRECTION ( 'NONE',  ( 0.000000000000000000, 0.000000000000000000, 1.000000000000000000 ) ) ;
#6267=CARTESIAN_POINT ( 'NONE',  ( 29.98328813315935193, -23.06114190392259289, -6.706346631438581340 ) ) ;
#6268=CARTESIAN_POINT ( 'NONE',  ( 19.13006845375997500, 15.51315894313477983, -10.36673289579281310 ) ) ;
#6269=CARTESIAN_POINT ( 'NONE',  ( 11.98624204988562880, 26.50047453519442087, -14.18334459157481220 ) ) ;
#6271=CARTESIAN_POINT ( 'NONE',  ( -20.57814701393325763, 13.58265700682677135, -7.917366862160838181 ) ) ;
#6274=CARTESIAN_POINT ( 'NONE',  ( 15.57999310324684394, -26.64107673304671664, -6.883736562959432703 ) ) ;
#6276=CARTESIAN_POINT ( 'NONE',  ( -20.55563217186184133, -29.52600041847739476, -4.999999999999992006 ) ) ;
#6278=CARTESIAN_POINT ( 'NONE',  ( -14.52059246409109328, 25.00446786749478179, -11.59653688421371065 ) ) ;
#6279=CARTESIAN_POINT ( 'NONE',  ( -13.17255477323779544, -15.81076920432264110, -28.55881255893810078 ) ) ;
#6280=CARTESIAN_POINT ( 'NONE',  ( 8.830897544850476066, -18.97134069234825304, -26.30954933935015916 ) ) ;
#6283=CARTESIAN_POINT ( 'NONE',  ( -11.09255391874927099, 33.80179150524796228, -6.759096040517531989 ) ) ;
#6288=CARTESIAN_POINT ( 'NONE',  ( 29.77530023422455230, 0.07316830583486964856, -9.709745822606079102 ) ) ;
#6289=CARTESIAN_POINT ( 'NONE',  ( 14.95151364724920207, 28.45442998384968547, -4.999999999999999112 ) ) ;
#6292=CARTESIAN_POINT ( 'NONE',  ( -25.19426195496336263, 0.4106078367068997648, -17.44179917993732332 ) ) ;
#6295=CARTESIAN_POINT ( 'NONE',  ( 22.74347250796713027, -4.688569809066241767, -22.15124392207232873 ) ) ;
#6302=VECTOR ( 'NONE', #25874, 1000.000000000000000 ) ;
#6312=CARTESIAN_POINT ( 'NONE',  ( 6.027897580125727295, 26.69635721636051073, -17.72624810141741492 ) ) ;
#6315=CARTESIAN_POINT ( 'NONE',  ( 12.89270566647465444, -19.40238606651385211, -21.34760501390315213 ) ) ;
#6318=CARTESIAN_POINT ( 'NONE',  ( -13.22900060383164522, 22.20087300463323743, -16.44710350152914557 ) ) ;
#6320=CARTESIAN_POINT ( 'NONE',  ( 11.08661522344922190, -20.48618510043472085, -20.55290280245016632 ) ) ;
#6321=DIRECTION ( 'NONE',  ( -0.000000000000000000, -0.000000000000000000, -1.000000000000000000 ) ) ;
#6324=CARTESIAN_POINT ( 'NONE',  ( -14.22743693889722394, 29.09337559512570692, -7.745675218731769007 ) ) ;
#6325=CARTESIAN_POINT ( 'NONE',  ( -19.06118249889109606, -26.77635033892090632, -8.172094255800319118 ) ) ;
#6330=CARTESIAN_POINT ( 'NONE',  ( -33.38602273161038170, -9.282055417215806514, -10.25250355813210845 ) ) ;
#6331=CARTESIAN_POINT ( 'NONE',  ( -15.26010364459756552, -26.56150138407807404, -6.888153286160101807 ) ) ;
#6334=CARTESIAN_POINT ( 'NONE',  ( 30.29183792527964059, 0.1916456675836968604, -7.829246360666628490 ) ) ;
#6338=CARTESIAN_POINT ( 'NONE',  ( -30.81836931999540852, -0.05788259138545252813, -6.416469516946182949 ) ) ;
#6342=CARTESIAN_POINT ( 'NONE',  ( 28.89050959737125623, -1.486091803545947387, -13.35079000493364632 ) ) ;
#6344=CARTESIAN_POINT ( 'NONE',  ( 11.64820663778509058, -16.88399544672437358, -29.99999999999998579 ) ) ;
#6347=CARTESIAN_POINT ( 'NONE',  ( -26.73099083996467584, 4.407957416117326055, -7.387802156515522967 ) ) ;
#6348=CARTESIAN_POINT ( 'NONE',  ( -16.77267017368471258, -29.13948811608345935, -5.000000000000002665 ) ) ;
#6357=CARTESIAN_POINT ( 'NONE',  ( -21.91272648427093372, 6.709759433590156696, -17.91613236003459519 ) ) ;
#6360=CARTESIAN_POINT ( 'NONE',  ( 21.71680379357236745, -25.33241256410994069, -10.33255673083395543 ) ) ;
#6364=CARTESIAN_POINT ( 'NONE',  ( 15.00644039686974551, 26.44642701462099410, -8.754054474938953945 ) ) ;
#6367=CARTESIAN_POINT ( 'NONE',  ( -15.99501842261168427, 24.59332436110834408, -6.420401403374273563 ) ) ;
#6370=CARTESIAN_POINT ( 'NONE',  ( 14.85818005886212667, 25.55460827346378139, -10.18136880024061952 ) ) ;
#6374=CARTESIAN_POINT ( 'NONE',  ( -11.79361442241011027, 19.48717355318980538, -21.59818088168338690 ) ) ;
#6376=CARTESIAN_POINT ( 'NONE',  ( -9.782119759365757616, -18.39785806163243720, -26.82258960566558059 ) ) ;
#6379=CARTESIAN_POINT ( 'NONE',  ( -31.29495162020109333, -14.00799367487466185, -11.98689060328322142 ) ) ;
#6380=CARTESIAN_POINT ( 'NONE',  ( -8.378134998683849588, -20.54869970867327567, -21.89539286573533161 ) ) ;
#6382=CARTESIAN_POINT ( 'NONE',  ( 13.09240611201286519, 16.96975280483636084, -24.07475001065767017 ) ) ;
#6384=CARTESIAN_POINT ( 'NONE',  ( 26.01521168343815305, 5.578082495604143709, -5.000000000000002665 ) ) ;
#6388=VERTEX_POINT ( 'NONE', #39792 ) ;
#6389=CARTESIAN_POINT ( 'NONE',  ( -24.72616565644901243, 0.08492666307556424876, -18.40537585932330700 ) ) ;
#6392=CARTESIAN_POINT ( 'NONE',  ( 21.30732809765730806, 0.5481137214583843287, -24.98958552468036132 ) ) ;
#6394=EDGE_CURVE ( 'NONE', #33574, #19822, #5950, .T. ) ;
#6398=CARTESIAN_POINT ( 'NONE',  ( 11.41987377193677489, -19.41918266173338026, -30.00000000000000000 ) ) ;
#6405=CARTESIAN_POINT ( 'NONE',  ( 1.554709515727994651, 21.96439674343446669, -24.23040823157819545 ) ) ;
#6415=CARTESIAN_POINT ( 'NONE',  ( 11.65847521008705812, 20.47009998216675797, -20.44825086755248122 ) ) ;
#6419=CARTESIAN_POINT ( 'NONE',  ( -15.43930883336586035, 13.51924180792083519, -28.84025985046385898 ) ) ;
#6422=CARTESIAN_POINT ( 'NONE',  ( 12.28289708515961642, -22.02286693616888158, -17.43820040517785941 ) ) ;
#6423=CARTESIAN_POINT ( 'NONE',  ( -12.22510872812234339, -16.67830574990779624, -27.92440097068585203 ) ) ;
#6424=CARTESIAN_POINT ( 'NONE',  ( 12.13852697037936323, 19.91481632497913168, -20.54250373147018749 ) ) ;
#6425=CARTESIAN_POINT ( 'NONE',  ( 11.10429069022538151, 17.62735859018268059, -26.82846151514053901 ) ) ;
#6430=CARTESIAN_POINT ( 'NONE',  ( -10.78160465641473031, -20.00368079376380948, -21.62412776798347736 ) ) ;
#6432=CARTESIAN_POINT ( 'NONE',  ( -25.08679319729055734, -18.48182376974868646, -14.75278769208404839 ) ) ;
#6433=CARTESIAN_POINT ( 'NONE',  ( -0.2923764691290959283, -21.41221548788711360, -22.24809644302292710 ) ) ;
#6434=CARTESIAN_POINT ( 'NONE',  ( 15.50648612925562375, 25.79783529730770653, -7.360586758651527006 ) ) ;
#6435=CARTESIAN_POINT ( 'NONE',  ( 22.06023045062189425, 11.03359190991180938, -7.916614531392779597 ) ) ;
#6438=CARTESIAN_POINT ( 'NONE',  ( -27.56931151251565026, -3.500274113982246860, -16.06196160150427588 ) ) ;
#6445=CARTESIAN_POINT ( 'NONE',  ( -20.76830098884414966, 1.334683384510298110, -26.86827762553903298 ) ) ;
#6446=CARTESIAN_POINT ( 'NONE',  ( 19.60222645149177367, -7.245507050130505888, -27.01638570009309248 ) ) ;
#6450=DIRECTION ( 'NONE',  ( -0.000000000000000000, -0.000000000000000000, -1.000000000000000000 ) ) ;
#6451=ORIENTED_EDGE ( 'NONE', *, *, #11413, .F. ) ;
#6457=CARTESIAN_POINT ( 'NONE',  ( -4.095232911848371238, 36.67075768270702696, -8.855017135934939887 ) ) ;
#6463=CARTESIAN_POINT ( 'NONE',  ( 8.682226116870198851, 18.58302833326690262, -29.30013558004020524 ) ) ;
#6465=CARTESIAN_POINT ( 'NONE',  ( -17.67601262323927713, 10.51340875361112559, -28.30043818710294801 ) ) ;
#6467=CARTESIAN_POINT ( 'NONE',  ( 9.643767478264347659, -18.09000205506835712, -30.00000000000000000 ) ) ;
#6470=CARTESIAN_POINT ( 'NONE',  ( 13.45860491773726153, 22.88270912621719688, -15.44303183026240944 ) ) ;
#6471=CARTESIAN_POINT ( 'NONE',  ( -15.72991998290134141, -16.18894361744923316, -30.00000000000001421 ) ) ;
#6474=CARTESIAN_POINT ( 'NONE',  ( -14.52190046171712368, -14.48203382165085529, -30.00000000000001421 ) ) ;
#6475=CARTESIAN_POINT ( 'NONE',  ( 13.11109743797562466, -26.17839091903269733, -5.000000000000000888 ) ) ;
#6476=CARTESIAN_POINT ( 'NONE',  ( 13.81932564897710769, 23.28965451441122170, -14.48244069928644606 ) ) ;
#6477=CARTESIAN_POINT ( 'NONE',  ( 30.98351270641326138, -22.36505350041220197, -5.858347467683552523 ) ) ;
#6481=CARTESIAN_POINT ( 'NONE',  ( -10.13300055019763235, 34.07230637579879584, -8.053685743483509185 ) ) ;
#6486=CARTESIAN_POINT ( 'NONE',  ( 21.27281131302195760, 0.8015103380762446106, -25.01733364797255632 ) ) ;
#6490=CARTESIAN_POINT ( 'NONE',  ( -30.84974397859977557, 0.01335361837341110004, -5.474185262456348511 ) ) ;
#6493=CARTESIAN_POINT ( 'NONE',  ( 24.37211768435814108, -5.035534140336434206, -19.93691038785375369 ) ) ;
#6503=CARTESIAN_POINT ( 'NONE',  ( -19.31259245582888084, 6.905577324211579437, -30.00000000000000355 ) ) ;
#6507=CARTESIAN_POINT ( 'NONE',  ( 13.79510298735225859, 15.29130589365389703, -28.21449070774182388 ) ) ;
#6508=CARTESIAN_POINT ( 'NONE',  ( 4.803761294507334689, 21.37012296307172932, -24.35659395119734683 ) ) ;
#6510=CARTESIAN_POINT ( 'NONE',  ( 10.66098508067554995, -17.52284468788354843, -29.32387687725450220 ) ) ;
#6514=CARTESIAN_POINT ( 'NONE',  ( -14.85706654925435366, 25.55795220932581202, -10.18130676548022606 ) ) ;
#6515=CIRCLE ( 'NONE', #15003, 21.00000000000002842 ) ;
#6517=CARTESIAN_POINT ( 'NONE',  ( 14.69203212197494324, -25.92680292136585862, -9.241851185403270108 ) ) ;
#6524=CARTESIAN_POINT ( 'NONE',  ( -10.01402912130534162, 17.90039694996872655, -29.99999999999999645 ) ) ;
#6525=CARTESIAN_POINT ( 'NONE',  ( -19.16096150374591289, -26.90160068996506126, -7.719816727323686401 ) ) ;
#6528=CARTESIAN_POINT ( 'NONE',  ( -26.11057960447877946, -8.126273745962151906, -17.72871576020790130 ) ) ;
#6529=CARTESIAN_POINT ( 'NONE',  ( -15.16468140352661997, -26.46607220469503474, -7.358403229616178542 ) ) ;
#6532=CARTESIAN_POINT ( 'NONE',  ( 20.47266963615838264, 1.058032431983775723, -30.00000000000000355 ) ) ;
#6537=CARTESIAN_POINT ( 'NONE',  ( -29.61695854582710297, 0.02674555327310050579, -10.17862021117223037 ) ) ;
#6539=CARTESIAN_POINT ( 'NONE',  ( 21.05791172284567025, -0.3372447964882535620, -26.12359182236599864 ) ) ;
#6540=CARTESIAN_POINT ( 'NONE',  ( 13.28052513718836458, -15.63203832709782581, -29.99999999999999645 ) ) ;
#6544=CARTESIAN_POINT ( 'NONE',  ( -22.31696031899349464, 4.303969307314124748, -19.86790886566943470 ) ) ;
#6554=CARTESIAN_POINT ( 'NONE',  ( -24.70587413898208951, 7.101647862693369007, -7.408522823150167191 ) ) ;
#6556=CARTESIAN_POINT ( 'NONE',  ( 23.35460752408678786, -25.71782482220768173, -8.953985723103441430 ) ) ;
#6559=CARTESIAN_POINT ( 'NONE',  ( 14.43041895983224343, 25.25700966609383258, -11.57758239486862983 ) ) ;
#6561=CARTESIAN_POINT ( 'NONE',  ( -12.99709060340919820, 16.32919408374584691, -26.39889406728086030 ) ) ;
#6564=CARTESIAN_POINT ( 'NONE',  ( 15.38907305648967139, 26.61214354874361021, -6.417068104208305535 ) ) ;
#6567=EDGE_LOOP ( 'NONE', ( #15473, #19399, #10602, #29322, #37817, #21965, #14497 ) ) ;
#6568=CARTESIAN_POINT ( 'NONE',  ( -14.85275514143794062, 26.05732730074270620, -9.694811670314079421 ) ) ;
#6570=CARTESIAN_POINT ( 'NONE',  ( -15.63755959170095089, -26.78052150289263622, -5.473470747264984837 ) ) ;
#6574=CARTESIAN_POINT ( 'NONE',  ( -28.14503232587697923, -13.65727403788577377, -14.73885408196157343 ) ) ;
#6575=CARTESIAN_POINT ( 'NONE',  ( -9.042639598297487424, -18.73478658976852529, -26.88259372887121756 ) ) ;
#6577=CARTESIAN_POINT ( 'NONE',  ( 15.99681398212475081, 22.41394734825504997, -10.24358248442191943 ) ) ;
#6578=ORIENTED_EDGE ( 'NONE', *, *, #38722, .F. ) ;
#6579=CARTESIAN_POINT ( 'NONE',  ( 22.61667714053060863, 4.539058822887956701, -18.82962114486994665 ) ) ;
#6585=ORIENTED_EDGE ( 'NONE', *, *, #34125, .T. ) ;
#6586=CARTESIAN_POINT ( 'NONE',  ( -28.63560929655779219, -0.2296132274206826862, -12.51332363996011310 ) ) ;
#6587=CARTESIAN_POINT ( 'NONE',  ( 28.61027353976883347, -0.1971735349054578590, -12.51648547223809160 ) ) ;
#6592=CARTESIAN_POINT ( 'NONE',  ( 7.289639608743136989, -27.06962010326278545, -13.42901749168595593 ) ) ;
#6597=DIRECTION ( 'NONE',  ( -1.000000000000000000, 0.000000000000000000, 0.000000000000000000 ) ) ;
#6598=CARTESIAN_POINT ( 'NONE',  ( 0.8480541672973396228, 20.90088328258439887, -26.96762484265282112 ) ) ;
#6599=DIRECTION ( 'NONE',  ( 0.000000000000000000, 0.000000000000000000, 1.000000000000000000 ) ) ;
#6605=CARTESIAN_POINT ( 'NONE',  ( 10.28246022096949908, 18.16882197377053032, -26.75189561797980531 ) ) ;
#6608=CARTESIAN_POINT ( 'NONE',  ( -18.68025062537304493, 17.59719118396984072, -6.925800422574094561 ) ) ;
#6611=EDGE_CURVE ( 'NONE', #12248, #12299, #33859, .T. ) ;
#6613=CARTESIAN_POINT ( 'NONE',  ( 15.34965201500932785, -26.58387937520311084, -6.887971616833333144 ) ) ;
#6614=CARTESIAN_POINT ( 'NONE',  ( -20.58361896323833307, -25.87753243228978661, -9.918039572038674478 ) ) ;
#6615=CARTESIAN_POINT ( 'NONE',  ( 13.21227310165477320, 22.23035794993680270, -16.44475469494696540 ) ) ;
#6616=CARTESIAN_POINT ( 'NONE',  ( 11.67513080692914151, 18.92206925029848108, -22.73326350911885285 ) ) ;
#6619=CARTESIAN_POINT ( 'NONE',  ( -14.85743854809297737, -25.96320633999491179, -9.239818057270476004 ) ) ;
#6622=CARTESIAN_POINT ( 'NONE',  ( -31.09129472269700756, -21.46021889108168779, -7.549027889585831375 ) ) ;
#6623=CARTESIAN_POINT ( 'NONE',  ( -1.777045556556341888, -20.53114539011956197, -28.29789199099749908 ) ) ;
#6624=CARTESIAN_POINT ( 'NONE',  ( 12.21857019178368020, 19.03452810332261080, -21.67269469152422445 ) ) ;
#6626=CARTESIAN_POINT ( 'NONE',  ( 22.75140569375547983, 10.14465275586799997, -6.451765741814347699 ) ) ;
#6630=CARTESIAN_POINT ( 'NONE',  ( -32.38786556318342491, -4.220081569580368175, -9.945407286558161530 ) ) ;
#6637=CARTESIAN_POINT ( 'NONE',  ( -30.25911448991262276, 0.6236314785230304691, -5.474043737439959756 ) ) ;
#6639=CARTESIAN_POINT ( 'NONE',  ( 19.31437624530733643, -7.140418407204370155, -28.47186176483214837 ) ) ;
#6650=CARTESIAN_POINT ( 'NONE',  ( -2.423886253481512210, 30.01527867101077973, -15.69239631665445422 ) ) ;
#6651=DIRECTION ( 'NONE',  ( -0.000000000000000000, -0.000000000000000000, 1.000000000000000000 ) ) ;
#6655=ADVANCED_FACE ( 'NONE', ( #10313 ), #7457, .T. ) ;
#6657=CARTESIAN_POINT ( 'NONE',  ( 12.24878116420049068, 29.33560266281129358, -11.31652717080035231 ) ) ;
#6659=CARTESIAN_POINT ( 'NONE',  ( -21.25484840722362279, 12.72181903587277318, -5.483107197446321024 ) ) ;
#6662=CARTESIAN_POINT ( 'NONE',  ( 14.92053913355477590, -25.84391472125183498, -9.706504376371448473 ) ) ;
#6664=CARTESIAN_POINT ( 'NONE',  ( 11.64760469399007725, 18.94855002001494171, -22.72844738028206635 ) ) ;
#6665=CARTESIAN_POINT ( 'NONE',  ( 31.47283671532267846, -25.12609584734865464, -5.000000000000006217 ) ) ;
#6668=CARTESIAN_POINT ( 'NONE',  ( -23.35727036480124852, -23.34227582478836993, -12.07518644368831850 ) ) ;
#6669=CARTESIAN_POINT ( 'NONE',  ( 11.11180036078298272, -23.01599423131538558, -15.57141518415062720 ) ) ;
#6670=CARTESIAN_POINT ( 'NONE',  ( 12.26164114550799944, 19.76946988966989949, -20.56397771860881107 ) ) ;
#6671=CARTESIAN_POINT ( 'NONE',  ( 29.43405427299785515, -21.28324550421933381, -9.736337039119780101 ) ) ;
#6676=CARTESIAN_POINT ( 'NONE',  ( -5.620579596833452207, 21.10756638118547457, -24.41133304458605124 ) ) ;
#6678=VECTOR ( 'NONE', #39300, 1000.000000000000000 ) ;
#6681=CARTESIAN_POINT ( 'NONE',  ( 30.83224212302263822, -0.07211122296361122119, -6.416159285224059872 ) ) ;
#6685=CARTESIAN_POINT ( 'NONE',  ( -25.83958759730864685, 0.3586317713515524974, -16.44731683257352373 ) ) ;
#6686=CARTESIAN_POINT ( 'NONE',  ( -20.57926082973601822, -27.21289976943432265, -4.999999999999998224 ) ) ;
#6689=CARTESIAN_POINT ( 'NONE',  ( 20.94073701540919075, -3.630281487320123457, -25.85615716460149827 ) ) ;
#6700=CARTESIAN_POINT ( 'NONE',  ( -19.98575265377075993, -4.745023977884823552, -30.00000000000000355 ) ) ;
#6701=MECHANICAL_DESIGN_GEOMETRIC_PRESENTATION_REPRESENTATION('',(#5414),#8666);
#6704=CARTESIAN_POINT ( 'NONE',  ( 17.65119513763062287, 19.95841547798437077, -6.914159246569045791 ) ) ;
#6705=CARTESIAN_POINT ( 'NONE',  ( 9.937273488330333748, 34.60605125810194949, -7.177303487740063659 ) ) ;
#6707=CARTESIAN_POINT ( 'NONE',  ( 13.44315901770257682, -21.33295835193786516, -18.26921127929339050 ) ) ;
#6711=CARTESIAN_POINT ( 'NONE',  ( -14.85137426362708624, 25.57504807805499070, -10.18098964417948693 ) ) ;
#6714=CARTESIAN_POINT ( 'NONE',  ( 11.69482082898245956, -21.50151594381998166, -18.47287864288130876 ) ) ;
#6718=CARTESIAN_POINT ( 'NONE',  ( -13.11788538660038306, 24.75960143229000110, -14.33734891237946130 ) ) ;
#6719=CARTESIAN_POINT ( 'NONE',  ( -12.40276990898003895, -16.90054566293658667, -26.59307398587640137 ) ) ;
#6722=CARTESIAN_POINT ( 'NONE',  ( -25.24452815043373022, -7.038082672387002248, -18.79164011408699153 ) ) ;
#6723=CARTESIAN_POINT ( 'NONE',  ( -15.01606105974973104, -26.24525916788589086, -8.298880598885562065 ) ) ;
#6726=CARTESIAN_POINT ( 'NONE',  ( 30.16006263997094550, 0.2005578054670466015, -8.299689423995275206 ) ) ;
#6727=CARTESIAN_POINT ( 'NONE',  ( 11.30648189679965654, 18.04080162749803407, -25.01410075632841412 ) ) ;
#6732=CARTESIAN_POINT ( 'NONE',  ( -21.27998365777518330, 0.7502355399091473753, -25.01178682489351601 ) ) ;
#6734=CARTESIAN_POINT ( 'NONE',  ( 31.94105064681168571, -2.205082878242727862, -8.660796739423290092 ) ) ;
#6736=CARTESIAN_POINT ( 'NONE',  ( -3.357890496178010054, -20.26885263950605420, -30.00000000000000000 ) ) ;
#6748=VECTOR ( 'NONE', #18722, 1000.000000000000000 ) ;
#6751=CARTESIAN_POINT ( 'NONE',  ( -18.95922262551748361, 7.795319610833783663, -30.00000000000000000 ) ) ;
#6752=CARTESIAN_POINT ( 'NONE',  ( 18.71898351499973145, -19.47505160051558448, -17.80877851765054132 ) ) ;
#6753=CARTESIAN_POINT ( 'NONE',  ( -20.71630303010418572, -29.20803740758281464, -4.999999999999997335 ) ) ;
#6754=CARTESIAN_POINT ( 'NONE',  ( 15.23567902583548417, 26.71743813441107207, -7.352606933093872144 ) ) ;
#6755=VERTEX_POINT ( 'NONE', #26356 ) ;
#6757=CARTESIAN_POINT ( 'NONE',  ( -15.60993106802417252, 25.69096736691974669, -6.890080393197788311 ) ) ;
#6762=CARTESIAN_POINT ( 'NONE',  ( 15.31233209253673699, 26.45408978173025005, -7.358089053015683945 ) ) ;
#6766=CARTESIAN_POINT ( 'NONE',  ( -14.91657227004425934, 26.29114371075054990, -9.222413299652547636 ) ) ;
#6768=CARTESIAN_POINT ( 'NONE',  ( -14.82334245325438538, -25.50166360968241719, -10.64068735651913578 ) ) ;
#6771=CARTESIAN_POINT ( 'NONE',  ( -34.86194987718285176, -15.64482351731836474, -5.858316081785087448 ) ) ;
#6772=CARTESIAN_POINT ( 'NONE',  ( -14.14861525076418580, -26.29469343071681209, -6.890863552359059341 ) ) ;
#6774=CARTESIAN_POINT ( 'NONE',  ( 12.68075659042399117, 16.15066152451087689, -28.76951523894423701 ) ) ;
#6776=CARTESIAN_POINT ( 'NONE',  ( 25.68561304534730283, 5.556133728777049363, -8.363004190235322710 ) ) ;
#6781=CARTESIAN_POINT ( 'NONE',  ( -25.58894034025924213, -0.3267592592326616363, -17.34686670204293435 ) ) ;
#6783=CARTESIAN_POINT ( 'NONE',  ( 31.11181571040396321, -0.2945068792762812193, -5.942526464314708434 ) ) ;
#6788=CARTESIAN_POINT ( 'NONE',  ( -37.49625565938783467, -14.69322820095469240, -5.000000000000006217 ) ) ;
#6794=CARTESIAN_POINT ( 'NONE',  ( 16.17302619178590462, 24.05975780865501790, -4.999999999999999112 ) ) ;
#6795=CARTESIAN_POINT ( 'NONE',  ( 4.921717144059290838, 36.96778581912766271, -7.986823970829891373 ) ) ;
#6803=CARTESIAN_POINT ( 'NONE',  ( 15.22299664760056537, 27.42699395385487904, -5.000000000000000000 ) ) ;
#6806=CARTESIAN_POINT ( 'NONE',  ( -16.30574288886405654, 14.63324257956979224, -21.08092481694252029 ) ) ;
#6810=CARTESIAN_POINT ( 'NONE',  ( 9.486164890912217373, -18.17313361576023212, -30.00000000000000000 ) ) ;
#6813=CARTESIAN_POINT ( 'NONE',  ( 11.89393184209717624, 19.38028970819429020, -21.61737904418150436 ) ) ;
#6815=CARTESIAN_POINT ( 'NONE',  ( 10.96874445820387223, 17.31868006298826046, -30.00000000000000000 ) ) ;
#6819=CARTESIAN_POINT ( 'NONE',  ( -11.84263605179389778, -21.48980687254330846, -18.45847382795814795 ) ) ;
#6821=VECTOR ( 'NONE', #36454, 1000.000000000000000 ) ;
#6823=CARTESIAN_POINT ( 'NONE',  ( -28.89889151792434063, -21.30051352786605179, -10.18607909959966840 ) ) ;
#6824=CARTESIAN_POINT ( 'NONE',  ( -4.782499769022778402, -24.84304998847331092, -6.931069079744395012 ) ) ;
#6825=CARTESIAN_POINT ( 'NONE',  ( 12.08418194466055695, 18.52621323336339287, -22.79847468729924742 ) ) ;
#6827=CARTESIAN_POINT ( 'NONE',  ( 18.77593942704109509, 8.755078447771618144, -26.61273691426299592 ) ) ;
#6831=CARTESIAN_POINT ( 'NONE',  ( -33.48494503266941535, -3.494085805712010107, -5.909783893160384771 ) ) ;
#6836=CARTESIAN_POINT ( 'NONE',  ( -28.42036332966587509, 2.623993810986072095, -5.000000000000000000 ) ) ;
#6838=CARTESIAN_POINT ( 'NONE',  ( 19.38136568836685925, -7.835196129137437460, -26.99971740741212756 ) ) ;
#6840=ORIENTED_EDGE ( 'NONE', *, *, #9229, .T. ) ;
#6849=CARTESIAN_POINT ( 'NONE',  ( -0.7383155542429340468, 37.49228970066121747, -8.404103827552029671 ) ) ;
#6855=CARTESIAN_POINT ( 'NONE',  ( 10.39566615896967683, 22.74892090402041944, -19.14879625716820044 ) ) ;
#6858=CARTESIAN_POINT ( 'NONE',  ( -19.27084013280208197, 11.49840606477986071, -18.02072584537811650 ) ) ;
#6861=CARTESIAN_POINT ( 'NONE',  ( 9.609346625839055633, -18.25387553414934771, -28.07524107909567590 ) ) ;
#6863=CARTESIAN_POINT ( 'NONE',  ( 14.91174806184727153, 25.87366738573922120, -9.704845141577239431 ) ) ;
#6865=CARTESIAN_POINT ( 'NONE',  ( 5.636483973512839363, -22.01575377102105691, -30.00000000000001421 ) ) ;
#6868=CARTESIAN_POINT ( 'NONE',  ( -14.97360822305132722, -15.86213100947220944, -24.45481922633826599 ) ) ;
#6869=CARTESIAN_POINT ( 'NONE',  ( 7.307221220942812678, -22.95671206205766524, -15.78720648459951192 ) ) ;
#6870=CARTESIAN_POINT ( 'NONE',  ( 15.49934645862682103, 26.48612375915841710, -5.474131244744144809 ) ) ;
#6871=CARTESIAN_POINT ( 'NONE',  ( 16.96937371531925365, -12.22095849417253532, -26.98299665146808834 ) ) ;
#6875=CARTESIAN_POINT ( 'NONE',  ( -6.226819983209127329, 23.40422832001528519, -20.90460070830227224 ) ) ;
#6880=CARTESIAN_POINT ( 'NONE',  ( 21.71290527652266888, 0.7082383630531658980, -23.85174149327086113 ) ) ;
#6885=CARTESIAN_POINT ( 'NONE',  ( -23.92393967644365915, 0.5257180683408601007, -19.50104800721178577 ) ) ;
#6889=CARTESIAN_POINT ( 'NONE',  ( 20.09314088254942021, -4.111701498484372053, -29.99999999999998579 ) ) ;
#6900=CARTESIAN_POINT ( 'NONE',  ( -10.25710140050888519, 17.79863391756059698, -30.00000000000000000 ) ) ;
#6903=CARTESIAN_POINT ( 'NONE',  ( 18.00529160253907079, 18.80124742017171968, -7.886222486033878099 ) ) ;
#6904=CARTESIAN_POINT ( 'NONE',  ( 5.103355680224398228, 19.86390335519187289, -30.00000000000000355 ) ) ;
#6907=CARTESIAN_POINT ( 'NONE',  ( 10.39682445600779026, -18.27815074178298360, -26.16533906555415356 ) ) ;
#6913=CARTESIAN_POINT ( 'NONE',  ( -13.49222746860650624, 22.81367680405242382, -15.45099856532659643 ) ) ;
#6915=CARTESIAN_POINT ( 'NONE',  ( 13.01178723928756575, -23.59175502374137778, -14.49606265435651764 ) ) ;
#6916=FACE_OUTER_BOUND ( 'NONE', #14736, .T. ) ;
#6919=CARTESIAN_POINT ( 'NONE',  ( -13.17720483057398972, 28.77380982630769424, -10.45774930547776904 ) ) ;
#6920=CARTESIAN_POINT ( 'NONE',  ( -14.51034694435784722, -19.54383023510037276, -20.13759940241521207 ) ) ;
#6922=CARTESIAN_POINT ( 'NONE',  ( -27.13658926588106723, -5.861905960888289080, -16.87029009801329593 ) ) ;
#6925=CARTESIAN_POINT ( 'NONE',  ( 20.47688798105681940, 0.9740165025114797537, -29.35045312999529799 ) ) ;
#6929=CARTESIAN_POINT ( 'NONE',  ( -30.92750986253986767, -0.06599190286722676768, -5.474045238037080985 ) ) ;
#6933=CARTESIAN_POINT ( 'NONE',  ( 20.88296681861968551, -0.3172434910415447007, -26.74114674371728029 ) ) ;
#6947=CARTESIAN_POINT ( 'NONE',  ( -22.14118475150960563, 9.614454132667919595, -11.87011620208269314 ) ) ;
#6948=CARTESIAN_POINT ( 'NONE',  ( 20.22886225973998719, -23.64398365531091528, -13.09675354266916258 ) ) ;
#6949=CARTESIAN_POINT ( 'NONE',  ( 11.20572440089081390, 18.11902114148211851, -25.00021980855870396 ) ) ;
#6952=CARTESIAN_POINT ( 'NONE',  ( -12.63699674669057949, 17.97954234152161490, -22.88184407339303661 ) ) ;
#6956=CARTESIAN_POINT ( 'NONE',  ( 11.71173409423554190, 18.88690681544503391, -22.73936493488036703 ) ) ;
#6958=CARTESIAN_POINT ( 'NONE',  ( 33.01650362960521079, -18.20503022527935855, -7.971919029728472772 ) ) ;
#6963=CARTESIAN_POINT ( 'NONE',  ( -15.09307680312074140, 26.86446856943478423, -7.812756861724547974 ) ) ;
#6965=CARTESIAN_POINT ( 'NONE',  ( -14.00048334364361402, -23.68480630221392147, -14.41671907191942559 ) ) ;
#6969=CARTESIAN_POINT ( 'NONE',  ( -23.12572148637181257, -11.24311462695209585, -19.64121234349231315 ) ) ;
#6970=CARTESIAN_POINT ( 'NONE',  ( -12.26289438224282158, -23.05663733951990935, -15.49923916903545340 ) ) ;
#6972=CARTESIAN_POINT ( 'NONE',  ( 15.87663021223514548, 23.08495078608549633, -9.753722227093680530 ) ) ;
#6974=CARTESIAN_POINT ( 'NONE',  ( 27.02756462025498152, 2.904459085774969473, -10.73325283292277099 ) ) ;
#6979=CARTESIAN_POINT ( 'NONE',  ( -22.92914194212210788, -0.07278265280095547185, -21.52489520804394019 ) ) ;
#6980=CARTESIAN_POINT ( 'NONE',  ( 22.27536895993342014, 0.4410975482186068053, -22.70620645469208654 ) ) ;
#6982=ORIENTED_EDGE ( 'NONE', *, *, #19398, .T. ) ;
#6984=CARTESIAN_POINT ( 'NONE',  ( -35.84808252048276955, -3.038699442442200027, -5.000000000000002665 ) ) ;
#6994=CARTESIAN_POINT ( 'NONE',  ( 17.06447150072999719, 21.55760828791484585, -5.000000000000003553 ) ) ;
#6995=CARTESIAN_POINT ( 'NONE',  ( 5.880870157263162312, 35.77077879190645149, -9.310133446813710023 ) ) ;
#7000=CARTESIAN_POINT ( 'NONE',  ( 17.14449823358358316, -14.87368394026793972, -23.09499826230010200 ) ) ;
#7001=B_SPLINE_CURVE_WITH_KNOTS ( 'NONE', 3,
 ( #31839, #25536, #31642, #23098, #16814, #22488, #1168, #10508, #4004, #32249, #3807, #29200, #7047, #16405, #967, #13348, #32042, #25739, #22691, #35091 ),
 .UNSPECIFIED., .F., .F.,
 ( 4, 2, 1, 1, 1, 1, 1, 1, 2, 2, 2, 2, 4 ),
 ( 0.000000000000000000, 0.0009765625000000435849, 0.001953125000000087170, 0.003906250000000174340, 0.007812500000000305311, 0.01562500000000027409, 0.03125000000000020817, 0.06250000000000018041, 0.1250000000000000278, 0.2499999999999998890, 0.5000000000000000000, 0.7500000000000000000, 1.000000000000000000 ),
 .UNSPECIFIED. ) ;
#7005=CARTESIAN_POINT ( 'NONE',  ( 15.13246232760047505, 27.45171539379471781, -6.404961841383983945 ) ) ;
#7008=CARTESIAN_POINT ( 'NONE',  ( -16.71939040854026715, 19.69829189495437305, -11.75715933036468286 ) ) ;
#7012=CARTESIAN_POINT ( 'NONE',  ( 10.22002048505811800, -19.16611505460419806, -23.85456539383813990 ) ) ;
#7014=CARTESIAN_POINT ( 'NONE',  ( 13.21628872672062194, 22.22346690588532425, -16.44513725962594819 ) ) ;
#7016=CARTESIAN_POINT ( 'NONE',  ( 15.33694215129142790, 26.62211003415141164, -6.887897498730079171 ) ) ;
#7018=CARTESIAN_POINT ( 'NONE',  ( -13.75448907894945805, 23.42996800784982270, -14.47271240302549700 ) ) ;
#7020=CARTESIAN_POINT ( 'NONE',  ( -10.82815314884593860, -19.99260957008704409, -21.61855094834904989 ) ) ;
#7023=CARTESIAN_POINT ( 'NONE',  ( -30.92874242133839502, -21.35189250303394815, -7.976690102107105496 ) ) ;
#7024=CARTESIAN_POINT ( 'NONE',  ( -3.280732279199019441, -20.30841954709158870, -28.85152870245993739 ) ) ;
#7025=CARTESIAN_POINT ( 'NONE',  ( 15.59458766223087167, 25.74192377969740519, -6.889944325882612297 ) ) ;
#7027=VERTEX_POINT ( 'NONE', #6013 ) ;
#7028=CARTESIAN_POINT ( 'NONE',  ( 20.04105427597066225, 10.14435442418174738, -18.01185279135228257 ) ) ;
#7034=CARTESIAN_POINT ( 'NONE',  ( -30.79476031969355176, -3.968954442311656283, -12.24617189075128643 ) ) ;
#7039=CARTESIAN_POINT ( 'NONE',  ( 19.48557158514975285, -11.24999999999995737, 10.00000000000000000 ) ) ;
#7040=CARTESIAN_POINT ( 'NONE',  ( 34.65956455088738153, -16.45432426470986798, -4.999999999999995559 ) ) ;
#7047=CARTESIAN_POINT ( 'NONE',  ( -17.56752247727831673, 20.37189381199461025, -4.999999999999999112 ) ) ;
#7052=CARTESIAN_POINT ( 'NONE',  ( -0.5950768495228482280, 30.23063772115626691, -15.67701037968547872 ) ) ;
#7059=CARTESIAN_POINT ( 'NONE',  ( 10.89816891502054830, 21.26322318888422558, -20.31437330493695370 ) ) ;
#7062=CARTESIAN_POINT ( 'NONE',  ( -19.67958062024562338, 15.63688475377917086, -5.964679019702594509 ) ) ;
#7065=CARTESIAN_POINT ( 'NONE',  ( 10.88014080686398977, -19.98056130176378531, -21.61155136698059209 ) ) ;
#7067=CARTESIAN_POINT ( 'NONE',  ( 11.44734449680894350, 18.46921977093748524, -23.84809478162342700 ) ) ;
#7068=CARTESIAN_POINT ( 'NONE',  ( 2.927345865710861972E-15, 22.57051819516765789, -19.69475445967420768 ) ) ;
#7071=CARTESIAN_POINT ( 'NONE',  ( -17.16483700087839992, -17.10857606624298199, -20.90193344114118190 ) ) ;
#7072=CARTESIAN_POINT ( 'NONE',  ( 6.178680871570535693, -24.89148437011798620, -7.894064581684323123 ) ) ;
#7073=CARTESIAN_POINT ( 'NONE',  ( 11.32202086828915100, 17.65615535816628423, -26.23948895313833063 ) ) ;
#7074=CARTESIAN_POINT ( 'NONE',  ( 30.42719773241262260, -20.61230597470657955, -9.287414125035716950 ) ) ;
#7078=CARTESIAN_POINT ( 'NONE',  ( -6.993233941076627325, 29.63588997363762090, -14.83726457422114287 ) ) ;
#7082=CARTESIAN_POINT ( 'NONE',  ( 25.88303574148295993, 0.2867772994816546461, -16.43952562929733219 ) ) ;
#7087=PRODUCT ( 'Detachable Washable Trimmer Head Cap', 'Detachable Washable Trimmer Head Cap', '', ( #29641 ) ) ;
#7089=CARTESIAN_POINT ( 'NONE',  ( -20.48011438624494218, 0.9027161730473580725, -30.00000000000000000 ) ) ;
#7092=CARTESIAN_POINT ( 'NONE',  ( 35.44138113946621615, -9.599287445864765900, -5.442910742026312754 ) ) ;
#7104=SHAPE_REPRESENTATION_RELATIONSHIP ( 'NONE' , 'NONE' ,  #8618, #23086 ) ;
#7105=CARTESIAN_POINT ( 'NONE',  ( 3.057012479096308688, 20.28136394534261555, -30.00000000000001066 ) ) ;
#7108=CARTESIAN_POINT ( 'NONE',  ( 18.14143768169351034, 18.99352574702872687, -5.000000000000003553 ) ) ;
#7109=CARTESIAN_POINT ( 'NONE',  ( 8.803475244830952562, 27.36709591607177572, -15.90040107698557570 ) ) ;
#7112=CARTESIAN_POINT ( 'NONE',  ( 12.87862734366817108, -22.00492508238036393, -17.36953957828150763 ) ) ;
#7117=ORIENTED_EDGE ( 'NONE', *, *, #18338, .T. ) ;
#7118=CARTESIAN_POINT ( 'NONE',  ( -11.31322392688638523, 18.03553487960044777, -25.01503145050758548 ) ) ;
#7120=CARTESIAN_POINT ( 'NONE',  ( 14.44676625670391168, -25.74302676979435134, -9.715428041659723846 ) ) ;
#7123=ORIENTED_EDGE ( 'NONE', *, *, #33006, .T. ) ;
#7125=CARTESIAN_POINT ( 'NONE',  ( -8.515539604177867261, 19.39886015949181441, -25.95454680849416462 ) ) ;
#7129=CARTESIAN_POINT ( 'NONE',  ( -35.08557715296313262, -7.694570891656546507, -5.000000000000002665 ) ) ;
#7132=CARTESIAN_POINT ( 'NONE',  ( 20.95308506363175738, 0.9643035589587092282, -26.23839846377317997 ) ) ;
#7136=CARTESIAN_POINT ( 'NONE',  ( -30.19800961909351855, -0.002553536262527825347, -8.766955577734158567 ) ) ;
#7139=CARTESIAN_POINT ( 'NONE',  ( 20.45006009983584860, -1.583034825077791696, -29.30351957104910809 ) ) ;
#7140=CARTESIAN_POINT ( 'NONE',  ( 20.49802635999024147, 0.7366814822345414404, -30.00000000000001066 ) ) ;
#7142=ORIENTED_EDGE ( 'NONE', *, *, #12587, .F. ) ;
#7147=CARTESIAN_POINT ( 'NONE',  ( -20.71630303010418572, -29.20803740758281464, -4.999999999999997335 ) ) ;
#7156=CARTESIAN_POINT ( 'NONE',  ( -22.51939234098515996, 9.738838319951677036, -9.880579217825056659 ) ) ;
#7157=CARTESIAN_POINT ( 'NONE',  ( 15.50525388175314312, -18.17829242494390130, -21.05556129404982002 ) ) ;
#7158=CARTESIAN_POINT ( 'NONE',  ( -28.16747440122964008, -24.83813135940263805, -4.999999999999999112 ) ) ;
#7161=CARTESIAN_POINT ( 'NONE',  ( 14.47143598563519085, 25.14360450831679117, -11.58605191478856078 ) ) ;
#7163=CARTESIAN_POINT ( 'NONE',  ( -13.27773080846810672, 20.14855683102708284, -18.55665866639438022 ) ) ;
#7167=CARTESIAN_POINT ( 'NONE',  ( 15.12875536725216463, 26.04897481050989683, -8.768510653149395040 ) ) ;
#7169=CARTESIAN_POINT ( 'NONE',  ( 24.45946707268589293, -13.48901220950923019, -17.59677725036030793 ) ) ;
#7173=CARTESIAN_POINT ( 'NONE',  ( -14.54989670408210500, 25.93872036832522454, -10.61834747045229399 ) ) ;
#7175=CARTESIAN_POINT ( 'NONE',  ( -15.30846161082977197, -25.59754758358769777, -10.61048781664426599 ) ) ;
#7176=CARTESIAN_POINT ( 'NONE',  ( -19.48557158514985588, -11.25000000000002309, 6.000000000000000000 ) ) ;
#7178=CARTESIAN_POINT ( 'NONE',  ( -34.78882160387538391, -14.36995147936751138, -7.130009219520698771 ) ) ;
#7179=CARTESIAN_POINT ( 'NONE',  ( -14.51760670474123671, -26.47485642095533365, -5.946377559672243684 ) ) ;
#7181=CARTESIAN_POINT ( 'NONE',  ( 13.19356601497149839, 17.97120000216638047, -21.82600956427421579 ) ) ;
#7183=CARTESIAN_POINT ( 'NONE',  ( 27.98880052845386501, 2.891254499028016234, -7.376140888623180736 ) ) ;
#7187=CARTESIAN_POINT ( 'NONE',  ( -27.95296816494704117, -0.09156375941248461048, -13.48332082428012768 ) ) ;
#7188=CARTESIAN_POINT ( 'NONE',  ( 20.71295742291022890, 0.5317868688435807289, -27.42788539693542305 ) ) ;
#7193=CARTESIAN_POINT ( 'NONE',  ( -8.937590682902627037, -20.71651963383551731, -21.24786896499727007 ) ) ;
#7204=CARTESIAN_POINT ( 'NONE',  ( 16.36039051805071765, -13.34769688759530482, -26.31117674288608654 ) ) ;
#7207=CARTESIAN_POINT ( 'NONE',  ( 14.77749770927584549, 26.69806964646038239, -9.202908815035055312 ) ) ;
#7211=CARTESIAN_POINT ( 'NONE',  ( -15.32646819449677800, 15.98035180726021665, -20.99571673828884144 ) ) ;
#7214=CARTESIAN_POINT ( 'NONE',  ( 15.41329945644580413, -26.72332452139117720, -5.474185070702327849 ) ) ;
#7216=CARTESIAN_POINT ( 'NONE',  ( 11.89771786224719285, 19.37622671090241511, -21.61810800180225911 ) ) ;
#7218=CARTESIAN_POINT ( 'NONE',  ( 15.28841811250725868, 26.53669736298195048, -7.357800263959026310 ) ) ;
#7220=CARTESIAN_POINT ( 'NONE',  ( -15.26742702018640507, 26.60978498224415745, -7.355557875012173952 ) ) ;
#7221=LINE ( 'NONE', #16991, #29597 ) ;
#7222=CARTESIAN_POINT ( 'NONE',  ( -15.45423376311904917, -26.70816042823125613, -5.946215788419346282 ) ) ;
#7224=CARTESIAN_POINT ( 'NONE',  ( -22.04784006917977379, -13.31140231594222634, -19.62697991373520878 ) ) ;
#7225=CARTESIAN_POINT ( 'NONE',  ( -7.052297394767913730, -25.17996142191265463, -4.999999999999999112 ) ) ;
#7226=CARTESIAN_POINT ( 'NONE',  ( 12.76514706875002858, 19.99879491202248261, -19.56037735346854589 ) ) ;
#7228=CARTESIAN_POINT ( 'NONE',  ( 19.37711718808892769, 7.349286276001018692, -26.58382230141096159 ) ) ;
#7229=CARTESIAN_POINT ( 'NONE',  ( 33.31689420198952689, -19.38461815459663029, -5.000000000000000000 ) ) ;
#7231=CARTESIAN_POINT ( 'NONE',  ( -13.11868842595538176, -26.17317209596299321, -5.000000000000001776 ) ) ;
#7234=CARTESIAN_POINT ( 'NONE',  ( -31.49989133076260117, -4.076527785121538905, -11.31888596494559529 ) ) ;
#7239=CARTESIAN_POINT ( 'NONE',  ( 20.85651332716498274, -9.164426480176581791, -23.02215317269795847 ) ) ;
#7250=CARTESIAN_POINT ( 'NONE',  ( -1.858046560160577565, 36.81141413151663500, -9.283575669460820023 ) ) ;
#7257=CARTESIAN_POINT ( 'NONE',  ( 9.856912408380251733, 19.70089498851076470, -23.61131346103714890 ) ) ;
#7260=CARTESIAN_POINT ( 'NONE',  ( -17.30414937619200799, 11.17673895782788485, -27.73534995255125324 ) ) ;
#7262=DIRECTION ( 'NONE',  ( 1.000000000000000000, 0.000000000000000000, 0.000000000000000000 ) ) ;
#7263=CARTESIAN_POINT ( 'NONE',  ( 15.30027160615963844, -26.40643539529997241, -7.826203141063676760 ) ) ;
#7265=CARTESIAN_POINT ( 'NONE',  ( 12.11308143205599919, 19.94536299475516472, -20.53731574209467681 ) ) ;
#7266=CARTESIAN_POINT ( 'NONE',  ( -22.52744239175981278, -0.1803094636421871677, -30.00000000000000000 ) ) ;
#7268=CARTESIAN_POINT ( 'NONE',  ( -21.36603670794792009, -21.34451933144417879, -14.86881065236695143 ) ) ;
#7270=CARTESIAN_POINT ( 'NONE',  ( 8.200574578750897459, -24.73362697332168736, -9.819646422388172979 ) ) ;
#7271=CARTESIAN_POINT ( 'NONE',  ( 12.74342753841739118, 20.92241134701107441, -18.46772647367177100 ) ) ;
#7272=CARTESIAN_POINT ( 'NONE',  ( 20.33298947872574658, 13.79308491711421247, -8.897425670759471217 ) ) ;
#7278=CARTESIAN_POINT ( 'NONE',  ( -9.263779654156028442, 34.90887495674188301, -7.602959551972078067 ) ) ;
#7282=CARTESIAN_POINT ( 'NONE',  ( 26.51902585559564685, 0.2539472759805578295, -15.44871964324930325 ) ) ;
#7286=CARTESIAN_POINT ( 'NONE',  ( -29.45261839425941375, 0.2115709630840172106, -10.18423039480368431 ) ) ;
#7289=CARTESIAN_POINT ( 'NONE',  ( 28.18850087859003040, -7.572030850641755961, -15.83067351684029589 ) ) ;
#7301=CARTESIAN_POINT ( 'NONE',  ( -13.45809327831024405, 15.47793591600723850, -30.00000000000001421 ) ) ;
#7305=CARTESIAN_POINT ( 'NONE',  ( 16.84884541703955918, 18.74267451200035950, -12.76513676328720415 ) ) ;
#7307=CARTESIAN_POINT ( 'NONE',  ( 10.90692232337486445, 34.26194292751238635, -5.446513464750788458 ) ) ;
#7312=CARTESIAN_POINT ( 'NONE',  ( 10.07140245800056633, -18.11449741766177368, -27.41507013238322088 ) ) ;
#7316=CARTESIAN_POINT ( 'NONE',  ( -14.03908325169028615, 23.91319235039795643, -13.51416224689532086 ) ) ;
#7319=CARTESIAN_POINT ( 'NONE',  ( 10.79644714444348708, -20.53841121863572994, -20.58586955329300139 ) ) ;
#7324=CARTESIAN_POINT ( 'NONE',  ( -13.29693570674033687, 31.40254479259449383, -5.904557403147712158 ) ) ;
#7327=CARTESIAN_POINT ( 'NONE',  ( -34.97676071130810271, -8.686622228168268123, -7.176601743262130739 ) ) ;
#7331=CARTESIAN_POINT ( 'NONE',  ( 30.77433313779998159, 0.05499387012786746687, -5.946098457891356936 ) ) ;
#7335=CARTESIAN_POINT ( 'NONE',  ( -30.87810876133901061, -0.05119658576620297191, -5.945909103480649271 ) ) ;
#7338=CARTESIAN_POINT ( 'NONE',  ( 32.07230589051683722, -3.026076898309492336, -9.536960300404496493 ) ) ;
#7345=CARTESIAN_POINT ( 'NONE',  ( 0.000000000000000000, 0.000000000000000000, -30.00000000000000000 ) ) ;
#7356=CARTESIAN_POINT ( 'NONE',  ( -20.20854214045650110, 8.100511891533708209, -21.13395932336453598 ) ) ;
#7357=CARTESIAN_POINT ( 'NONE',  ( 20.75735356854552904, -27.05917745021801224, -6.795945968575883178 ) ) ;
#7359=EDGE_LOOP ( 'NONE', ( #8185, #25832, #31729, #9146, #13532 ) ) ;
#7360=CARTESIAN_POINT ( 'NONE',  ( 13.11120197629568196, 22.41587477055116295, -16.42154945907974195 ) ) ;
#7363=CARTESIAN_POINT ( 'NONE',  ( -11.99665585415270996, 16.62659876986841567, -29.36898932499439496 ) ) ;
#7366=CARTESIAN_POINT ( 'NONE',  ( 15.20579750689515919, 26.17738660362985570, -8.298505875400808307 ) ) ;
#7368=CARTESIAN_POINT ( 'NONE',  ( 18.30700033879082866, -10.10138274711125916, -26.96693921537031358 ) ) ;
#7370=VERTEX_POINT ( 'NONE', #29760 ) ;
#7371=CARTESIAN_POINT ( 'NONE',  ( -15.26147044535763619, 27.21892886845185089, -5.941221209073404452 ) ) ;
#7374=CARTESIAN_POINT ( 'NONE',  ( -10.36434502333254315, -19.11546864033186566, -23.83618939619293542 ) ) ;
#7379=CARTESIAN_POINT ( 'NONE',  ( -34.44723686885956226, -13.00661877071162209, -8.430185889806901756 ) ) ;
#7380=CARTESIAN_POINT ( 'NONE',  ( -13.46329895589916426, -25.24432993333344655, -10.67838853379888420 ) ) ;
#7381=DIRECTION ( 'NONE',  ( 0.000000000000000000, 0.000000000000000000, 1.000000000000000000 ) ) ;
#7382=CARTESIAN_POINT ( 'NONE',  ( 13.21519265033025370, 15.68751749194264811, -29.39041693340186256 ) ) ;
#7384=CARTESIAN_POINT ( 'NONE',  ( 28.17783618559230163, 2.888000139098982455, -5.949579471811276221 ) ) ;
#7388=CARTESIAN_POINT ( 'NONE',  ( -29.98028507518004915, -0.1513904216296562966, -9.695762027821260176 ) ) ;
#7389=CARTESIAN_POINT ( 'NONE',  ( 31.12761295898370406, -0.5681698218874843276, -7.338521178719154214 ) ) ;
#7392=VERTEX_POINT ( 'NONE', #21018 ) ;
#7393=CARTESIAN_POINT ( 'NONE',  ( -16.24796006241077961, 15.88921519459651499, -30.00000000000001421 ) ) ;
#7408=CARTESIAN_POINT ( 'NONE',  ( 28.16003781345056112, -24.46727846297508790, -6.718121626700479077 ) ) ;
#7411=CARTESIAN_POINT ( 'NONE',  ( 11.17633995497393151, 19.38694057465163922, -22.64794263314978906 ) ) ;
#7413=CARTESIAN_POINT ( 'NONE',  ( -14.43025776552523709, 14.57938852240508965, -29.40747009719811444 ) ) ;
#7415=CARTESIAN_POINT ( 'NONE',  ( 15.14062276522389361, -26.27454551934281213, -8.297974524426454224 ) ) ;
#7417=CARTESIAN_POINT ( 'NONE',  ( 15.24290316429634373, 26.37011248965962551, -7.827967277537388746 ) ) ;
#7419=CARTESIAN_POINT ( 'NONE',  ( 14.02760127444125438, 23.93997290703913805, -13.51284491737120064 ) ) ;
#7422=CARTESIAN_POINT ( 'NONE',  ( -15.33535238615493235, 26.80152092193110391, -6.415128186030386814 ) ) ;
#7424=CARTESIAN_POINT ( 'NONE',  ( -15.07294390951978791, -26.14423714609062799, -8.768195475925240956 ) ) ;
#7428=CARTESIAN_POINT ( 'NONE',  ( -28.05941199598445834, -18.14228187561381134, -12.89353790789255783 ) ) ;
#7429=CARTESIAN_POINT ( 'NONE',  ( -4.809173904559163937, -24.92317228705597287, -4.999999999999999112 ) ) ;
#7430=CARTESIAN_POINT ( 'NONE',  ( 15.89036220987575376, 24.93293676434921835, -6.419745934221619876 ) ) ;
#7432=CARTESIAN_POINT ( 'NONE',  ( 23.38135512150587658, 9.224932765178692762, -5.964625366264517226 ) ) ;
#7439=CARTESIAN_POINT ( 'NONE',  ( -20.43418187165424982, -1.772479648697218302, -30.00000000000000000 ) ) ;
#7445=DIRECTION ( 'NONE',  ( -0.000000000000000000, -0.000000000000000000, -1.000000000000000000 ) ) ;
#7446=CARTESIAN_POINT ( 'NONE',  ( 18.98852328848152382, -8.348878395094288862, -27.72209281211808118 ) ) ;
#7452=CIRCLE ( 'NONE', #36676, 61.99999999999998579 ) ;
#7455=CARTESIAN_POINT ( 'NONE',  ( -1.635714998051162938, 32.39290691969485891, -13.80806220344194024 ) ) ;
#7457=CYLINDRICAL_SURFACE ( 'NONE', #11149, 61.99999999999997868 ) ;
#7462=CARTESIAN_POINT ( 'NONE',  ( 9.616349836912345239, 18.28445365398381028, -27.99377830595204841 ) ) ;
#7463=CARTESIAN_POINT ( 'NONE',  ( 32.35383858704737037, -1.519079388893764149, -4.999999999999999112 ) ) ;
#7466=CARTESIAN_POINT ( 'NONE',  ( -17.92042771800729639, 12.70853344890674386, -20.10281234600826394 ) ) ;
#7470=CARTESIAN_POINT ( 'NONE',  ( 15.53190721697598242, -26.72795937246275599, -5.945400711064137589 ) ) ;
#7472=CARTESIAN_POINT ( 'NONE',  ( 10.96965864260556600, 17.37149835738324910, -28.70543893499321086 ) ) ;
#7473=CARTESIAN_POINT ( 'NONE',  ( -6.155076441694329326, 21.71698211341365337, -20.11584339644705111 ) ) ;
#7475=CARTESIAN_POINT ( 'NONE',  ( -15.56847894655029485, -14.60930148832306763, -25.70159151419933252 ) ) ;
#7476=CARTESIAN_POINT ( 'NONE',  ( 7.481479378253174772, -23.30152825933829774, -14.77492706919554522 ) ) ;
#7477=CARTESIAN_POINT ( 'NONE',  ( 13.87218762615114542, 23.17697767821096377, -14.48925779226203758 ) ) ;
#7478=CARTESIAN_POINT ( 'NONE',  ( 20.57095190365273396, 13.97674357447790250, -5.482604214182108748 ) ) ;
#7484=CARTESIAN_POINT ( 'NONE',  ( -9.379895652603979173, 35.46246444712465973, -5.443039496959672263 ) ) ;
#7486=CARTESIAN_POINT ( 'NONE',  ( -14.21183036229989938, -25.04515749559450555, -11.60314391679283297 ) ) ;
#7489=CARTESIAN_POINT ( 'NONE',  ( 20.48245044547724447, 0.8483310608570673317, -30.00000000000000000 ) ) ;
#7494=CARTESIAN_POINT ( 'NONE',  ( -20.48011438624494218, 0.9027161730473576284, -29.34916148302687589 ) ) ;
#7496=CARTESIAN_POINT ( 'NONE',  ( 20.09314088254942021, -4.111701498484372053, -29.26211593337953687 ) ) ;
#7511=CARTESIAN_POINT ( 'NONE',  ( 18.24376955283985424, 17.51282272560135667, -9.848228921199581265 ) ) ;
#7512=CARTESIAN_POINT ( 'NONE',  ( 7.361316653671116761, 22.88337532404381491, -20.99261860353674436 ) ) ;
#7516=CARTESIAN_POINT ( 'NONE',  ( 10.29754018676950622, -18.14354158297081909, -26.77788074137142615 ) ) ;
#7522=CARTESIAN_POINT ( 'NONE',  ( -11.70184164389253745, 18.89639632332092845, -22.73775843682962261 ) ) ;
#7525=CARTESIAN_POINT ( 'NONE',  ( 14.50550552640858015, -26.01656545232359363, -8.773312412628245127 ) ) ;
#7531=CARTESIAN_POINT ( 'NONE',  ( -13.26798563164391354, 31.32064769528049197, -6.352507814907438544 ) ) ;
#7532=CARTESIAN_POINT ( 'NONE',  ( -15.52303001916276592, -20.83641102679212764, -18.06021460390243405 ) ) ;
#7535=CARTESIAN_POINT ( 'NONE',  ( -22.66259745418890859, -5.598351139313090030, -22.08065378927834388 ) ) ;
#7538=CARTESIAN_POINT ( 'NONE',  ( 22.69409974816363729, 0.7326708127613092980, -21.63252463746919929 ) ) ;
#7545=CARTESIAN_POINT ( 'NONE',  ( -29.82034722167092156, 0.02361265341038061225, -9.708167889285391539 ) ) ;
#7548=CARTESIAN_POINT ( 'NONE',  ( 33.36633864933632054, -3.217268494394103229, -5.458641031229113594 ) ) ;
#7549=CARTESIAN_POINT ( 'NONE',  ( 17.25552743462859695, 11.08949724875112608, -29.99999999999998934 ) ) ;
#7558=CIRCLE ( 'NONE', #30279, 15.99999999999999645 ) ;
#7564=CARTESIAN_POINT ( 'NONE',  ( -22.44844293511189193, 8.669737220969816249, -12.85907312109028133 ) ) ;
#7565=CARTESIAN_POINT ( 'NONE',  ( 20.90254793926122900, -27.22588555765620555, -5.000000000000008882 ) ) ;
#7568=CARTESIAN_POINT ( 'NONE',  ( 11.59239201401879171, 19.00133579775832615, -22.71882842871296404 ) ) ;
#7570=CARTESIAN_POINT ( 'NONE',  ( -12.37225743350618146, 18.24419790101515204, -22.84300898652141854 ) ) ;
#7573=CARTESIAN_POINT ( 'NONE',  ( 13.52849422955318914, 22.74332991843149543, -15.45577255175012787 ) ) ;
#7575=CARTESIAN_POINT ( 'NONE',  ( 28.41128743669290557, -15.66287405488943740, -13.80598174040671466 ) ) ;
#7576=DIRECTION ( 'NONE',  ( 0.000000000000000000, 0.000000000000000000, 1.000000000000000000 ) ) ;
#7578=CARTESIAN_POINT ( 'NONE',  ( -10.81707015764707691, 17.67222468787956302, -27.42788574818700553 ) ) ;
#7580=CARTESIAN_POINT ( 'NONE',  ( -16.31051618889534893, -26.39850790843190254, -8.716711649698549280 ) ) ;
#7585=CARTESIAN_POINT ( 'NONE',  ( -34.18333301601428786, -12.90150185328116628, -8.870171403992342718 ) ) ;
#7586=CARTESIAN_POINT ( 'NONE',  ( -14.75944605622549943, -26.27728134964919349, -7.830481699696290931 ) ) ;
#7588=CARTESIAN_POINT ( 'NONE',  ( 15.94977354568814754, 20.60013326908762465, -12.70067996356593021 ) ) ;
#7590=CARTESIAN_POINT ( 'NONE',  ( 24.80460892327041833, 3.756148522752393859, -14.69522679569688250 ) ) ;
#7594=CARTESIAN_POINT ( 'NONE',  ( -22.78220600028421927, 0.4401612305667206293, -21.59410079891940626 ) ) ;
#7595=CARTESIAN_POINT ( 'NONE',  ( 29.97538051898516187, -0.6571090628178190007, -10.59662107009966547 ) ) ;
#7599=CARTESIAN_POINT ( 'NONE',  ( -22.77989339854785200, 2.034344915145157806, -20.71315197334980951 ) ) ;
#7600=CARTESIAN_POINT ( 'NONE',  ( -6.023418944065157987, 39.81932404830322270, -4.999999999999988454 ) ) ;
#7605=AXIS2_PLACEMENT_3D ( 'NONE', #998, #19675, #25767 ) ;
#7607=CARTESIAN_POINT ( 'NONE',  ( 19.48557158514975285, -11.24999999999995737, 6.000000000000000000 ) ) ;
#7612=CARTESIAN_POINT ( 'NONE',  ( 25.68472818303882121, -23.76469768826056850, -10.23310688448228944 ) ) ;
#7616=CARTESIAN_POINT ( 'NONE',  ( 14.49073764824685639, 26.09592138030880903, -10.60856989523508354 ) ) ;
#7620=CARTESIAN_POINT ( 'NONE',  ( -17.10053421514107086, 20.30440721539819648, -9.319735994576449301 ) ) ;
#7622=CARTESIAN_POINT ( 'NONE',  ( 15.37571132048090838, -26.71368809714059722, -5.000000000000000888 ) ) ;
#7624=CARTESIAN_POINT ( 'NONE',  ( 12.66461257586694522, 21.03697436711803093, -18.45420929576124180 ) ) ;
#7626=CARTESIAN_POINT ( 'NONE',  ( 14.02442048416569875, 23.94739483851058992, -13.51247984510621691 ) ) ;
#7628=CARTESIAN_POINT ( 'NONE',  ( -14.25168967311887336, 24.57581336903061597, -12.54168332028313770 ) ) ;
#7630=CARTESIAN_POINT ( 'NONE',  ( -9.962624055743289020, -18.81531389238340424, -25.01503139869100067 ) ) ;
#7633=CARTESIAN_POINT ( 'NONE',  ( -24.40043856705758429, -15.76608764628647386, -16.63189293991312923 ) ) ;
#7634=CARTESIAN_POINT ( 'NONE',  ( -5.781254241314485398, -22.30500674272131079, -17.88517324897596339 ) ) ;
#7635=CARTESIAN_POINT ( 'NONE',  ( 13.51725026480668213, 20.71157673340521654, -17.53186203222074724 ) ) ;
#7638=CARTESIAN_POINT ( 'NONE',  ( 18.90684236932249362, 8.006108384110648402, -28.85488273963430572 ) ) ;
#7639=CARTESIAN_POINT ( 'NONE',  ( 21.52603227935954777, -27.16584173104201483, -4.999999999999999112 ) ) ;
#7644=CARTESIAN_POINT ( 'NONE',  ( -27.39143991665605427, -1.197730116296394920, -15.28568366619224506 ) ) ;
#7654=CARTESIAN_POINT ( 'NONE',  ( 19.01366704504291150, -7.688495684904651739, -29.22164179442962606 ) ) ;
#7664=CARTESIAN_POINT ( 'NONE',  ( -0.6617914413177042876, 33.48614826591853699, -12.88875466627582611 ) ) ;
#7667=DIRECTION ( 'NONE',  ( 0.000000000000000000, 0.000000000000000000, 1.000000000000000000 ) ) ;
#7671=CARTESIAN_POINT ( 'NONE',  ( 12.77361610477846021, 26.39586754454798623, -13.30043833072773118 ) ) ;
#7673=AXIS2_PLACEMENT_3D ( 'NONE', #7794, #3738, #31974 ) ;
#7675=CARTESIAN_POINT ( 'NONE',  ( -17.80721512534418594, 11.54891248224037703, -23.32888160359681606 ) ) ;
#7678=CARTESIAN_POINT ( 'NONE',  ( 14.78531380799004857, -25.66241841546151647, -10.17861963493258592 ) ) ;
#7680=CARTESIAN_POINT ( 'NONE',  ( 14.27327873935064240, 24.51847890865961332, -12.54657257531869163 ) ) ;
#7682=CARTESIAN_POINT ( 'NONE',  ( -15.29245034862078256, 32.56469986091995850, -13.99876745781543441 ) ) ;
#7686=CARTESIAN_POINT ( 'NONE',  ( -15.00563708114499839, -14.08213718363703038, -28.49568921477004579 ) ) ;
#7687=CARTESIAN_POINT ( 'NONE',  ( 7.295766330847792247, -19.78656087607541281, -25.27750885764057287 ) ) ;
#7688=CARTESIAN_POINT ( 'NONE',  ( 13.07663108452908673, 21.41433421891530742, -17.46206790837113232 ) ) ;
#7689=EDGE_CURVE ( 'NONE', #39696, #20607, #21589, .T. ) ;
#7690=CARTESIAN_POINT ( 'NONE',  ( 21.09554553119179587, 13.00325820389446640, -5.483046721296032544 ) ) ;
#7692=EDGE_LOOP ( 'NONE', ( #7946, #983, #9218, #6840 ) ) ;
#7693=CARTESIAN_POINT ( 'NONE',  ( -6.113050074066779693, 35.28635442325187199, -9.759865422729246731 ) ) ;
#7700=CARTESIAN_POINT ( 'NONE',  ( -28.80451674142937435, 0.2040911148255387941, -11.60275554337247250 ) ) ;
#7702=CARTESIAN_POINT ( 'NONE',  ( 30.88881066025174249, -7.339856315056953129, -13.03470611699965254 ) ) ;
#7718=CARTESIAN_POINT ( 'NONE',  ( 18.46013033000776105, 17.79035490549923892, -7.894551517905889604 ) ) ;
#7719=CARTESIAN_POINT ( 'NONE',  ( 11.71220820147315500, 33.45731985618542836, -4.999999999999999112 ) ) ;
#7723=CARTESIAN_POINT ( 'NONE',  ( 14.59862030170441294, -25.11507782388870069, -11.58181169016334700 ) ) ;
#7724=FACE_OUTER_BOUND ( 'NONE', #6567, .T. ) ;
#7728=CARTESIAN_POINT ( 'NONE',  ( -14.83546796608161067, 25.62370260551899648, -10.17934226487036398 ) ) ;
#7730=CARTESIAN_POINT ( 'NONE',  ( 14.65009913602293246, -26.04841806957208306, -8.771861423863645868 ) ) ;
#7733=ORIENTED_EDGE ( 'NONE', *, *, #33684, .F. ) ;
#7735=CARTESIAN_POINT ( 'NONE',  ( -13.23903555654749020, 31.23875059796648301, -6.800458226667165818 ) ) ;
#7738=CARTESIAN_POINT ( 'NONE',  ( -33.89543892622803156, -8.375972393599855792, -9.375676559666750620 ) ) ;
#7741=CARTESIAN_POINT ( 'NONE',  ( 20.68287806670252849, 0.9940655047353081919, -27.45775483230204728 ) ) ;
#7746=CARTESIAN_POINT ( 'NONE',  ( -30.90411674721317326, -0.04211297212934855816, -5.474206011825583751 ) ) ;
#7749=CARTESIAN_POINT ( 'NONE',  ( 31.26306821908464428, -2.125275754412755624, -10.04085527566182634 ) ) ;
#7750=CARTESIAN_POINT ( 'NONE',  ( 18.28409177823415277, 9.297167255826021659, -29.99999999999998934 ) ) ;
#7759=VERTEX_POINT ( 'NONE', #2726 ) ;
#7762=AXIS2_PLACEMENT_3D ( 'NONE', #32043, #13753, #22692 ) ;
#7763=CARTESIAN_POINT ( 'NONE',  ( 5.000626697282971378, 37.74343557191168941, -4.999999999999998224 ) ) ;
#7768=CARTESIAN_POINT ( 'NONE',  ( 17.86928906486870616, -20.91001877870844439, -16.92124633107672338 ) ) ;
#7769=CARTESIAN_POINT ( 'NONE',  ( -75.15099915297791711, 43.38844959084113384, 0.000000000000000000 ) ) ;
#7770=CARTESIAN_POINT ( 'NONE',  ( -35.48538791413474769, -11.24999995268676933, -5.000000000000001776 ) ) ;
#7773=CARTESIAN_POINT ( 'NONE',  ( 12.58653840504220156, 21.15301265646719742, -18.43749620103639586 ) ) ;
#7775=CARTESIAN_POINT ( 'NONE',  ( -11.60488116879842835, 17.80579030430908816, -25.05364671859870640 ) ) ;
#7778=CARTESIAN_POINT ( 'NONE',  ( 15.45734228612143646, 26.63525802094401840, -5.000000000000000000 ) ) ;
#7780=CARTESIAN_POINT ( 'NONE',  ( 21.14049327140447687, -10.84634200327551312, -21.84289514537541166 ) ) ;
#7782=CARTESIAN_POINT ( 'NONE',  ( -15.18956287470529709, 27.28009750321776039, -6.407581706259474430 ) ) ;
#7784=CARTESIAN_POINT ( 'NONE',  ( -13.64508740925339758, -22.56256837047442687, -16.33802543730708123 ) ) ;
#7788=CARTESIAN_POINT ( 'NONE',  ( -35.01063367814790439, -14.47062566131834416, -6.283729949479822885 ) ) ;
#7789=CARTESIAN_POINT ( 'NONE',  ( -12.26719960628313899, -22.55384718030699176, -16.47309707856247485 ) ) ;
#7791=CARTESIAN_POINT ( 'NONE',  ( 17.28126569830730475, 21.10767333569910065, -5.476227410499634018 ) ) ;
#7793=CARTESIAN_POINT ( 'NONE',  ( 27.14291608416113988, 3.777963889476882109, -7.862006169886337048 ) ) ;
#7794=CARTESIAN_POINT ( 'NONE',  ( 19.48557158514988075, -11.24999999999998224, 0.000000000000000000 ) ) ;
#7800=CARTESIAN_POINT ( 'NONE',  ( -25.96849961500957349, 0.1468702090680218675, -16.42151745127020135 ) ) ;
#7801=CARTESIAN_POINT ( 'NONE',  ( 20.49250884496040115, 0.5553618484168653113, -30.00000000000000355 ) ) ;
#7804=CARTESIAN_POINT ( 'NONE',  ( -20.63698148512490604, 1.517229800946207297, -27.48967112051710160 ) ) ;
#7805=CARTESIAN_POINT ( 'NONE',  ( 3.091399026088761826, 22.35909668862748489, -30.00000000000000711 ) ) ;
#7814=CARTESIAN_POINT ( 'NONE',  ( -23.14161831312300066, 5.133065578429416576, -16.80419845731963946 ) ) ;
#7817=CARTESIAN_POINT ( 'NONE',  ( 18.61921750058829517, -17.17969631063009928, -19.77528146303147949 ) ) ;
#7818=CARTESIAN_POINT ( 'NONE',  ( 1.485571585149812135, -11.25000000000009415, 3.000000000000000000 ) ) ;
#7820=CARTESIAN_POINT ( 'NONE',  ( 14.68255685887305795, 26.08100846820239838, -10.15216213446657356 ) ) ;
#7822=CARTESIAN_POINT ( 'NONE',  ( -17.16552075097585117, 20.40790064679622873, -8.835065107039243415 ) ) ;
#7824=CARTESIAN_POINT ( 'NONE',  ( 11.11074582133875843, -20.48182189777266160, -20.55012700056129660 ) ) ;
#7826=CARTESIAN_POINT ( 'NONE',  ( 14.54328903961689790, 24.94079327997583917, -11.59986628730510105 ) ) ;
#7828=CARTESIAN_POINT ( 'NONE',  ( 11.47176157324268786, 18.44815111932139118, -23.85198228110581908 ) ) ;
#7829=ORIENTED_EDGE ( 'NONE', *, *, #20021, .F. ) ;
#7830=CARTESIAN_POINT ( 'NONE',  ( -15.25818811814006715, 26.64143884112164073, -7.354687272877148629 ) ) ;
#7832=CARTESIAN_POINT ( 'NONE',  ( -14.74254311150509622, -25.65307385468569734, -10.18114048116609460 ) ) ;
#7834=CARTESIAN_POINT ( 'NONE',  ( -31.94951466207645296, -20.64243727267584561, -7.119159330032495347 ) ) ;
#7835=CARTESIAN_POINT ( 'NONE',  ( -9.079790354755763460, -25.03302911735815073, -8.836781494452289110 ) ) ;
#7836=CARTESIAN_POINT ( 'NONE',  ( 15.81916445039664687, 24.79389647095221250, -7.365108267298476008 ) ) ;
#7838=CARTESIAN_POINT ( 'NONE',  ( 20.75988934644436767, 7.624137786315204224, -20.05700069588757728 ) ) ;
#7842=EDGE_CURVE ( 'NONE', #33096, #33201, #15789, .T. ) ;
#7845=CARTESIAN_POINT ( 'NONE',  ( -31.44789842147330106, -2.359368921698832722, -10.02552052183717635 ) ) ;
#7850=CARTESIAN_POINT ( 'NONE',  ( -3.485571585149855434, -11.25000000000002132, 6.000000000000000000 ) ) ;
#7851=CARTESIAN_POINT ( 'NONE',  ( 24.20165044650383734, -11.49403616741239809, -18.62786580867516051 ) ) ;
#7861=CARTESIAN_POINT ( 'NONE',  ( 0.2867187372796554667, 26.83502801510120506, -18.61248171148112363 ) ) ;
#7867=CARTESIAN_POINT ( 'NONE',  ( 9.427076569009681606, 18.67421965452293620, -26.67537954699011848 ) ) ;
#7871=CARTESIAN_POINT ( 'NONE',  ( -17.71759125216689412, 12.53367430966638985, -21.16048139840979658 ) ) ;
#7874=CARTESIAN_POINT ( 'NONE',  ( 9.640484335838371166, -18.33127209161421334, -27.44640424101937626 ) ) ;
#7876=CARTESIAN_POINT ( 'NONE',  ( 15.40208502184672135, 26.83309954512951023, -4.999999999999998224 ) ) ;
#7877=CARTESIAN_POINT ( 'NONE',  ( -22.40982762235195835, 2.618079236897030704, -21.24786896499725231 ) ) ;
#7879=CARTESIAN_POINT ( 'NONE',  ( -15.82313792508790584, -13.97225745301835964, -26.33890869513203370 ) ) ;
#7880=CARTESIAN_POINT ( 'NONE',  ( 5.143376291546045032, -22.33000100694908241, -17.91295319193513791 ) ) ;
#7881=CARTESIAN_POINT ( 'NONE',  ( 15.44311626412968508, 26.25345304022521375, -6.888681639014727409 ) ) ;
#7882=CARTESIAN_POINT ( 'NONE',  ( 19.51749221952617930, 13.16658399996466322, -13.89803554530751128 ) ) ;
#7886=CARTESIAN_POINT ( 'NONE',  ( -7.127291779580057884, 34.85034489748454689, -9.772412510442009648 ) ) ;
#7897=CARTESIAN_POINT ( 'NONE',  ( -23.25167227063256803, 0.7341704794712563542, -20.56396823476833902 ) ) ;
#7899=CARTESIAN_POINT ( 'NONE',  ( 34.05899686684449534, -10.24931931024947929, -9.342407649574157702 ) ) ;
#7911=EDGE_CURVE ( 'NONE', #31854, #16687, #4744, .T. ) ;
#7913=CARTESIAN_POINT ( 'NONE',  ( -16.72879317732252247, -11.86740072773090127, -30.00000000000002132 ) ) ;
#7916=CARTESIAN_POINT ( 'NONE',  ( 18.05890274853723199, 15.78661794053360801, -13.85158280915597473 ) ) ;
#7917=CARTESIAN_POINT ( 'NONE',  ( 10.15314824002201810, 31.60015277329938144, -11.20656053573065236 ) ) ;
#7921=CARTESIAN_POINT ( 'NONE',  ( 15.68476252645482205, -26.40036019609846107, -8.278550333207020273 ) ) ;
#7922=CARTESIAN_POINT ( 'NONE',  ( 31.47283671532267846, -25.12609584734865464, -5.000000000000008882 ) ) ;
#7925=CARTESIAN_POINT ( 'NONE',  ( -12.65206519043741551, 21.05528877957942768, -18.45198030644581877 ) ) ;
#7927=CARTESIAN_POINT ( 'NONE',  ( 12.73482621124554726, -24.80592790563511585, -11.64540342703255682 ) ) ;
#7929=ORIENTED_EDGE ( 'NONE', *, *, #264, .T. ) ;
#7931=CARTESIAN_POINT ( 'NONE',  ( -12.58732244184787774, 32.13884721240458475, -6.785466956703739783 ) ) ;
#7935=CARTESIAN_POINT ( 'NONE',  ( -20.17828169183510667, -3.673208557823401943, -29.26865376204499114 ) ) ;
#7938=CARTESIAN_POINT ( 'NONE',  ( 20.47879743316550005, 0.9320964914785052624, -30.00000000000000000 ) ) ;
#7944=CARTESIAN_POINT ( 'NONE',  ( -30.86643083211014016, -0.03928469928488562135, -5.946079256554607007 ) ) ;
#7946=ORIENTED_EDGE ( 'NONE', *, *, #24930, .T. ) ;
#7947=CARTESIAN_POINT ( 'NONE',  ( 31.76370184099492633, -4.744110583585224639, -11.28924081358098341 ) ) ;
#7959=CARTESIAN_POINT ( 'NONE',  ( 6.075063716662223001, 37.19263437435982667, -6.287285438531430515 ) ) ;
#7963=CARTESIAN_POINT ( 'NONE',  ( 14.22296627154594084, -18.85705313786432313, -21.18946184155140244 ) ) ;
#7969=CARTESIAN_POINT ( 'NONE',  ( 11.60819584869819288, 18.98628572600766518, -22.72157423742040905 ) ) ;
#7971=CARTESIAN_POINT ( 'NONE',  ( -15.43622781282135215, 26.27460386919110746, -6.888601964265022026 ) ) ;
#7974=CARTESIAN_POINT ( 'NONE',  ( 14.76676254508215713, 25.31098156848036851, -10.65510591171607579 ) ) ;
#7976=CARTESIAN_POINT ( 'NONE',  ( 31.77261430474117532, -21.49768664888851788, -4.999999999999999112 ) ) ;
#7978=CARTESIAN_POINT ( 'NONE',  ( -14.67061210956474326, 28.11310680807456208, -7.773254751785441563 ) ) ;
#7980=CARTESIAN_POINT ( 'NONE',  ( -16.71012240396724025, -26.29450614545289611, -9.160826647832207570 ) ) ;
#7984=CARTESIAN_POINT ( 'NONE',  ( -28.69690197025867562, -11.83258904652041643, -14.76511728228867604 ) ) ;
#7985=CARTESIAN_POINT ( 'NONE',  ( -14.45483107746191465, -26.00542429865824090, -8.773822038624603081 ) ) ;
#7987=CARTESIAN_POINT ( 'NONE',  ( 16.77170801253743448, 22.01473390083994275, -7.380717902106597172 ) ) ;
#7989=CARTESIAN_POINT ( 'NONE',  ( 20.54205287650563250, 2.405902401984270522, -27.54068107859523096 ) ) ;
#7995=CARTESIAN_POINT ( 'NONE',  ( -30.57520037393770451, -0.1065157518614621435, -7.823604440374101188 ) ) ;
#7996=CARTESIAN_POINT ( 'NONE',  ( 27.50873112917703978, -0.2858532659916371843, -14.41729497493959045 ) ) ;
#8001=CARTESIAN_POINT ( 'NONE',  ( -21.17204097405855023, 1.464915700757598360, -25.08531244034496055 ) ) ;
#8003=CARTESIAN_POINT ( 'NONE',  ( -16.84920187454419960, 29.09530251867925443, -13.79123840944734170 ) ) ;
#8013=CARTESIAN_POINT ( 'NONE',  ( -21.59735981781079417, 5.059875484007670288, -20.98042407182869340 ) ) ;
#8017=CARTESIAN_POINT ( 'NONE',  ( 26.32663925810967953, -25.71384748841218837, -4.999999999999998224 ) ) ;
#8019=CARTESIAN_POINT ( 'NONE',  ( -14.98890121934610242, -28.67928442654176635, 0.000000000000000000 ) ) ;
#8020=CARTESIAN_POINT ( 'NONE',  ( 15.30309001416959802, 27.17055420720160441, -4.999999999999999112 ) ) ;
#8024=CARTESIAN_POINT ( 'NONE',  ( -16.25978453391780221, 22.36894860302335886, -9.288381802591871406 ) ) ;
#8026=CARTESIAN_POINT ( 'NONE',  ( 15.21665703708782935, -26.47879611614396111, -7.358218835048320194 ) ) ;
#8028=CARTESIAN_POINT ( 'NONE',  ( 12.40183761314701449, 20.47613423964896029, -19.49836111761218405 ) ) ;
#8032=CARTESIAN_POINT ( 'NONE',  ( -13.41058178396609080, 22.98005122180817139, -15.43185508673824735 ) ) ;
#8034=CARTESIAN_POINT ( 'NONE',  ( -15.44635164275937811, -26.65726164833965228, -6.416678024205798359 ) ) ;
#8036=CARTESIAN_POINT ( 'NONE',  ( -17.29914876638407861, -11.16020024788362974, -28.44682971825362827 ) ) ;
#8037=CARTESIAN_POINT ( 'NONE',  ( -6.226074173696266811, -19.80104272504923557, -27.05930787988562258 ) ) ;
#8038=CARTESIAN_POINT ( 'NONE',  ( 15.49015922161475167, 24.15577049684528887, -9.735419282224947679 ) ) ;
#8040=CARTESIAN_POINT ( 'NONE',  ( 23.97835192852010167, 8.298819924180955709, -6.446434780486328009 ) ) ;
#8045=CARTESIAN_POINT ( 'NONE',  ( -32.30815150485408793, -1.680769291408187316, -5.000000000000000000 ) ) ;
#8047=STYLED_ITEM ( 'NONE', ( #31 ), #9362 ) ;
#8050=CARTESIAN_POINT ( 'NONE',  ( -11.01950087092618524, 17.43848460801469002, -28.07618716959215277 ) ) ;
#8054=CARTESIAN_POINT ( 'NONE',  ( 19.35680011505175457, -9.211710752562881410, -25.58994971620333558 ) ) ;
#8062=CARTESIAN_POINT ( 'NONE',  ( 0.4110586764534028270, 38.44431916748334288, -5.855741157794193796 ) ) ;
#8071=CARTESIAN_POINT ( 'NONE',  ( 9.903829054754655914, 18.12412366152800658, -28.01031554129876966 ) ) ;
#8074=CARTESIAN_POINT ( 'NONE',  ( -16.91598364292035939, 12.90154645153827140, -23.29995136833793268 ) ) ;
#8077=CARTESIAN_POINT ( 'NONE',  ( 14.88972759991149530, -25.83697725034997461, -9.708168427115946741 ) ) ;
#8078=DIRECTION ( 'NONE',  ( -0.000000000000000000, -0.000000000000000000, -1.000000000000000000 ) ) ;
#8079=CARTESIAN_POINT ( 'NONE',  ( 15.38794517075334056, 26.79091751018437861, -5.945654618937589397 ) ) ;
#8083=CARTESIAN_POINT ( 'NONE',  ( -17.65121957807252784, -15.59521983380484222, -21.96053948915082188 ) ) ;
#8084=CARTESIAN_POINT ( 'NONE',  ( 4.234769651857060779, -20.16607359150837553, -27.68998930902958122 ) ) ;
#8085=CARTESIAN_POINT ( 'NONE',  ( 14.85392080762270339, 25.05954230463082766, -10.66070852731747998 ) ) ;
#8086=CARTESIAN_POINT ( 'NONE',  ( 17.99011237037677802, 13.10895772829668182, -19.04357418431120763 ) ) ;
#8089=CARTESIAN_POINT ( 'NONE',  ( -6.361647429086256800, 31.06932854847694969, -13.87644038312246764 ) ) ;
#8093=VERTEX_POINT ( 'NONE', #1362 ) ;
#8097=CARTESIAN_POINT ( 'NONE',  ( -29.61458559055934714, 0.2518799484168193770, -9.713275453577335128 ) ) ;
#8099=CARTESIAN_POINT ( 'NONE',  ( 28.16713897950105405, -8.472997818002736992, -15.79648965232683544 ) ) ;
#8108=VECTOR ( 'NONE', #20872, 1000.000000000000000 ) ;
#8116=CARTESIAN_POINT ( 'NONE',  ( 14.85614242573017840, 14.30966537380568759, -27.67306061729238209 ) ) ;
#8117=CARTESIAN_POINT ( 'NONE',  ( 8.359857552323353147, 21.45424803955862458, -22.25965238277191460 ) ) ;
#8121=CARTESIAN_POINT ( 'NONE',  ( 13.23316282574661251, -23.10607048933782082, -15.42806814948440497 ) ) ;
#8126=CARTESIAN_POINT ( 'NONE',  ( -11.47830338918615745, 18.44249444189321707, -23.85302490474181880 ) ) ;
#8128=CARTESIAN_POINT ( 'NONE',  ( 11.58858825903818257, -23.03010094018678089, -15.54224781274825595 ) ) ;
#8132=CARTESIAN_POINT ( 'NONE',  ( -11.75129741676435380, 32.67431248936103572, -7.653645928010829103 ) ) ;
#8138=CARTESIAN_POINT ( 'NONE',  ( -33.33009440080085284, -5.279162264021511675, -9.006299637744488606 ) ) ;
#8142=CARTESIAN_POINT ( 'NONE',  ( 28.81778564524760000, 0.1882255715981525357, -11.60218017744097807 ) ) ;
#8148=CARTESIAN_POINT ( 'NONE',  ( -23.31383330372760909, 0.5610641285874745643, -20.54315880825037510 ) ) ;
#8151=CARTESIAN_POINT ( 'NONE',  ( 20.68113486913782850, -2.268168025704259794, -27.24842174564768982 ) ) ;
#8167=CARTESIAN_POINT ( 'NONE',  ( 4.527020475796621923, 33.83005428846027485, -11.99704615662030527 ) ) ;
#8172=CARTESIAN_POINT ( 'NONE',  ( 17.86692456966301989, -23.49199618837229764, -14.12595633806949103 ) ) ;
#8177=CARTESIAN_POINT ( 'NONE',  ( 11.83320386989883488, 19.44516747061696904, -21.60573074431047402 ) ) ;
#8178=ORIENTED_EDGE ( 'NONE', *, *, #25883, .F. ) ;
#8179=CARTESIAN_POINT ( 'NONE',  ( -12.78688490849339487, 19.97022096780329292, -19.56400173231042317 ) ) ;
#8182=CARTESIAN_POINT ( 'NONE',  ( 14.99150837520656410, 25.62483198016352759, -9.711665107101897121 ) ) ;
#8184=CARTESIAN_POINT ( 'NONE',  ( 32.47636040670842306, -20.57534817285772277, -5.855945076690642459 ) ) ;
#8185=ORIENTED_EDGE ( 'NONE', *, *, #485, .T. ) ;
#8186=CARTESIAN_POINT ( 'NONE',  ( -14.50613712064790306, 26.05512619081983772, -10.61110433390421015 ) ) ;
#8188=CARTESIAN_POINT ( 'NONE',  ( -18.34279529041538126, -27.21360250413895443, -5.919932557224159453 ) ) ;
#8192=CARTESIAN_POINT ( 'NONE',  ( -35.12294622822932411, -10.95518361376287508, -7.153933696636912032 ) ) ;
#8193=CARTESIAN_POINT ( 'NONE',  ( -14.01793117240702458, -25.34536848690236255, -10.66627488844276073 ) ) ;
#8196=CARTESIAN_POINT ( 'NONE',  ( 27.89362309832364417, 2.032256754323124248, -10.22863755220655513 ) ) ;
#8197=EDGE_CURVE ( 'NONE', #15130, #16687, #35696, .T. ) ;
#8202=CARTESIAN_POINT ( 'NONE',  ( -20.61417483570997433, 0.7840236751464569886, -28.07419235526585055 ) ) ;
#8204=CARTESIAN_POINT ( 'NONE',  ( 28.39197557152373363, -0.7107394051037417837, -13.42105332491729541 ) ) ;
#8209=CARTESIAN_POINT ( 'NONE',  ( -29.17914473192155711, 1.735411910516140299, -5.947304834939044049 ) ) ;
#8210=CARTESIAN_POINT ( 'NONE',  ( -22.45323650136969462, -2.382502413133420038, -20.55760979252980647 ) ) ;
#8217=CARTESIAN_POINT ( 'NONE',  ( -25.87260067993565116, 5.291969182969162411, -8.360226650860235864 ) ) ;
#8220=CARTESIAN_POINT ( 'NONE',  ( 25.59259726831772497, -25.05938252355970519, -8.471152770727268688 ) ) ;
#8224=CARTESIAN_POINT ( 'NONE',  ( 13.58448792996048304, 23.80199789373500963, -14.43409159148844090 ) ) ;
#8228=CARTESIAN_POINT ( 'NONE',  ( -14.12254998924808191, 16.91766681099430869, -21.95434448082308521 ) ) ;
#8232=CARTESIAN_POINT ( 'NONE',  ( 11.31505853063862688, 18.03411298331075940, -25.01525395742355329 ) ) ;
#8233=EDGE_LOOP ( 'NONE', ( #37688, #35872, #22461, #22940, #21321, #26863, #13635 ) ) ;
#8234=CARTESIAN_POINT ( 'NONE',  ( 13.20924685295718248, 22.23599012058754099, -16.44404666642639867 ) ) ;
#8236=CARTESIAN_POINT ( 'NONE',  ( -10.92267213224567968, 17.34778819946280493, -29.99999999999998934 ) ) ;
#8238=CARTESIAN_POINT ( 'NONE',  ( -15.55120232977052552, -26.73296669180702878, -5.945196455431404736 ) ) ;
#8240=CARTESIAN_POINT ( 'NONE',  ( -23.40264495275803469, -13.17898732060409372, -18.60987684574479673 ) ) ;
#8241=CARTESIAN_POINT ( 'NONE',  ( -9.241023740148470722, -25.33547218322737038, -6.910767586270462282 ) ) ;
#8243=CARTESIAN_POINT ( 'NONE',  ( 13.92769306801763207, 21.97374865699145019, -15.51183746870685809 ) ) ;
#8245=CARTESIAN_POINT ( 'NONE',  ( 24.57025407321291510, 7.375674204439781612, -6.926099335226528098 ) ) ;
#8246=CARTESIAN_POINT ( 'NONE',  ( 15.48853125999101898, -26.74269726803731828, -5.000000000000000000 ) ) ;
#8250=CARTESIAN_POINT ( 'NONE',  ( -31.84661580973198625, -1.628238131297263358, -7.766091669641889794 ) ) ;
#8251=CARTESIAN_POINT ( 'NONE',  ( 29.73426277082694114, -0.1029795250634506915, -10.16860317180123374 ) ) ;
#8266=CARTESIAN_POINT ( 'NONE',  ( 0.4001783121710071889, 37.17016172131723550, -8.843365538038478135 ) ) ;
#8275=CARTESIAN_POINT ( 'NONE',  ( 13.79182622341905962, 26.77182061978390237, -11.47104827624631262 ) ) ;
#8278=CARTESIAN_POINT ( 'NONE',  ( -16.38814671032943693, 12.36958133795433135, -28.85484690269119668 ) ) ;
#8282=CARTESIAN_POINT ( 'NONE',  ( 14.37655681973246402, -25.07404765674405667, -11.59782526845664918 ) ) ;
#8285=CARTESIAN_POINT ( 'NONE',  ( 14.01431933016365150, 23.97271075189374656, -13.50973434947982099 ) ) ;
#8290=CARTESIAN_POINT ( 'NONE',  ( -21.37336528869494146, -18.93283188275981743, -16.72296912899527399 ) ) ;
#8291=CARTESIAN_POINT ( 'NONE',  ( 3.641758806176171870, -23.49846102025998817, -13.88050724111706913 ) ) ;
#8292=CARTESIAN_POINT ( 'NONE',  ( 11.35670081024726663, 17.63068499975756964, -26.24312638122347607 ) ) ;
#8293=CARTESIAN_POINT ( 'NONE',  ( 19.13565567046500959, 11.72986290071136217, -18.01978235670257789 ) ) ;
#8297=CARTESIAN_POINT ( 'NONE',  ( -4.675295383163502017, 19.96902330696676131, -29.99999999999998579 ) ) ;
#8305=EDGE_CURVE ( 'NONE', #13116, #34935, #14486, .T. ) ;
#8310=ORIENTED_EDGE ( 'NONE', *, *, #2798, .T. ) ;
#8311=CARTESIAN_POINT ( 'NONE',  ( -22.67633955519294631, 0.7916079257996353480, -21.63973890270278844 ) ) ;
#8313=CARTESIAN_POINT ( 'NONE',  ( 19.63120307387857011, -5.935663759831211195, -29.23833046634263511 ) ) ;
#8322=ORIENTED_EDGE ( 'NONE', *, *, #12343, .T. ) ;
#8328=CARTESIAN_POINT ( 'NONE',  ( 18.09980013376456398, 17.32878008101015155, -10.83467271882861560 ) ) ;
#8330=CARTESIAN_POINT ( 'NONE',  ( 8.579543980086729249, 24.19985443805853720, -18.94540614325930150 ) ) ;
#8331=EDGE_LOOP ( 'NONE', ( #38796, #35257, #3165, #2657 ) ) ;
#8332=CARTESIAN_POINT ( 'NONE',  ( -18.81000520956799704, 8.529488778487996470, -27.16704582425938597 ) ) ;
#8335=CARTESIAN_POINT ( 'NONE',  ( 11.36210984317571615, -20.43702075986949040, -20.51812109925986150 ) ) ;
#8338=CARTESIAN_POINT ( 'NONE',  ( -11.03706680401473506, 17.42694036731077745, -28.07723557321667585 ) ) ;
#8340=CARTESIAN_POINT ( 'NONE',  ( 12.47139895626693828, -24.39478734073985677, -12.60803247688938988 ) ) ;
#8344=CARTESIAN_POINT ( 'NONE',  ( -9.986907921862322013, 27.50688179610501294, -14.99363465816162666 ) ) ;
#8351=CARTESIAN_POINT ( 'NONE',  ( 20.52348880615194915, 0.9275646289840523417, -28.70940543212687501 ) ) ;
#8358=CARTESIAN_POINT ( 'NONE',  ( -25.20077581846105375, 0.3984468658264971319, -17.44060062697873192 ) ) ;
#8361=CARTESIAN_POINT ( 'NONE',  ( 33.54902081565550276, -4.132526625222229910, -7.247087903461005176 ) ) ;
#8374=CARTESIAN_POINT ( 'NONE',  ( 3.888268390277564546, 20.12764833916413210, -30.00000000000000000 ) ) ;
#8379=CARTESIAN_POINT ( 'NONE',  ( 19.58288088771594815, -26.98521917108113399, -7.262093437065574975 ) ) ;
#8385=CARTESIAN_POINT ( 'NONE',  ( 15.12690670045320651, 26.44130067926909788, -8.291666083221429062 ) ) ;
#8387=CARTESIAN_POINT ( 'NONE',  ( -15.59869368156687486, 26.13660472685725722, -5.000000000000000000 ) ) ;
#8391=CARTESIAN_POINT ( 'NONE',  ( 11.97503790938721657, 19.29424847012439059, -21.63139525819087439 ) ) ;
#8393=CARTESIAN_POINT ( 'NONE',  ( 19.66064036848656826, -11.63052904784041353, -22.98217444469445425 ) ) ;
#8395=CARTESIAN_POINT ( 'NONE',  ( -10.86333472933958433, 17.98415157847645318, -26.19019042869090086 ) ) ;
#8397=CARTESIAN_POINT ( 'NONE',  ( -17.29263770120802945, -27.09866115540251030, -4.999999999999999112 ) ) ;
#8400=CARTESIAN_POINT ( 'NONE',  ( -19.17275462598830060, -7.282501898908932958, -30.00000000000000711 ) ) ;
#8401=CARTESIAN_POINT ( 'NONE',  ( -14.98552525403816027, -26.61491965241963342, -5.474092641348948796 ) ) ;
#8404=CARTESIAN_POINT ( 'NONE',  ( 28.07054727141038697, 2.026488101130145658, -9.749946147146546949 ) ) ;
#8410=CARTESIAN_POINT ( 'NONE',  ( -20.69840430391611008, 0.7747587285446246863, -27.44368215450492698 ) ) ;
#8413=CARTESIAN_POINT ( 'NONE',  ( 20.54837291512225406, 0.2170867354722968989, -28.68434330076379979 ) ) ;
#8416=CARTESIAN_POINT ( 'NONE',  ( -27.64268375266474109, 3.518380400506786909, -5.950924345792210524 ) ) ;
#8426=CARTESIAN_POINT ( 'NONE',  ( -24.98617032440317942, 5.239009436875295300, -11.77689850835809793 ) ) ;
#8429=CARTESIAN_POINT ( 'NONE',  ( 20.86948450591783555, -20.46856481552917373, -15.82250207514942986 ) ) ;
#8432=CARTESIAN_POINT ( 'NONE',  ( 15.13840818345982520, 27.03333146816605748, -7.344069862628868073 ) ) ;
#8436=CARTESIAN_POINT ( 'NONE',  ( -16.52923656195466151, 22.85177225473215756, -6.899933075074482502 ) ) ;
#8439=CARTESIAN_POINT ( 'NONE',  ( 11.00415319253780488, 17.29620292487934563, -30.00000000000001421 ) ) ;
#8444=CARTESIAN_POINT ( 'NONE',  ( -13.43406490775605278, 22.93255246805462733, -15.43730422837821159 ) ) ;
#8446=CARTESIAN_POINT ( 'NONE',  ( -14.43849888084333877, -25.08593691932569314, -11.59330415005311643 ) ) ;
#8448=CARTESIAN_POINT ( 'NONE',  ( -31.87643534942240819, -17.94561782331171784, -9.724772667764392864 ) ) ;
#8449=CARTESIAN_POINT ( 'NONE',  ( -6.368927712313042555, -20.05147684786715701, -25.34049200730608220 ) ) ;
#8451=CARTESIAN_POINT ( 'NONE',  ( 12.55804699249790168, 17.47949508554678388, -24.00749146857737770 ) ) ;
#8453=CARTESIAN_POINT ( 'NONE',  ( 19.58333117617996777, 6.632644045549831446, -27.12887243873458942 ) ) ;
#8458=CARTESIAN_POINT ( 'NONE',  ( -31.33630356776520642, -0.7993948758031136359, -7.330644645363229017 ) ) ;
#8459=CARTESIAN_POINT ( 'NONE',  ( 20.69783600767029696, 0.7831999650737890839, -27.44422954938529813 ) ) ;
#8463=CARTESIAN_POINT ( 'NONE',  ( 22.52744239175980923, -0.1803094636422790109, -20.90349153981001606 ) ) ;
#8464=DIRECTION ( 'NONE',  ( 1.000000000000000000, 0.000000000000000000, 0.000000000000000000 ) ) ;
#8468=CARTESIAN_POINT ( 'NONE',  ( 0.000000000000000000, 22.50000000000000355, 0.000000000000000000 ) ) ;
#8471=CARTESIAN_POINT ( 'NONE',  ( 0.3940515309154056234, 36.53847938540027229, -9.725803077370580141 ) ) ;
#8474=CARTESIAN_POINT ( 'NONE',  ( -19.48557158514988785, -11.24999999999987743, 10.00000000000000000 ) ) ;
#8478=CARTESIAN_POINT ( 'NONE',  ( 14.41393829650433211, 27.23447492386241819, -9.633712356753633799 ) ) ;
#8482=CARTESIAN_POINT ( 'NONE',  ( -16.60583435348276282, 13.74075903883709593, -22.18912786978531315 ) ) ;
#8486=CARTESIAN_POINT ( 'NONE',  ( 10.25084136881418573, -19.15538197628319139, -23.85068623870123972 ) ) ;
#8487=DIRECTION ( 'NONE',  ( 0.000000000000000000, 0.000000000000000000, 1.000000000000000000 ) ) ;
#8488=CARTESIAN_POINT ( 'NONE',  ( 15.39020460041367855, 26.78288689686343105, -5.945739410967055605 ) ) ;
#8491=CARTESIAN_POINT ( 'NONE',  ( -29.08184185256072141, -22.79149011935838587, -8.424513042702869825 ) ) ;
#8492=CARTESIAN_POINT ( 'NONE',  ( 1.817969461173305712, -24.76413945269762351, -5.000000000000001776 ) ) ;
#8493=CARTESIAN_POINT ( 'NONE',  ( 15.34008105399866828, 26.04368486401110871, -7.829779149383753634 ) ) ;
#8494=CARTESIAN_POINT ( 'NONE',  ( 18.01512450864053250, 10.08994624255825912, -27.17860653033931939 ) ) ;
#8498=CARTESIAN_POINT ( 'NONE',  ( -4.693749193973906664, 20.04595565361518084, -28.49495074315137799 ) ) ;
#8505=CARTESIAN_POINT ( 'NONE',  ( -25.74458659788053083, 0.5194498575017915121, -16.46142640285149028 ) ) ;
#8506=CARTESIAN_POINT ( 'NONE',  ( 25.05526511386589306, -8.388987150351875144, -18.72753401343204160 ) ) ;
#8522=CARTESIAN_POINT ( 'NONE',  ( 18.90535999708258075, 15.28347868722541669, -11.85787095818008297 ) ) ;
#8523=CARTESIAN_POINT ( 'NONE',  ( 11.20956939700582211, 31.79909661247546637, -9.876575786099936138 ) ) ;
#8525=CARTESIAN_POINT ( 'NONE',  ( -20.61860813537857240, 9.113149517100110231, -17.99812580813538432 ) ) ;
#8530=CARTESIAN_POINT ( 'NONE',  ( 9.922609748437189126, -18.19104734674453994, -27.42597713094579248 ) ) ;
#8532=CARTESIAN_POINT ( 'NONE',  ( 21.88444403592372112, 6.126538576424477966, -21.50719306941230613 ) ) ;
#8533=CARTESIAN_POINT ( 'NONE',  ( -13.76553621605945210, 23.40493025121552506, -14.47534936899553948 ) ) ;
#8535=CARTESIAN_POINT ( 'NONE',  ( -13.33966701959958456, -16.00384814976887426, -27.17537271300066237 ) ) ;
#8536=CARTESIAN_POINT ( 'NONE',  ( 13.73668809508641608, -25.59735168978018294, -9.726329721036846010 ) ) ;
#8538=ORIENTED_EDGE ( 'NONE', *, *, #19001, .T. ) ;
#8541=CARTESIAN_POINT ( 'NONE',  ( -11.89071426873642778, 33.14490429473632105, -5.891362697687537953 ) ) ;
#8546=CARTESIAN_POINT ( 'NONE',  ( 29.28231774309053748, 0.1570984678961929726, -10.65577805818864121 ) ) ;
#8550=VERTEX_POINT ( 'NONE', #35508 ) ;
#8551=CARTESIAN_POINT ( 'NONE',  ( -24.55370900864287975, 0.4434148628449753882, -18.45356317131482982 ) ) ;
#8555=CARTESIAN_POINT ( 'NONE',  ( 34.73099849614892065, -6.268898363069737911, -5.000000000000007994 ) ) ;
#8566=CARTESIAN_POINT ( 'NONE',  ( 6.086784706011969526, 31.15961814524406037, -13.87178128487113327 ) ) ;
#8571=CARTESIAN_POINT ( 'NONE',  ( 11.74422086145278499, -16.80344316252863734, -29.30034920398468046 ) ) ;
#8574=FACE_OUTER_BOUND ( 'NONE', #9955, .T. ) ;
#8576=CARTESIAN_POINT ( 'NONE',  ( 14.69914344428350539, 25.51220288795486368, -10.64560462785820327 ) ) ;
#8578=CARTESIAN_POINT ( 'NONE',  ( -15.27513262873028665, 25.94661827369742113, -8.300200833134605105 ) ) ;
#8583=CARTESIAN_POINT ( 'NONE',  ( 11.76965676669902727, 18.83126597396366009, -22.74873947259427709 ) ) ;
#8585=CARTESIAN_POINT ( 'NONE',  ( 18.00492286382134566, -10.65055271466412812, -26.96479788887356221 ) ) ;
#8587=CARTESIAN_POINT ( 'NONE',  ( -15.19527047305266443, 27.50996873332976378, -5.000000000000001776 ) ) ;
#8589=CARTESIAN_POINT ( 'NONE',  ( -16.60262275586455161, -24.86345949671113331, -12.36567362711010354 ) ) ;
#8592=CARTESIAN_POINT ( 'NONE',  ( -34.03066577109931501, -11.68171929586705815, -9.322546398942927581 ) ) ;
#8594=CARTESIAN_POINT ( 'NONE',  ( -9.947661678533670226, -19.26027892739813652, -23.88733551178417613 ) ) ;
#8598=CARTESIAN_POINT ( 'NONE',  ( 21.57580026240890447, 3.046887179118514588, -22.98849545702982766 ) ) ;
#8599=B_SPLINE_CURVE_WITH_KNOTS ( 'NONE', 3,
 ( #37641, #6348, #3904, #15904, #7147 ),
 .UNSPECIFIED., .F., .F.,
 ( 4, 1, 4 ),
 ( 0.000000000000000000, 0.1250000000212990459, 0.1282122296533009798 ),
 .UNSPECIFIED. ) ;
#8603=CARTESIAN_POINT ( 'NONE',  ( -27.79845905001932849, 0.1112929649325302972, -13.50539263835538506 ) ) ;
#8606=CARTESIAN_POINT ( 'NONE',  ( 20.64185622598208170, 0.04121980942568206213, -28.03684029888757578 ) ) ;
#8611=CARTESIAN_POINT ( 'NONE',  ( -20.33969889556806265, 2.904538857774676686, -28.77042324836267895 ) ) ;
#8612=CYLINDRICAL_SURFACE ( 'NONE', #5765, 17.00000000000000000 ) ;
#8618=SHAPE_REPRESENTATION ( 'Detachable Washable Trimmer Head Cap', ( #24238 ), #9333 ) ;
#8621=ORIENTED_EDGE ( 'NONE', *, *, #17470, .T. ) ;
#8622=CARTESIAN_POINT ( 'NONE',  ( -20.18459099282218006, 5.011188685773205975, -26.50361906614367058 ) ) ;
#8625=CARTESIAN_POINT ( 'NONE',  ( 24.39459500260992542, -25.35271717551619020, -8.931748512371612492 ) ) ;
#8629=CARTESIAN_POINT ( 'NONE',  ( 15.30309001416959802, 27.17055420720160441, -5.472318710501133943 ) ) ;
#8633=CARTESIAN_POINT ( 'NONE',  ( -13.81191689907480047, 17.90740787171185389, -20.81067546043863103 ) ) ;
#8636=CARTESIAN_POINT ( 'NONE',  ( 15.41225152681027311, 26.70409590730232452, -5.946085469612699015 ) ) ;
#8640=CARTESIAN_POINT ( 'NONE',  ( -15.29484476591128228, 26.76856196483461048, -6.884705497639315830 ) ) ;
#8642=CARTESIAN_POINT ( 'NONE',  ( -10.02177213464359617, -18.79137684907821537, -25.00808960492178912 ) ) ;
#8645=CARTESIAN_POINT ( 'NONE',  ( -18.68643025256734447, -10.52603743360108268, -25.57491845876295500 ) ) ;
#8646=CARTESIAN_POINT ( 'NONE',  ( -11.46238439996275638, -22.55099105456122999, -16.53223957159231716 ) ) ;
#8648=CARTESIAN_POINT ( 'NONE',  ( 15.75550723163302713, 23.75836650642312975, -9.268051056800263865 ) ) ;
#8650=CARTESIAN_POINT ( 'NONE',  ( 21.17479613538668914, 6.043406367430672610, -21.04370527317109918 ) ) ;
#8655=CARTESIAN_POINT ( 'NONE',  ( -31.44678074335321938, -0.8094497182387121459, -6.866296305381922593 ) ) ;
#8658=CARTESIAN_POINT ( 'NONE',  ( 29.02264181254402686, -0.05255188267202027391, -11.58473844147850684 ) ) ;
#8663=CARTESIAN_POINT ( 'NONE',  ( 16.24796006241085422, 15.88921519459651144, -21.50719306941225639 ) ) ;
#8666=( GEOMETRIC_REPRESENTATION_CONTEXT ( 3 ) GLOBAL_UNCERTAINTY_ASSIGNED_CONTEXT ( ( #26635 ) ) GLOBAL_UNIT_ASSIGNED_CONTEXT ( ( #35352, #16873, #10167 ) ) REPRESENTATION_CONTEXT ( 'NONE', 'WORKASPACE' ) );
#8672=CARTESIAN_POINT ( 'NONE',  ( 1.558973647184125122, 37.87412607290816169, -7.545089284928025108 ) ) ;
#8681=CARTESIAN_POINT ( 'NONE',  ( 14.31634612938960593, 27.02271693021451782, -10.09916008547401489 ) ) ;
#8683=ORIENTED_EDGE ( 'NONE', *, *, #115, .F. ) ;
#8684=CARTESIAN_POINT ( 'NONE',  ( -18.97573237204982277, 16.39359448400360009, -8.880896986686993344 ) ) ;
#8688=CARTESIAN_POINT ( 'NONE',  ( 11.19426416879276687, -20.46679275895131767, -20.54027932467983319 ) ) ;
#8689=CARTESIAN_POINT ( 'NONE',  ( 14.02760127444122951, 23.93997290703920910, -13.51284491737118465 ) ) ;
#8690=CARTESIAN_POINT ( 'NONE',  ( 12.37672620654822175, 20.50964447495777421, -19.49331178464071002 ) ) ;
#8695=CARTESIAN_POINT ( 'NONE',  ( -15.77773026942784185, -13.10308996503666101, -30.00000000000001066 ) ) ;
#8696=CARTESIAN_POINT ( 'NONE',  ( 4.764572365127394349, -21.41444608039761022, -21.06969765009909423 ) ) ;
#8697=CARTESIAN_POINT ( 'NONE',  ( 11.58080580526187298, 17.82453155642948772, -25.05040652983576166 ) ) ;
#8698=CARTESIAN_POINT ( 'NONE',  ( 17.56107106814955898, 10.70378322536777205, -28.30016637139251756 ) ) ;
#8700=CARTESIAN_POINT ( 'NONE',  ( -3.610436583610349359, 21.08180157035248214, -25.64550946592787284 ) ) ;
#8708=CARTESIAN_POINT ( 'NONE',  ( -23.85997367143794889, 0.6784800307181348966, -19.51840897779039352 ) ) ;
#8710=CARTESIAN_POINT ( 'NONE',  ( 35.29110269690040269, -10.66697437443527008, -6.728013520106306267 ) ) ;
#8714=ORIENTED_EDGE ( 'NONE', *, *, #21810, .T. ) ;
#8724=CARTESIAN_POINT ( 'NONE',  ( 28.33613644512890772, -21.83622121967587759, -10.19242865772655549 ) ) ;
#8725=CARTESIAN_POINT ( 'NONE',  ( 19.98855543418123659, 14.89803298009520383, -6.936588910547434317 ) ) ;
#8726=CARTESIAN_POINT ( 'NONE',  ( 12.06095707006059037, 31.48640300589477548, -9.007870101607295510 ) ) ;
#8729=CARTESIAN_POINT ( 'NONE',  ( -18.76069801487658850, 8.513798778646419763, -27.72809068051395442 ) ) ;
#8733=CARTESIAN_POINT ( 'NONE',  ( 9.606819337878498288, -18.10969338424137831, -29.34610233316817585 ) ) ;
#8737=CARTESIAN_POINT ( 'NONE',  ( -14.92028588230428987, 25.84647088687363237, -9.706342443300702172 ) ) ;
#8738=CARTESIAN_POINT ( 'NONE',  ( -13.91976629483763972, -16.67082186115019482, -24.55897349996614665 ) ) ;
#8739=CARTESIAN_POINT ( 'NONE',  ( 8.893966021365395491, -18.47319264949478779, -30.00000000000000000 ) ) ;
#8744=CARTESIAN_POINT ( 'NONE',  ( -6.444683815770512858, 21.56947076293902654, -23.23860985537865886 ) ) ;
#8745=CYLINDRICAL_SURFACE ( 'NONE', #28336, 16.00000000000000711 ) ;
#8750=CARTESIAN_POINT ( 'NONE',  ( 21.26671072780636251, 0.8446411308849943733, -25.02192136719475712 ) ) ;
#8755=CARTESIAN_POINT ( 'NONE',  ( -30.69713694106416568, -0.001249014335545420122, -6.887971490028672150 ) ) ;
#8758=CARTESIAN_POINT ( 'NONE',  ( 31.99794295650106690, -3.876779942215285324, -10.41291006183080725 ) ) ;
#8762=EDGE_CURVE ( 'NONE', #10807, #32040, #9274, .T. ) ;
#8764=FACE_OUTER_BOUND ( 'NONE', #2517, .T. ) ;
#8770=CARTESIAN_POINT ( 'NONE',  ( 5.459820500924835507, 28.05023579833048686, -16.71664541261905157 ) ) ;
#8774=CARTESIAN_POINT ( 'NONE',  ( 19.79884881832018806, -27.24719281008185590, -5.457829539577221389 ) ) ;
#8780=EDGE_LOOP ( 'NONE', ( #8683, #13125, #1023, #28790 ) ) ;
#8781=CARTESIAN_POINT ( 'NONE',  ( 15.39300221565557436, 26.86528302342467001, -5.473805150799548436 ) ) ;
#8784=CARTESIAN_POINT ( 'NONE',  ( -15.38278943354864836, 26.63434012099637727, -6.417044010450005942 ) ) ;
#8787=CARTESIAN_POINT ( 'NONE',  ( 9.930210031747556343, -18.82842284079468698, -25.01870781754495709 ) ) ;
#8790=CARTESIAN_POINT ( 'NONE',  ( 11.14269862834027158, 17.45542210456148879, -27.45318300851278082 ) ) ;
#8793=CARTESIAN_POINT ( 'NONE',  ( 30.49893448008974417, -18.04955498499799305, -11.06631362726178835 ) ) ;
#8795=CARTESIAN_POINT ( 'NONE',  ( -14.61184883681244884, 26.27612152894188213, -10.14089745567681078 ) ) ;
#8797=CARTESIAN_POINT ( 'NONE',  ( -20.57926088536441966, -27.21289976561331514, -5.455544558262904076 ) ) ;
#8798=CARTESIAN_POINT ( 'NONE',  ( -15.29245034909719081, 32.56469986039895304, -4.999999999999988454 ) ) ;
#8800=CARTESIAN_POINT ( 'NONE',  ( -19.38376532770186600, -6.700500133912340672, -29.23023060093576930 ) ) ;
#8801=CARTESIAN_POINT ( 'NONE',  ( -14.97946999438102189, -26.42093270519550074, -7.359069949749521555 ) ) ;
#8804=CARTESIAN_POINT ( 'NONE',  ( 20.76747401923929104, 2.389443645289128337, -26.35181366210539977 ) ) ;
#8808=CARTESIAN_POINT ( 'NONE',  ( -30.77003892953206332, -0.07641085285610303701, -6.886502699455107290 ) ) ;
#8810=CARTESIAN_POINT ( 'NONE',  ( 30.69110547573335168, -1.275449444801196597, -10.08822704699340456 ) ) ;
#8814=CARTESIAN_POINT ( 'NONE',  ( -25.39309054194246329, 3.513990607092289054, -13.69008351871648443 ) ) ;
#8824=CARTESIAN_POINT ( 'NONE',  ( -22.58227240774737510, 6.801869239798123523, -15.85529687906895369 ) ) ;
#8828=CARTESIAN_POINT ( 'NONE',  ( 24.88102591590622836, -25.82163281467740745, -7.612408864933811969 ) ) ;
#8829=FACE_OUTER_BOUND ( 'NONE', #16928, .T. ) ;
#8831=CARTESIAN_POINT ( 'NONE',  ( 11.13836630440169984, 18.17080407247200924, -24.99097017320102054 ) ) ;
#8834=CARTESIAN_POINT ( 'NONE',  ( -16.59571780117528306, 22.97185772529794434, -5.474759697025393557 ) ) ;
#8837=CARTESIAN_POINT ( 'NONE',  ( 12.15468870735817752, 19.89582195369037620, -20.54525176704591516 ) ) ;
#8841=AXIS2_PLACEMENT_3D ( 'NONE', #38010, #13020, #34970 ) ;
#8842=CARTESIAN_POINT ( 'NONE',  ( -11.00971296877878558, 17.54494704588714882, -27.44286833666322067 ) ) ;
#8844=CARTESIAN_POINT ( 'NONE',  ( -15.47037888674134187, -26.61430711100896573, -6.886084615588098146 ) ) ;
#8847=CARTESIAN_POINT ( 'NONE',  ( -18.36169979798018304, -11.08193507441912296, -25.57557639782013936 ) ) ;
#8848=CARTESIAN_POINT ( 'NONE',  ( -13.94379063328525703, -26.36485034788368864, -4.999999999999999112 ) ) ;
#8850=CARTESIAN_POINT ( 'NONE',  ( 12.12823232338804402, 16.57707950519044005, -28.75067251775697486 ) ) ;
#8852=CARTESIAN_POINT ( 'NONE',  ( 25.22318582504367868, 6.470064654807184290, -6.921000316633144855 ) ) ;
#8858=CARTESIAN_POINT ( 'NONE',  ( -30.00628679341476968, -0.6868000848423935212, -10.59368060977712389 ) ) ;
#8859=CARTESIAN_POINT ( 'NONE',  ( 24.62928168306611454, 0.2893784230877288199, -18.43276624462634317 ) ) ;
#8862=CARTESIAN_POINT ( 'NONE',  ( 35.84808252048253507, -3.038699442442335030, -4.999999999999996447 ) ) ;
#8870=CARTESIAN_POINT ( 'NONE',  ( 1.992325487150441665, 27.82770543502457983, -17.60688455110214790 ) ) ;
#8878=CARTESIAN_POINT ( 'NONE',  ( 13.73764686189923445, 25.77870856457095172, -12.44422647077569266 ) ) ;
#8881=CARTESIAN_POINT ( 'NONE',  ( -19.19919298765988813, 15.16185000874999211, -10.86730081220202671 ) ) ;
#8885=CARTESIAN_POINT ( 'NONE',  ( 15.40837845075638057, -26.64760342190364995, -6.417007949787735477 ) ) ;
#8886=CARTESIAN_POINT ( 'NONE',  ( -21.22055300418212553, -26.61708612678433283, -8.117996566443485662 ) ) ;
#8888=CARTESIAN_POINT ( 'NONE',  ( 13.47312776821850200, 22.85298590836225330, -15.44645774616055967 ) ) ;
#8893=CARTESIAN_POINT ( 'NONE',  ( -18.15993858576987563, -15.09575340168067470, -21.92571465217806193 ) ) ;
#8894=CARTESIAN_POINT ( 'NONE',  ( 1.503347432918254123, -22.43982916438487152, -18.02207112121201504 ) ) ;
#8895=CARTESIAN_POINT ( 'NONE',  ( 14.48665838210651025, 23.98092697758879410, -12.56944135157504228 ) ) ;
#8896=CARTESIAN_POINT ( 'NONE',  ( 20.72086712622418148, 12.75943518406283594, -9.890071669578944125 ) ) ;
#8898=CARTESIAN_POINT ( 'NONE',  ( -2.905413696073824603, 20.70236046713645095, -26.99976967470244560 ) ) ;
#8900=CARTESIAN_POINT ( 'NONE',  ( -34.13545392654325639, -6.417351548865673827, -8.088078764923306352 ) ) ;
#8909=CARTESIAN_POINT ( 'NONE',  ( -30.15656701667666439, 0.6301168163923819288, -6.418133929584069364 ) ) ;
#8910=EDGE_CURVE ( 'NONE', #5646, #19243, #726, .T. ) ;
#8911=CARTESIAN_POINT ( 'NONE',  ( 34.05585594407177297, -13.68619932326567756, -8.863084868655485948 ) ) ;
#8914=EDGE_LOOP ( 'NONE', ( #27107, #9370, #4644, #27794 ) ) ;
#8921=CARTESIAN_POINT ( 'NONE',  ( -1.811830127027588722, 22.73191323099810290, -23.00449321371658939 ) ) ;
#8925=CARTESIAN_POINT ( 'NONE',  ( 18.78373925409778877, -14.41787429400073428, -21.88907065838856525 ) ) ;
#8927=CARTESIAN_POINT ( 'NONE',  ( 16.30460026483097735, 12.60001878089315674, -27.71906073260982595 ) ) ;
#8929=CARTESIAN_POINT ( 'NONE',  ( 13.05426751670861130, 31.50888625344096994, -6.795852486021440875 ) ) ;
#8931=ORIENTED_EDGE ( 'NONE', *, *, #17882, .F. ) ;
#8932=CARTESIAN_POINT ( 'NONE',  ( -18.69324927053147789, 8.492311550642993367, -28.85813498384544218 ) ) ;
#8935=CARTESIAN_POINT ( 'NONE',  ( 14.99763921991110571, -25.86109370504824412, -9.702356291737144645 ) ) ;
#8938=FACE_OUTER_BOUND ( 'NONE', #18407, .T. ) ;
#8939=CARTESIAN_POINT ( 'NONE',  ( -15.00345964543641308, 26.01693641737093543, -9.235896020594065448 ) ) ;
#8940=CARTESIAN_POINT ( 'NONE',  ( -17.77420980351482171, -19.95186716711776143, -17.87573902456129460 ) ) ;
#8941=CARTESIAN_POINT ( 'NONE',  ( 12.51658123429344371, -25.23695220677343798, -10.22225441809272617 ) ) ;
#8945=CARTESIAN_POINT ( 'NONE',  ( -10.67202016487744309, 32.33296029975388564, -9.856390611844069838 ) ) ;
#8950=CARTESIAN_POINT ( 'NONE',  ( 30.44811295758598391, 0.02673777661638704339, -7.828045874607348686 ) ) ;
#8955=CARTESIAN_POINT ( 'NONE',  ( -30.60578642345652156, -0.007519314768002983290, -7.357895972641363080 ) ) ;
#8958=CARTESIAN_POINT ( 'NONE',  ( 20.84933153278981166, -4.276367845268469026, -25.81179670892463918 ) ) ;
#8974=CARTESIAN_POINT ( 'NONE',  ( 6.877368450614945061, 35.27937098263085858, -9.323842147869731534 ) ) ;
#8976=CARTESIAN_POINT ( 'NONE',  ( 16.53758848021426076, -26.97586464850826005, -5.469368573213387208 ) ) ;
#8982=CARTESIAN_POINT ( 'NONE',  ( -15.18305171862558645, 26.25295951765882307, -8.297948513766829848 ) ) ;
#8983=CIRCLE ( 'NONE', #7673, 16.00000000000001066 ) ;
#8985=CARTESIAN_POINT ( 'NONE',  ( 14.79500207508366216, -26.08087507433808483, -8.770434559489167725 ) ) ;
#8990=CARTESIAN_POINT ( 'NONE',  ( -11.39786025644706768, 22.73419919495342256, -18.20970581293603985 ) ) ;
#8992=CARTESIAN_POINT ( 'NONE',  ( -14.28885256234768164, -20.44271994159482020, -19.17122735343420459 ) ) ;
#8996=CARTESIAN_POINT ( 'NONE',  ( -23.11120214780726201, -7.974055487576295675, -20.80445922199539055 ) ) ;
#8997=CARTESIAN_POINT ( 'NONE',  ( -14.29598325306471907, -25.39746503277514122, -10.66025640362116533 ) ) ;
#9000=CARTESIAN_POINT ( 'NONE',  ( 22.44741482142110911, 1.549842875461872937, -21.73216677922275863 ) ) ;
#9004=CARTESIAN_POINT ( 'NONE',  ( -23.96634676013683318, 0.4262288974861807023, -19.48813325609940605 ) ) ;
#9006=CARTESIAN_POINT ( 'NONE',  ( 31.77445454197319563, -1.004264897904582954, -5.468445260902000449 ) ) ;
#9010=CARTESIAN_POINT ( 'NONE',  ( -24.98802169602269174, 2.696897768699792586, -15.63010232505275177 ) ) ;
#9023=CARTESIAN_POINT ( 'NONE',  ( -24.75996061988843167, 7.109052737702043601, -6.924578970779640130 ) ) ;
#9026=CARTESIAN_POINT ( 'NONE',  ( 14.20597032484196376, -14.79219592438034780, -29.99999999999998934 ) ) ;
#9028=CARTESIAN_POINT ( 'NONE',  ( 11.74151979421917957, 19.54197345652316287, -21.58831892365258653 ) ) ;
#9031=CARTESIAN_POINT ( 'NONE',  ( -15.62169025857701499, 22.97777262041562807, -10.70896060004613659 ) ) ;
#9036=CARTESIAN_POINT ( 'NONE',  ( 15.42861054628522233, 26.73803055450190058, -4.999999999999998224 ) ) ;
#9037=ORIENTED_EDGE ( 'NONE', *, *, #32237, .T. ) ;
#9040=CARTESIAN_POINT ( 'NONE',  ( -11.37233562734991743, 18.53355911076921458, -23.83618781163009714 ) ) ;
#9042=CARTESIAN_POINT ( 'NONE',  ( -12.06406342568560852, -21.47399357335907411, -18.43280010396646773 ) ) ;
#9046=CARTESIAN_POINT ( 'NONE',  ( -33.93084094755159441, -17.77584818155513702, -6.276893119624509687 ) ) ;
#9047=CARTESIAN_POINT ( 'NONE',  ( -7.556576989782998410, -19.27055189435807137, -27.57996940079889825 ) ) ;
#9049=CARTESIAN_POINT ( 'NONE',  ( 14.65083719384613659, 22.52921530560692887, -13.58206962684690922 ) ) ;
#9051=CARTESIAN_POINT ( 'NONE',  ( 19.17388597792686866, 7.309708964681583154, -28.84800037308729515 ) ) ;
#9052=CARTESIAN_POINT ( 'NONE',  ( -75.15099915297791711, 43.38844959084113384, -5.000000000000000000 ) ) ;
#9054=CARTESIAN_POINT ( 'NONE',  ( -20.57924982997939622, -27.21273881503329051, -4.999999999999998224 ) ) ;
#9057=CARTESIAN_POINT ( 'NONE',  ( -20.49507156785942641, -0.4678258087238867380, -30.00000000000000000 ) ) ;
#9058=CARTESIAN_POINT ( 'NONE',  ( 30.67844260339930074, -0.08294063150054889477, -7.355559089466812139 ) ) ;
#9063=CARTESIAN_POINT ( 'NONE',  ( 20.90924525106827758, -8.502318254486461058, -30.00000000000001421 ) ) ;
#9070=CARTESIAN_POINT ( 'NONE',  ( 2.547048354218667043, 35.22824564786088075, -11.07258388855395914 ) ) ;
#9078=CARTESIAN_POINT ( 'NONE',  ( 14.50911442997946388, 26.55381056816341712, -10.12498485435761886 ) ) ;
#9081=CARTESIAN_POINT ( 'NONE',  ( -16.50249576148715036, 14.88229690510866199, -20.02363424797698954 ) ) ;
#9084=CARTESIAN_POINT ( 'NONE',  ( 14.87432661258679900, -25.83349755148350013, -9.709001257180572608 ) ) ;
#9086=CARTESIAN_POINT ( 'NONE',  ( -21.53459943946054622, -26.97023605249422928, -6.785410596037112718 ) ) ;
#9088=CARTESIAN_POINT ( 'NONE',  ( 15.16643734843948721, 26.30888157207252931, -8.296799070927670883 ) ) ;
#9091=CARTESIAN_POINT ( 'NONE',  ( -9.526537139939113885, -18.29543337056835028, -28.07984914598426229 ) ) ;
#9093=CARTESIAN_POINT ( 'NONE',  ( -21.21462556743105310, -17.67001013903248108, -17.67149726547187072 ) ) ;
#9094=CARTESIAN_POINT ( 'NONE',  ( 1.281579315327491253, -20.83699243184387129, -25.51341547554553202 ) ) ;
#9095=CARTESIAN_POINT ( 'NONE',  ( 15.24262546998190437, 25.26847083144028971, -9.247276495989826373 ) ) ;
#9096=CARTESIAN_POINT ( 'NONE',  ( 21.57989771907153198, 12.01233037074124788, -6.940427116014089570 ) ) ;
#9098=CARTESIAN_POINT ( 'NONE',  ( -3.498807313483044634, 20.43805243329230592, -27.74525970097024086 ) ) ;
#9100=CARTESIAN_POINT ( 'NONE',  ( -30.36244809506906606, -4.747588337124046376, -13.13675111056742217 ) ) ;
#9106=CARTESIAN_POINT ( 'NONE',  ( -20.78574042926797460, 1.163748492297181025, -26.85583114029146401 ) ) ;
#9108=CARTESIAN_POINT ( 'NONE',  ( 33.14339359398684337, -13.30814253901729316, -10.19541812155104488 ) ) ;
#9119=CARTESIAN_POINT ( 'NONE',  ( -3.045440459837997604, 37.80942315677882704, -7.122015871823959898 ) ) ;
#9121=DIRECTION ( 'NONE',  ( 1.000000000000000000, 0.000000000000000000, 0.000000000000000000 ) ) ;
#9123=CARTESIAN_POINT ( 'NONE',  ( 16.27615822911637622, -12.47890632334475924, -30.00000000000001421 ) ) ;
#9124=CARTESIAN_POINT ( 'NONE',  ( 19.48931724336470594, 15.88182490461431406, -6.933233223513477483 ) ) ;
#9125=CARTESIAN_POINT ( 'NONE',  ( 8.160668170145010336, 19.01481104899739094, -27.91480984821776801 ) ) ;
#9126=EDGE_LOOP ( 'NONE', ( #24357, #19443, #37182, #30732, #15343, #23399 ) ) ;
#9127=CARTESIAN_POINT ( 'NONE',  ( -19.83482056652078640, 8.857944167693910131, -21.15899509700257042 ) ) ;
#9129=CARTESIAN_POINT ( 'NONE',  ( 10.65945867603157815, -19.54002146369526827, -22.71882543429452284 ) ) ;
#9131=EDGE_CURVE ( 'NONE', #17337, #31250, #22974, .T. ) ;
#9133=CARTESIAN_POINT ( 'NONE',  ( 16.77267017469755217, -29.13948811618736912, -5.000000000000000888 ) ) ;
#9136=CARTESIAN_POINT ( 'NONE',  ( -12.11893889750869135, 19.93834885319187578, -20.53850700616269265 ) ) ;
#9137=CARTESIAN_POINT ( 'NONE',  ( -24.97569650337160496, -26.32149808972361527, -5.000000000000002665 ) ) ;
#9138=CARTESIAN_POINT ( 'NONE',  ( 8.369344652847257038, -18.90615068489544370, -27.52829367847808939 ) ) ;
#9141=CARTESIAN_POINT ( 'NONE',  ( -9.109889474751160066, 30.44524786122741489, -13.03254955294998751 ) ) ;
#9146=ORIENTED_EDGE ( 'NONE', *, *, #3441, .F. ) ;
#9147=CARTESIAN_POINT ( 'NONE',  ( 27.12540744812873683, 0.2567673158908028719, -14.47800510790882633 ) ) ;
#9149=CARTESIAN_POINT ( 'NONE',  ( 14.21391437420825099, 30.04769070240185869, -5.000000000000000000 ) ) ;
#9152=CARTESIAN_POINT ( 'NONE',  ( -27.70776136782869514, 0.2300040921888646395, -13.51576448074164993 ) ) ;
#9156=CARTESIAN_POINT ( 'NONE',  ( 26.10825148640684645, -4.601592950812219307, -17.92875175135799282 ) ) ;
#9168=CARTESIAN_POINT ( 'NONE',  ( 32.33143948541791701, 1.358872982501826865, 0.000000000000000000 ) ) ;
#9171=CARTESIAN_POINT ( 'NONE',  ( 5.041034891940512352, 25.97319188981542837, -18.71755947577446832 ) ) ;
#9172=CIRCLE ( 'NONE', #21494, 17.00000000000000355 ) ;
#9174=AXIS2_PLACEMENT_3D ( 'NONE', #7345, #13447, #19751 ) ;
#9175=CARTESIAN_POINT ( 'NONE',  ( 16.28251897248971503, -25.35181217798053765, -11.46904951680661000 ) ) ;
#9178=FACE_BOUND ( 'NONE', #3838, .T. ) ;
#9180=ORIENTED_EDGE ( 'NONE', *, *, #34335, .F. ) ;
#9181=CARTESIAN_POINT ( 'NONE',  ( -14.40426848691212847, 24.18477772179416974, -12.56146234885731872 ) ) ;
#9183=CARTESIAN_POINT ( 'NONE',  ( 9.629772704453449350, -18.63330705237584439, -26.23951421163814501 ) ) ;
#9188=CARTESIAN_POINT ( 'NONE',  ( -10.11312864869621286, 18.12346847508388237, -27.37340818524439001 ) ) ;
#9189=CARTESIAN_POINT ( 'NONE',  ( -20.43668249186664454, -27.04690955953348208, -6.800953625143487002 ) ) ;
#9192=CARTESIAN_POINT ( 'NONE',  ( -19.96736081760328574, -5.571863482751658658, -27.79030427704988071 ) ) ;
#9193=CARTESIAN_POINT ( 'NONE',  ( -11.76341657271260743, -21.49608334009564814, -18.46619230194481887 ) ) ;
#9196=CARTESIAN_POINT ( 'NONE',  ( 24.67560003803047408, 1.382580745444311088, -17.53657882121196465 ) ) ;
#9202=CARTESIAN_POINT ( 'NONE',  ( -22.74375665350138220, 0.5678067076679078617, -21.61155036081104086 ) ) ;
#9204=CARTESIAN_POINT ( 'NONE',  ( 32.43268799775532329, -2.266782117739180258, -7.289905317446092603 ) ) ;
#9206=CARTESIAN_POINT ( 'NONE',  ( -12.11431921870781281, -16.53859995802357474, -30.00000000000001066 ) ) ;
#9210=CARTESIAN_POINT ( 'NONE',  ( -20.30511407948876013, 2.906241227738919353, -29.99999999999999645 ) ) ;
#9218=ORIENTED_EDGE ( 'NONE', *, *, #355, .F. ) ;
#9219=CARTESIAN_POINT ( 'NONE',  ( -23.53005843440588052, 6.935657865434798452, -12.82094700181943558 ) ) ;
#9222=CARTESIAN_POINT ( 'NONE',  ( 15.12372412105587571, -15.73678478649937595, -24.44085377604933029 ) ) ;
#9224=CARTESIAN_POINT ( 'NONE',  ( 10.82761120373386099, 17.56290797765107925, -28.06474652081093879 ) ) ;
#9226=CARTESIAN_POINT ( 'NONE',  ( -12.87412475669415102, 16.08929808775789638, -28.17534248950969200 ) ) ;
#9229=EDGE_CURVE ( 'NONE', #35064, #10849, #39649, .T. ) ;
#9231=CARTESIAN_POINT ( 'NONE',  ( 11.91420444604188233, 19.35880423362332436, -21.62089463913763865 ) ) ;
#9233=DIRECTION ( 'NONE',  ( -0.000000000000000000, -0.000000000000000000, -1.000000000000000000 ) ) ;
#9235=CARTESIAN_POINT ( 'NONE',  ( -10.88833724461483321, 17.42332960106011797, -28.70205193506265573 ) ) ;
#9237=CARTESIAN_POINT ( 'NONE',  ( -13.19604288844774054, -23.10384307990375419, -15.43186663979633977 ) ) ;
#9239=CARTESIAN_POINT ( 'NONE',  ( -18.98149992151875054, -9.954718304477847113, -25.58083087282487611 ) ) ;
#9240=CARTESIAN_POINT ( 'NONE',  ( -8.776592290562826193, -18.65192578191585326, -28.11862783572077618 ) ) ;
#9242=CARTESIAN_POINT ( 'NONE',  ( 14.89222191165484155, 22.99967983981807862, -12.60792089205823174 ) ) ;
#9245=CARTESIAN_POINT ( 'NONE',  ( 26.63862888549859065, 4.673691467239231123, -6.432048232843499136 ) ) ;
#9250=CARTESIAN_POINT ( 'NONE',  ( -18.98517864108453068, -25.27528660209288702, -11.33194676435389248 ) ) ;
#9252=CARTESIAN_POINT ( 'NONE',  ( -21.06315986593275369, -0.5327104372337403415, -26.10652535518945427 ) ) ;
#9253=CARTESIAN_POINT ( 'NONE',  ( 26.72259468233993118, -0.05410243562783979832, -15.41034757420027290 ) ) ;
#9258=CARTESIAN_POINT ( 'NONE',  ( 33.62187204924162387, 0.04418559750794539415, -5.000000000000000000 ) ) ;
#9263=VECTOR ( 'NONE', #27940, 1000.000000000000000 ) ;
#9267=CARTESIAN_POINT ( 'NONE',  ( 1.444440266932477401, 20.45847851156178265, -30.00000000000001066 ) ) ;
#9274=LINE ( 'NONE', #33674, #17137 ) ;
#9275=CARTESIAN_POINT ( 'NONE',  ( 15.09524128205707072, 27.81033699783984403, -5.000000000000000000 ) ) ;
#9279=CARTESIAN_POINT ( 'NONE',  ( -15.96198011527028626, 14.19337421597026605, -23.24198305949962418 ) ) ;
#9282=CARTESIAN_POINT ( 'NONE',  ( 9.694524255575014848, -18.43926002963515742, -26.83009326277129603 ) ) ;
#9283=CARTESIAN_POINT ( 'NONE',  ( -13.37002884985804840, -17.04744882218747648, -24.61733060730478684 ) ) ;
#9284=CARTESIAN_POINT ( 'NONE',  ( 15.36806905513554788, 26.68643454456317698, -6.416988418440872088 ) ) ;
#9285=CARTESIAN_POINT ( 'NONE',  ( 12.92457025990295527, 21.65936192259344750, -17.43674491296770057 ) ) ;
#9289=CARTESIAN_POINT ( 'NONE',  ( -15.29737515392600322, -26.57080565899713775, -6.888077247771704492 ) ) ;
#9292=CARTESIAN_POINT ( 'NONE',  ( -29.90225311088989812, -23.39525860678804037, -5.000000000000006217 ) ) ;
#9294=CARTESIAN_POINT ( 'NONE',  ( -0.3741226908721868027, -24.24193228020686064, -10.38565774725202928 ) ) ;
#9295=CARTESIAN_POINT ( 'NONE',  ( 11.19848097534155684, 17.17100607549662072, -29.35292330717537368 ) ) ;
#9296=CARTESIAN_POINT ( 'NONE',  ( 22.78013759795664939, 10.15463924895263226, -5.966147905284203468 ) ) ;
#9298=ADVANCED_FACE ( 'NONE', ( #21562 ), #15870, .F. ) ;
#9299=CARTESIAN_POINT ( 'NONE',  ( -5.301386336604020144, 37.38718629579432928, -6.707813491147157414 ) ) ;
#9301=ORIENTED_EDGE ( 'NONE', *, *, #10524, .F. ) ;
#9302=CARTESIAN_POINT ( 'NONE',  ( -23.51180566201336930, -4.338079614371764592, -21.05291888185874427 ) ) ;
#9308=CARTESIAN_POINT ( 'NONE',  ( -29.40640376299546688, 0.6751206212795356487, -9.249095237612971587 ) ) ;
#9309=CARTESIAN_POINT ( 'NONE',  ( 21.49173964087244570, -7.212581857489289483, -23.10824091391128476 ) ) ;
#9322=CARTESIAN_POINT ( 'NONE',  ( -2.282314974550741837, 20.78572398550833000, -26.98632778830081236 ) ) ;
#9326=CARTESIAN_POINT ( 'NONE',  ( 22.88038781354014262, -17.60680147475983759, -16.66587105011879544 ) ) ;
#9327=CARTESIAN_POINT ( 'NONE',  ( 17.03883565536520450, 14.60776677102190213, -18.99045918486842410 ) ) ;
#9329=CARTESIAN_POINT ( 'NONE',  ( 12.90021850856434327, 31.07188364411424786, -8.136059182505970711 ) ) ;
#9331=CARTESIAN_POINT ( 'NONE',  ( -20.43794256383087671, 11.06939829604054992, -14.91976663991167662 ) ) ;
#9333=( GEOMETRIC_REPRESENTATION_CONTEXT ( 3 ) GLOBAL_UNCERTAINTY_ASSIGNED_CONTEXT ( ( #29484 ) ) GLOBAL_UNIT_ASSIGNED_CONTEXT ( ( #33951, #22743, #818 ) ) REPRESENTATION_CONTEXT ( 'NONE', 'WORKASPACE' ) );
#9334=CARTESIAN_POINT ( 'NONE',  ( 10.61757206484970517, -19.55229676520039561, -22.72432018335026171 ) ) ;
#9336=CARTESIAN_POINT ( 'NONE',  ( -11.41987377193683528, -19.41918266173334828, -30.00000000000000000 ) ) ;
#9339=CARTESIAN_POINT ( 'NONE',  ( -11.66966591706341383, 18.92733846212934878, -22.73230586722390356 ) ) ;
#9340=CARTESIAN_POINT ( 'NONE',  ( -19.41909531571028324, -23.12033621153826957, -14.04196714719246231 ) ) ;
#9341=CARTESIAN_POINT ( 'NONE',  ( 9.856402666990103256, -24.08899994559548574, -12.70246950836210331 ) ) ;
#9344=CARTESIAN_POINT ( 'NONE',  ( -8.712598976131317841, 26.30495431820440899, -16.88202031406565240 ) ) ;
#9350=CARTESIAN_POINT ( 'NONE',  ( 20.52661814301616161, 0.8646301841086654338, -28.70720715481454377 ) ) ;
#9351=CARTESIAN_POINT ( 'NONE',  ( -1.732915686479672868, 38.50000000000000711, -4.999999999999999112 ) ) ;
#9355=CARTESIAN_POINT ( 'NONE',  ( -20.48102978849703604, 0.8817738089609830077, -29.34878050620392642 ) ) ;
#9358=CARTESIAN_POINT ( 'NONE',  ( 26.18805396461011981, -5.413810846952083367, -17.87313096885579355 ) ) ;
#9359=AXIS2_PLACEMENT_3D ( 'NONE', #7769, #20171, #32568 ) ;
#9362=MANIFOLD_SOLID_BREP ( 'Extrude-Thin3', #11266 ) ;
#9370=ORIENTED_EDGE ( 'NONE', *, *, #19463, .F. ) ;
#9375=CARTESIAN_POINT ( 'NONE',  ( 6.036156669524302743, 23.50249717186115106, -20.88789013247724924 ) ) ;
#9376=CARTESIAN_POINT ( 'NONE',  ( 16.74105887149018201, -25.99454892381202598, -10.07209973717082008 ) ) ;
#9381=CARTESIAN_POINT ( 'NONE',  ( -13.50669571649333456, 22.78588612237093614, -15.45264257089643500 ) ) ;
#9383=CARTESIAN_POINT ( 'NONE',  ( 14.22552846898557632, -25.04752998104490302, -11.60275637146618344 ) ) ;
#9388=CARTESIAN_POINT ( 'NONE',  ( -12.03032039410056697, 24.14510420486799092, -16.21622471958081491 ) ) ;
#9390=CARTESIAN_POINT ( 'NONE',  ( -19.71199086647830967, -26.17691209112436113, -9.501020231640085356 ) ) ;
#9395=CARTESIAN_POINT ( 'NONE',  ( -27.12574315244719614, -8.434033646970773290, -16.74782370223186589 ) ) ;
#9396=CARTESIAN_POINT ( 'NONE',  ( -11.30698307648105860, -21.00710847950110249, -19.52216458991920689 ) ) ;
#9399=CARTESIAN_POINT ( 'NONE',  ( 30.47359799298996208, 0.2308879069823202845, -6.888633799088443865 ) ) ;
#9403=CARTESIAN_POINT ( 'NONE',  ( -20.48278845350746380, 0.8398715278162421916, -30.00000000000000000 ) ) ;
#9404=ORIENTED_EDGE ( 'NONE', *, *, #24047, .T. ) ;
#9405=CARTESIAN_POINT ( 'NONE',  ( 32.32777460232222211, -1.841093328404687313, -6.383748192902252150 ) ) ;
#9409=CARTESIAN_POINT ( 'NONE',  ( -20.13976743542029979, 4.300193810599860278, -28.21449245398771666 ) ) ;
#9413=AXIS2_PLACEMENT_3D ( 'NONE', #5034, #8078, #36122 ) ;
#9422=CARTESIAN_POINT ( 'NONE',  ( -24.83346892669243289, 7.119045183397740395, -5.960013684747799800 ) ) ;
#9425=CARTESIAN_POINT ( 'NONE',  ( 22.95410551231090679, -26.66747533545364135, -6.768454890417195280 ) ) ;
#9428=CARTESIAN_POINT ( 'NONE',  ( 15.13821314949306185, 26.72040169015227562, -7.817432155278004835 ) ) ;
#9430=CARTESIAN_POINT ( 'NONE',  ( -14.26164166507406605, 20.40696190269933297, -16.59697255856162101 ) ) ;
#9434=CARTESIAN_POINT ( 'NONE',  ( 15.31765784529594931, 26.43575136356594157, -7.358154011196789135 ) ) ;
#9436=LINE ( 'NONE', #24669, #21614 ) ;
#9438=CARTESIAN_POINT ( 'NONE',  ( -11.07006266871842470, 17.83849166442784906, -26.21249532911198088 ) ) ;
#9440=CARTESIAN_POINT ( 'NONE',  ( -15.39884463545014626, -26.43030500914523628, -7.822979998916790301 ) ) ;
#9444=CARTESIAN_POINT ( 'NONE',  ( -21.03375321176811852, -11.02753040179103472, -21.84322230830700562 ) ) ;
#9445=CARTESIAN_POINT ( 'NONE',  ( -13.92516281751823470, -26.33641981794989917, -5.946789951340505809 ) ) ;
#9447=CARTESIAN_POINT ( 'NONE',  ( 16.80931989995731968, 22.07997525327169086, -6.903476050494520955 ) ) ;
#9449=CARTESIAN_POINT ( 'NONE',  ( 20.02244736892210497, 5.216203046238859997, -27.08051660729452692 ) ) ;
#9455=CARTESIAN_POINT ( 'NONE',  ( -21.83110320996402010, 0.04483480959028030011, -23.77064350941624582 ) ) ;
#9456=CARTESIAN_POINT ( 'NONE',  ( 31.24124332302707785, -0.3963250197696455701, -5.000000000000000888 ) ) ;
#9462=CARTESIAN_POINT ( 'NONE',  ( 26.31271763591405133, -28.25584584496056806, -4.999999999999990230 ) ) ;
#9469=CARTESIAN_POINT ( 'NONE',  ( 2.331359131675258212, 32.30025893414131133, -13.81255405787268487 ) ) ;
#9477=CARTESIAN_POINT ( 'NONE',  ( 14.09416554623298090, 26.10268081555338782, -11.51672208091659400 ) ) ;
#9481=CARTESIAN_POINT ( 'NONE',  ( -16.01922876754991876, 15.59330759611457218, -19.98676936076589428 ) ) ;
#9486=CARTESIAN_POINT ( 'NONE',  ( 15.46971733045241670, -26.73784336799789330, -5.474200668421835836 ) ) ;
#9487=CARTESIAN_POINT ( 'NONE',  ( -21.65417613035611311, -27.10241255109310998, -5.897512186717746019 ) ) ;
#9488=CARTESIAN_POINT ( 'NONE',  ( 14.84347862571135224, 25.59847897344355161, -10.18086840633468348 ) ) ;
#9489=CARTESIAN_POINT ( 'NONE',  ( 10.96874445820387223, 17.31868006298826046, -29.34801594517404411 ) ) ;
#9493=CARTESIAN_POINT ( 'NONE',  ( -12.94992061884572365, -23.08857923432204373, -15.45460198982821787 ) ) ;
#9495=CARTESIAN_POINT ( 'NONE',  ( -24.80417270723568279, -17.12426492970035241, -15.69038464299936386 ) ) ;
#9496=CARTESIAN_POINT ( 'NONE',  ( 1.610546824266047006, -23.23319193122145165, -14.92450978981246656 ) ) ;
#9497=CARTESIAN_POINT ( 'NONE',  ( 15.58097433184440206, 25.94823047040191710, -6.417925113058433162 ) ) ;
#9498=CARTESIAN_POINT ( 'NONE',  ( 21.51745293842607509, 9.710779523656842827, -13.89343078686114552 ) ) ;
#9502=CARTESIAN_POINT ( 'NONE',  ( -31.67765172404683227, -3.222148243870730511, -10.44267939193049877 ) ) ;
#9507=CARTESIAN_POINT ( 'NONE',  ( -20.50889864978784161, 1.192488855597985564, -28.71852165833594484 ) ) ;
#9508=CARTESIAN_POINT ( 'NONE',  ( 35.37860232752390743, -13.03546680616358877, -5.863704084091365232 ) ) ;
#9522=CARTESIAN_POINT ( 'NONE',  ( -3.585224264196515520, 32.04905365121025795, -13.82507829668538868 ) ) ;
#9525=EDGE_CURVE ( 'NONE', #16948, #11613, #26250, .T. ) ;
#9528=DIRECTION ( 'NONE',  ( 0.000000000000000000, 0.000000000000000000, 1.000000000000000000 ) ) ;
#9529=CARTESIAN_POINT ( 'NONE',  ( 12.27639651543910837, 27.18797350401429824, -13.23837527007015602 ) ) ;
#9531=CARTESIAN_POINT ( 'NONE',  ( -21.25484840722362279, 12.72181903587277318, -5.000000000000000000 ) ) ;
#9532=CARTESIAN_POINT ( 'NONE',  ( -34.47241746879593904, 3.460351812918829761, 0.000000000000000000 ) ) ;
#9533=CARTESIAN_POINT ( 'NONE',  ( 10.08869499956528415, -18.76399072035841442, -25.00021918992353775 ) ) ;
#9535=CARTESIAN_POINT ( 'NONE',  ( 11.25614974650753375, 18.08000221745906089, -25.00715939995231096 ) ) ;
#9536=CARTESIAN_POINT ( 'NONE',  ( 21.88499642459564143, -5.528038495964486820, -20.11584339644707597 ) ) ;
#9539=CARTESIAN_POINT ( 'NONE',  ( -10.96701088540842761, 17.31978028264472513, -29.99999999999999645 ) ) ;
#9540=CARTESIAN_POINT ( 'NONE',  ( -14.45284558077854520, -15.31887616786443296, -26.42903543862076177 ) ) ;
#9541=CARTESIAN_POINT ( 'NONE',  ( 9.204648767762177997, -22.95956739582980077, -15.68808466976011040 ) ) ;
#9542=CARTESIAN_POINT ( 'NONE',  ( 14.98023422679249528, 25.65947670479530984, -9.711130374113162489 ) ) ;
#9543=CARTESIAN_POINT ( 'NONE',  ( 30.66924623482115209, -20.77338707453388977, -8.848560859720739913 ) ) ;
#9548=CARTESIAN_POINT ( 'NONE',  ( -10.07745175218284217, 33.85409929753423341, -8.493742715255910625 ) ) ;
#9553=CARTESIAN_POINT ( 'NONE',  ( 29.32892909551985028, 0.1034583756683473688, -10.65428865362305721 ) ) ;
#9557=CARTESIAN_POINT ( 'NONE',  ( -20.96646152425979537, 0.8383472484117416856, -26.22754307947055707 ) ) ;
#9560=CARTESIAN_POINT ( 'NONE',  ( 20.71247045076932736, -3.585883499709318745, -26.50471444526433373 ) ) ;
#9571=CARTESIAN_POINT ( 'NONE',  ( -16.74436491739946575, 11.83083178865852148, -30.00000000000000000 ) ) ;
#9575=CARTESIAN_POINT ( 'NONE',  ( 18.10616661872212418, 18.94352981041244277, -6.438559219923253529 ) ) ;
#9577=CARTESIAN_POINT ( 'NONE',  ( 8.932770706806998362, 34.72274584801672859, -8.469836187294838226 ) ) ;
#9578=CARTESIAN_POINT ( 'NONE',  ( 11.86460666947250964, -19.15457323191094119, -22.56163012647707333 ) ) ;
#9582=CARTESIAN_POINT ( 'NONE',  ( -15.24722010801124839, 26.35548338364083421, -7.828046445912475448 ) ) ;
#9584=CARTESIAN_POINT ( 'NONE',  ( 13.59058049318332806, -24.10307348923517523, -13.51868193062158063 ) ) ;
#9588=VERTEX_POINT ( 'NONE', #1847 ) ;
#9589=CARTESIAN_POINT ( 'NONE',  ( -10.02826340246190640, 19.59635890697872895, -23.63231146289030704 ) ) ;
#9590=CARTESIAN_POINT ( 'NONE',  ( -13.55038157627658002, -20.63826655719205760, -19.25262925335620778 ) ) ;
#9595=CARTESIAN_POINT ( 'NONE',  ( -19.64501015271085294, -6.129868598536533320, -28.49191429157074396 ) ) ;
#9596=CARTESIAN_POINT ( 'NONE',  ( -9.413550212251061922, -18.21086026825004112, -30.00000000000000000 ) ) ;
#9599=CARTESIAN_POINT ( 'NONE',  ( 20.59811166339096644, 1.045058112078671941, -28.08708561988663988 ) ) ;
#9604=CARTESIAN_POINT ( 'NONE',  ( -24.57004144261168932, 0.4099649594921800921, -18.44930745607893741 ) ) ;
#9606=CARTESIAN_POINT ( 'NONE',  ( 31.98272768806592481, -1.800652305183228830, -7.760027792917767009 ) ) ;
#9608=CARTESIAN_POINT ( 'NONE',  ( 16.15629783291639399, -12.69278426743109200, -30.00000000000003908 ) ) ;
#9611=CARTESIAN_POINT ( 'NONE',  ( -24.83189327688484838, 4.353783615239871452, -13.73059695307320105 ) ) ;
#9613=ADVANCED_FACE ( 'NONE', ( #1434, #7724 ), #17085, .T. ) ;
#9614=DIRECTION ( 'NONE',  ( 1.000000000000000000, 0.000000000000000000, 0.000000000000000000 ) ) ;
#9624=CARTESIAN_POINT ( 'NONE',  ( -21.79696480337856812, 7.571043879021812195, -16.91776734276888305 ) ) ;
#9627=CARTESIAN_POINT ( 'NONE',  ( 23.17353744146408800, -25.53105782170328553, -9.399317870189824120 ) ) ;
#9629=CARTESIAN_POINT ( 'NONE',  ( 15.32268921037612586, 27.10638078547256669, -5.472625680277237947 ) ) ;
#9632=CARTESIAN_POINT ( 'NONE',  ( -14.50975249381452592, 20.88454814334572163, -15.58843137732770856 ) ) ;
#9635=CARTESIAN_POINT ( 'NONE',  ( 15.43643446434663069, 26.70998168114506299, -4.999999999999998224 ) ) ;
#9638=EDGE_CURVE ( 'NONE', #2968, #14160, #22553, .T. ) ;
#9640=CARTESIAN_POINT ( 'NONE',  ( -13.93471959586060649, 24.16489319529103241, -13.49162670121266139 ) ) ;
#9643=CARTESIAN_POINT ( 'NONE',  ( -15.07802003622312270, -25.87832397125552220, -9.698090967223700787 ) ) ;
#9645=EDGE_CURVE ( 'NONE', #21571, #3398, #18677, .T. ) ;
#9647=CARTESIAN_POINT ( 'NONE',  ( -27.13442240602560318, -13.17128934651453598, -15.68741833354276416 ) ) ;
#9648=CARTESIAN_POINT ( 'NONE',  ( -8.888899028085873510, -18.51857346408734273, -28.73058333705254341 ) ) ;
#9650=CARTESIAN_POINT ( 'NONE',  ( 12.46547198588941896, 16.48917403503523005, -27.54678004591448470 ) ) ;
#9652=CARTESIAN_POINT ( 'NONE',  ( 25.76556103975890721, 5.561561074672148663, -7.879988086958064741 ) ) ;
#9655=CARTESIAN_POINT ( 'NONE',  ( -14.02522273992627078, -18.92975101292878293, -21.21400966844822378 ) ) ;
#9658=CARTESIAN_POINT ( 'NONE',  ( -24.88924877381098355, -0.2642620682496472084, -18.35903378176135803 ) ) ;
#9660=CARTESIAN_POINT ( 'NONE',  ( 29.57816538328471268, -0.1796088123746400478, -10.63313785040832293 ) ) ;
#9665=CARTESIAN_POINT ( 'NONE',  ( 26.31271763591406909, -28.25584584496056451, -14.26382729546506667 ) ) ;
#9672=DIRECTION ( 'NONE',  ( 0.000000000000000000, 0.000000000000000000, 1.000000000000000000 ) ) ;
#9673=CARTESIAN_POINT ( 'NONE',  ( 2.406064665179193263, 33.30697029628942119, -12.89611003825230107 ) ) ;
#9681=CARTESIAN_POINT ( 'NONE',  ( 10.27379371539876907, 17.74076016529687649, -30.00000000000000000 ) ) ;
#9682=CARTESIAN_POINT ( 'NONE',  ( -35.48538791413474769, -11.24999995268676933, -5.000000000000001776 ) ) ;
#9685=CARTESIAN_POINT ( 'NONE',  ( -15.46485185209717628, 13.55220689985132410, -28.26754509741839527 ) ) ;
#9688=CARTESIAN_POINT ( 'NONE',  ( 9.552972388026635286, -18.28221569941723601, -28.07838513181713225 ) ) ;
#9689=CARTESIAN_POINT ( 'NONE',  ( -14.02522273755474380, -18.92975100993347581, -21.21400967388834857 ) ) ;
#9690=CARTESIAN_POINT ( 'NONE',  ( 11.04317535683834883, 17.42292179296065413, -28.07760017567576583 ) ) ;
#9691=CARTESIAN_POINT ( 'NONE',  ( 15.40885724145108249, 26.80895719503613606, -5.474085382006591338 ) ) ;
#9696=CARTESIAN_POINT ( 'NONE',  ( -11.48389827485794434, -20.98450916179802306, -19.50346772467152334 ) ) ;
#9698=CARTESIAN_POINT ( 'NONE',  ( -22.40361533374172964, -16.48201631266229228, -17.62577809116323380 ) ) ;
#9699=CARTESIAN_POINT ( 'NONE',  ( -1.770315541423665318, -20.49735477589887367, -28.86146915265202750 ) ) ;
#9700=CARTESIAN_POINT ( 'NONE',  ( 14.44003496283569810, 22.99600343737122898, -13.55926162218559128 ) ) ;
#9702=CARTESIAN_POINT ( 'NONE',  ( 19.27723472360040091, 8.927243194702443319, -23.31752901678017054 ) ) ;
#9705=CARTESIAN_POINT ( 'NONE',  ( -28.41830146766454845, -3.622177512335159388, -15.08422308592607131 ) ) ;
#9711=CARTESIAN_POINT ( 'NONE',  ( -27.84741259050295170, 0.7654686433649292576, -12.57911469547112304 ) ) ;
#9712=CARTESIAN_POINT ( 'NONE',  ( 19.43389763942624882, -6.523976669268585660, -29.99999999999999645 ) ) ;
#9721=CARTESIAN_POINT ( 'NONE',  ( -3.003906060479351936, 37.17650976190002865, -8.411038520408236963 ) ) ;
#9727=CARTESIAN_POINT ( 'NONE',  ( 8.118011562862880837, 18.90506291166681052, -28.59249439703800988 ) ) ;
#9729=CARTESIAN_POINT ( 'NONE',  ( -19.25317702551486576, 10.46635355190964844, -20.12010506014689426 ) ) ;
#9731=CARTESIAN_POINT ( 'NONE',  ( 10.27113998026189989, -19.14829838377831805, -23.84809487166246811 ) ) ;
#9733=CARTESIAN_POINT ( 'NONE',  ( 13.45276934512811806, 22.89459220598109113, -15.44166492943546309 ) ) ;
#9734=CARTESIAN_POINT ( 'NONE',  ( 26.31271763591405133, -28.25584584496056806, -4.999999999999990230 ) ) ;
#9736=CARTESIAN_POINT ( 'NONE',  ( -27.01125781910978318, -25.31691801271181674, -5.870809593036823593 ) ) ;
#9737=CARTESIAN_POINT ( 'NONE',  ( 8.856982299079746213, -19.61396123686068549, -24.00676120555290183 ) ) ;
#9738=CARTESIAN_POINT ( 'NONE',  ( 15.47833181635298772, 26.56067009156167558, -4.999999999999998224 ) ) ;
#9739=CARTESIAN_POINT ( 'NONE',  ( 19.66024882222950509, -13.28965305365858818, -21.85380848813069576 ) ) ;
#9745=CARTESIAN_POINT ( 'NONE',  ( -7.666838832020851591, 32.44533431280383695, -12.05124513101535655 ) ) ;
#9749=CARTESIAN_POINT ( 'NONE',  ( 30.71313057055191820, -0.01776306241125666374, -6.887927186766908072 ) ) ;
#9755=CARTESIAN_POINT ( 'NONE',  ( -20.69195238456651964, 0.8693669606531726490, -27.44980246086476683 ) ) ;
#9758=CARTESIAN_POINT ( 'NONE',  ( 35.04727437832835335, -7.360793022001182351, -5.447201208417698837 ) ) ;
#9760=ORIENTED_EDGE ( 'NONE', *, *, #12309, .T. ) ;
#9768=CARTESIAN_POINT ( 'NONE',  ( -19.95996515113903769, 4.687952722032478370, -30.00000000000001066 ) ) ;
#9770=DIRECTION ( 'NONE',  ( 1.000000000000000000, 0.000000000000000000, 0.000000000000000000 ) ) ;
#9774=CARTESIAN_POINT ( 'NONE',  ( 17.90821008046413354, 18.66479283707571213, -8.856698538950956490 ) ) ;
#9775=CARTESIAN_POINT ( 'NONE',  ( 6.745778725514791851, 29.76450411120941908, -14.82904111780637280 ) ) ;
#9776=CARTESIAN_POINT ( 'NONE',  ( 17.60569237627828443, -25.83491465451036362, -10.48832399961285411 ) ) ;
#9780=CARTESIAN_POINT ( 'NONE',  ( -12.14918073411995003, 19.90232399862620127, -20.54428201483505134 ) ) ;
#9783=CARTESIAN_POINT ( 'NONE',  ( 15.03134232453200347, -26.43346543218465783, -7.358877968120621560 ) ) ;
#9787=ORIENTED_EDGE ( 'NONE', *, *, #13414, .T. ) ;
#9788=CARTESIAN_POINT ( 'NONE',  ( -14.39563127090040062, 29.49628440365493276, -5.920050663511798206 ) ) ;
#9792=CARTESIAN_POINT ( 'NONE',  ( -31.91225982942368233, -8.858501497912342870, -12.06783560505458297 ) ) ;
#9793=CARTESIAN_POINT ( 'NONE',  ( -15.20174574604959616, -26.47514097219373141, -7.358271501857936769 ) ) ;
#9796=CARTESIAN_POINT ( 'NONE',  ( 29.76485216031830205, 0.2778845579280027622, -9.242486094669974506 ) ) ;
#9801=CARTESIAN_POINT ( 'NONE',  ( -21.71446517679514088, 0.7002016955605907533, -23.85068631983916987 ) ) ;
#9803=CARTESIAN_POINT ( 'NONE',  ( 29.30903811477968546, -1.149447832272777248, -12.42997963733888334 ) ) ;
#9818=CARTESIAN_POINT ( 'NONE',  ( -22.97007816870513608, 9.885904127924739271, -4.999999999999999112 ) ) ;
#9819=CARTESIAN_POINT ( 'NONE',  ( 19.94105029877223600, -22.02225129578359031, -14.93283766574777616 ) ) ;
#9821=CARTESIAN_POINT ( 'NONE',  ( 10.93269978972138823, 17.59616206544103889, -27.43687381419555038 ) ) ;
#9823=CARTESIAN_POINT ( 'NONE',  ( -16.11342241529700914, 23.89935148421658440, -7.369744296171617748 ) ) ;
#9826=CARTESIAN_POINT ( 'NONE',  ( 14.54923841115265759, 24.92455583907450034, -11.60034771649255703 ) ) ;
#9830=CARTESIAN_POINT ( 'NONE',  ( -15.23769845792880950, 26.95939586459985549, -6.880603932344942386 ) ) ;
#9832=CARTESIAN_POINT ( 'NONE',  ( -10.32384819220336958, -19.12984685317730182, -23.84136453349647766 ) ) ;
#9836=CARTESIAN_POINT ( 'NONE',  ( -32.80859633437859202, -14.68931420806718435, -10.18384796241277712 ) ) ;
#9837=CARTESIAN_POINT ( 'NONE',  ( -11.36062271840278903, -22.05499941633807381, -17.51679325157146039 ) ) ;
#9839=CARTESIAN_POINT ( 'NONE',  ( 12.83478968634269712, 16.45627959073583568, -26.38328025063007232 ) ) ;
#9841=CARTESIAN_POINT ( 'NONE',  ( 26.59269643126366489, 4.672196685667098670, -6.910430442841478893 ) ) ;
#9848=CARTESIAN_POINT ( 'NONE',  ( -24.08328761345742208, 0.1459235441318743887, -19.45002103222414647 ) ) ;
#9849=CARTESIAN_POINT ( 'NONE',  ( 22.79849040394648441, 0.3847677357643901619, -21.58657492048318716 ) ) ;
#9853=CARTESIAN_POINT ( 'NONE',  ( -31.47283671532261806, -25.12609584734821766, -14.45070082761205477 ) ) ;
#9856=CARTESIAN_POINT ( 'NONE',  ( 75.15099915297797395, 43.38844959084117647, 0.000000000000000000 ) ) ;
#9861=CARTESIAN_POINT ( 'NONE',  ( 3.805984881634391748, 28.61912022499797104, -16.66590632089457458 ) ) ;
#9867=CARTESIAN_POINT ( 'NONE',  ( 10.22725543094859013, 18.04229054158819423, -27.38248356850343512 ) ) ;
#9870=CARTESIAN_POINT ( 'NONE',  ( -17.97959330666300559, 18.28784316811839972, -9.349175424125363065 ) ) ;
#9873=AXIS2_PLACEMENT_3D ( 'NONE', #21247, #2569, #33657 ) ;
#9874=CARTESIAN_POINT ( 'NONE',  ( 9.960472199639074375, -18.81618559987053985, -25.01525443589214248 ) ) ;
#9876=CARTESIAN_POINT ( 'NONE',  ( 14.74364839002157979, 25.37821730288758459, -10.65361825091638615 ) ) ;
#9878=CARTESIAN_POINT ( 'NONE',  ( 15.33243761980678599, 26.63804497122816528, -6.887548222410910803 ) ) ;
#9881=CARTESIAN_POINT ( 'NONE',  ( -13.97427186057036863, -24.60121427642448921, -12.55298982698177390 ) ) ;
#9884=AXIS2_PLACEMENT_3D ( 'NONE', #5591, #2556, #22717 ) ;
#9885=CARTESIAN_POINT ( 'NONE',  ( -29.03261643272151815, -20.06036525406060633, -11.07436732675348523 ) ) ;
#9886=CARTESIAN_POINT ( 'NONE',  ( -1.996201064919716606, -21.64193600980604515, -21.17403543307457170 ) ) ;
#9887=CARTESIAN_POINT ( 'NONE',  ( 13.28169970595349803, 21.08631984670124027, -17.49495114793986161 ) ) ;
#9890=CARTESIAN_POINT ( 'NONE',  ( 19.72017037454142141, 9.080320345084325950, -21.16391035189845482 ) ) ;
#9894=CARTESIAN_POINT ( 'NONE',  ( -31.96359514549918757, -3.261425111024537582, -9.982721131112327839 ) ) ;
#9902=CARTESIAN_POINT ( 'NONE',  ( -20.42898406783283960, 2.211777317264515652, -28.75134568260269674 ) ) ;
#9903=CARTESIAN_POINT ( 'NONE',  ( 34.24928854971908976, -14.99804081630860608, -7.982871076175817926 ) ) ;
#9916=CARTESIAN_POINT ( 'NONE',  ( -0.4101013132653836823, 21.15020722337806447, -26.25491541755722480 ) ) ;
#9922=CARTESIAN_POINT ( 'NONE',  ( 11.66971972310407146, 25.75749872935682561, -15.14234555051886666 ) ) ;
#9925=CARTESIAN_POINT ( 'NONE',  ( -21.19257405417214812, 12.68336146040521761, -6.940464740854612735 ) ) ;
#9928=CARTESIAN_POINT ( 'NONE',  ( 10.00997369995331177, -18.79612801155203883, -25.00947302926656235 ) ) ;
#9930=CARTESIAN_POINT ( 'NONE',  ( 15.31424333055854170, 26.70176439337667773, -6.886156298975530277 ) ) ;
#9931=CARTESIAN_POINT ( 'NONE',  ( 19.54664213359407654, -11.28525909758385914, -30.00000000000003908 ) ) ;
#9934=CARTESIAN_POINT ( 'NONE',  ( -21.19775588263476251, -22.46636194237366269, -13.96214201008129763 ) ) ;
#9935=CARTESIAN_POINT ( 'NONE',  ( 6.152249614461454463, -24.82641286710474660, -8.379856565498640109 ) ) ;
#9936=CARTESIAN_POINT ( 'NONE',  ( 11.28733053642023698, 17.68149975644739058, -26.23582624851832534 ) ) ;
#9938=CARTESIAN_POINT ( 'NONE',  ( 17.85505465768944333, -12.86254080347576512, -24.24539029509336885 ) ) ;
#9942=CARTESIAN_POINT ( 'NONE',  ( -8.350843205241419653, 35.56854215007076903, -7.588859392928601011 ) ) ;
#9945=CARTESIAN_POINT ( 'NONE',  ( 22.22902049279901959, 0.6319665380888792594, -22.73092917304706972 ) ) ;
#9946=CARTESIAN_POINT ( 'NONE',  ( -3.465511072935358428, 38.21601825462828828, -5.000000000000000000 ) ) ;
#9949=CARTESIAN_POINT ( 'NONE',  ( -29.76070246994180479, 0.08935854291201565658, -9.710064343477942117 ) ) ;
#9953=CARTESIAN_POINT ( 'NONE',  ( 20.48269730678144995, -4.854230542895870748, -26.43053413679163555 ) ) ;
#9955=EDGE_LOOP ( 'NONE', ( #21237, #5705, #32790, #23349, #17257, #24327, #12684 ) ) ;
#9964=CARTESIAN_POINT ( 'NONE',  ( -18.68149877921488766, -8.466985313562505056, -30.00000000000001421 ) ) ;
#9968=CARTESIAN_POINT ( 'NONE',  ( 14.27219392008591292, 14.71651433334269043, -29.40509136628979547 ) ) ;
#9969=CARTESIAN_POINT ( 'NONE',  ( 8.657666503606854747, 33.55139795693855831, -10.25229396191044273 ) ) ;
#9972=CARTESIAN_POINT ( 'NONE',  ( 15.74238530928792201, -25.84026302488051385, -10.12512499451556813 ) ) ;
#9976=CARTESIAN_POINT ( 'NONE',  ( -15.41471391286399317, 26.78795929021520550, -5.000000000000001776 ) ) ;
#9979=CARTESIAN_POINT ( 'NONE',  ( 14.19115657440825728, -25.54240891117661860, -10.19065319804806258 ) ) ;
#9983=CARTESIAN_POINT ( 'NONE',  ( -8.291215257814828377, 18.82905498736118588, -28.59874454941313360 ) ) ;
#9987=CARTESIAN_POINT ( 'NONE',  ( -28.12294647621138921, -8.736892962676476415, -15.78945194607744895 ) ) ;
#9990=CARTESIAN_POINT ( 'NONE',  ( 20.60369210407207063, 0.9606588650137843910, -28.08297012610058019 ) ) ;
#9995=CARTESIAN_POINT ( 'NONE',  ( -21.71849452838645789, 0.6790819573452312463, -23.84809452429628607 ) ) ;
#9997=CARTESIAN_POINT ( 'NONE',  ( 25.83202993258364089, -0.8389207943029072245, -17.28593405758972779 ) ) ;
#10014=CARTESIAN_POINT ( 'NONE',  ( -19.34217367975503876, 7.121619937563573366, -27.70688438477295179 ) ) ;
#10016=CARTESIAN_POINT ( 'NONE',  ( 15.00527517599701710, -17.60829065308229247, -22.19583011995415589 ) ) ;
#10018=CARTESIAN_POINT ( 'NONE',  ( 11.04596197333746055, 17.85565203605465001, -26.20988823588121619 ) ) ;
#10021=CARTESIAN_POINT ( 'NONE',  ( -15.22570016247339808, 24.01659300293151489, -10.68444636275925141 ) ) ;
#10024=CARTESIAN_POINT ( 'NONE',  ( 14.05306866902358820, 23.88062157653425643, -13.51576454616971645 ) ) ;
#10026=CARTESIAN_POINT ( 'NONE',  ( 27.88439565352735272, -14.28169649418448728, -14.73373279294286498 ) ) ;
#10029=CARTESIAN_POINT ( 'NONE',  ( -15.05229008872046670, 26.98958926311531670, -7.808750500632839930 ) ) ;
#10031=CARTESIAN_POINT ( 'NONE',  ( -12.83236629447386079, -21.40442163443030310, -18.34045313207591832 ) ) ;
#10034=CARTESIAN_POINT ( 'NONE',  ( -21.35353645564259750, -10.38814595318204326, -21.85098217641707308 ) ) ;
#10035=CARTESIAN_POINT ( 'NONE',  ( -9.453848434180018856, -19.01651734649589898, -25.07122770737407080 ) ) ;
#10037=CARTESIAN_POINT ( 'NONE',  ( 15.79381377564608613, 22.93146731034228480, -10.23294722842091353 ) ) ;
#10039=CARTESIAN_POINT ( 'NONE',  ( 24.48878357941496375, 5.471706907836950684, -12.77386761934589288 ) ) ;
#10046=CARTESIAN_POINT ( 'NONE',  ( -30.14783002406086609, -0.3420316433952748647, -9.682860013783926689 ) ) ;
#10048=CARTESIAN_POINT ( 'NONE',  ( 30.85995981617431028, -0.2746738912069357497, -7.348642656983717991 ) ) ;
#10052=CARTESIAN_POINT ( 'NONE',  ( 7.289639608743135213, -27.06962010326278190, -5.000000000000004441 ) ) ;
#10054=ORIENTED_EDGE ( 'NONE', *, *, #17470, .F. ) ;
#10058=CARTESIAN_POINT ( 'NONE',  ( 19.07667540469735101, 16.81475038977109548, -5.000000000000001776 ) ) ;
#10059=CARTESIAN_POINT ( 'NONE',  ( 2.790657799059328426, 21.23657145591617379, -25.61566959286999179 ) ) ;
#10060=FACE_BOUND ( 'NONE', #21032, .T. ) ;
#10064=CARTESIAN_POINT ( 'NONE',  ( 29.26826387686844910, -23.91120845623157010, -5.000000000000000888 ) ) ;
#10069=CARTESIAN_POINT ( 'NONE',  ( 10.76512838780859660, 18.45021222265605232, -24.94022975695240874 ) ) ;
#10072=CARTESIAN_POINT ( 'NONE',  ( -15.67910400704473517, 18.03213292446707783, -16.76744236533109245 ) ) ;
#10075=CARTESIAN_POINT ( 'NONE',  ( 12.99182960350822214, -23.09069332813563946, -15.45185403630547150 ) ) ;
#10077=CARTESIAN_POINT ( 'NONE',  ( 14.84680087938761872, 25.58880802702974933, -10.18073488593564413 ) ) ;
#10079=CARTESIAN_POINT ( 'NONE',  ( 14.52843121217837030, 24.98140828273265157, -11.59866322938457728 ) ) ;
#10083=CARTESIAN_POINT ( 'NONE',  ( -13.70756163817629414, -24.11668832361970161, -13.51384470570144458 ) ) ;
#10087=CARTESIAN_POINT ( 'NONE',  ( -23.30856450506559341, -17.15677614324469502, -16.65319078585623913 ) ) ;
#10088=CARTESIAN_POINT ( 'NONE',  ( -2.199171785053767980, -22.69879091448489916, -16.97731724952892662 ) ) ;
#10089=CARTESIAN_POINT ( 'NONE',  ( 12.45205971826092473, 19.54394706486126054, -20.59674335405842882 ) ) ;
#10091=CARTESIAN_POINT ( 'NONE',  ( 18.28802337575010384, 9.378636759438260029, -28.29756235655922225 ) ) ;
#10092=CARTESIAN_POINT ( 'NONE',  ( 35.48557158694710978, -12.46552367096746217, -4.999999999999999112 ) ) ;
#10095=CARTESIAN_POINT ( 'NONE',  ( -33.12478769974119786, -4.346059658142014115, -8.586455447396705409 ) ) ;
#10100=PLANE ( 'NONE',  #13494 ) ;
#10101=CARTESIAN_POINT ( 'NONE',  ( 22.52679405684453329, -9.890575151869189341, -20.72956160231121103 ) ) ;
#10114=CARTESIAN_POINT ( 'NONE',  ( -1.894380261295754098, 37.63992458223975746, -7.973046867981261165 ) ) ;
#10121=CARTESIAN_POINT ( 'NONE',  ( 9.285927727562647505, 18.34037923570121009, -28.63677830487614528 ) ) ;
#10125=CARTESIAN_POINT ( 'NONE',  ( -18.22877391798860458, 10.85510818490154250, -23.33390808761037860 ) ) ;
#10128=CARTESIAN_POINT ( 'NONE',  ( 14.09698363156053524, -24.62026783164278498, -12.54657184365754752 ) ) ;
#10130=CARTESIAN_POINT ( 'NONE',  ( 10.94214493613176664, 17.33550160327741096, -29.34744205922653393 ) ) ;
#10131=CARTESIAN_POINT ( 'NONE',  ( -19.79815887584811307, 19.84782313723621883, -4.999999999999999112 ) ) ;
#10133=CARTESIAN_POINT ( 'NONE',  ( -19.86385295935389550, -21.04324079092269173, -15.86974588982537782 ) ) ;
#10134=CARTESIAN_POINT ( 'NONE',  ( 7.644341925271119997, -20.35065011595537499, -23.04646567544028812 ) ) ;
#10135=CARTESIAN_POINT ( 'NONE',  ( 11.40938548045612499, 17.96021580865084744, -25.02785325939463235 ) ) ;
#10136=CARTESIAN_POINT ( 'NONE',  ( 20.81850934979185652, -15.01608711947214481, -19.65698525133124264 ) ) ;
#10141=CARTESIAN_POINT ( 'NONE',  ( -8.279978381213238592, 30.99040824897319979, -13.00426055310639839 ) ) ;
#10148=CARTESIAN_POINT ( 'NONE',  ( 25.22159695029489512, 0.3595918362293377135, -17.43676678839515759 ) ) ;
#10153=CARTESIAN_POINT ( 'NONE',  ( -28.21771817255893566, 0.2928912805552565390, -12.55734437234891132 ) ) ;
#10154=CARTESIAN_POINT ( 'NONE',  ( -19.35675341420076023, -25.73740943626670585, -10.41501234953343946 ) ) ;
#10156=CARTESIAN_POINT ( 'NONE',  ( 35.24432775889728475, -8.480040233932975013, -5.000000000000009770 ) ) ;
#10166=EDGE_CURVE ( 'NONE', #15787, #19280, #330, .T. ) ;
#10167=( NAMED_UNIT ( * ) SI_UNIT ( $, .STERADIAN. ) SOLID_ANGLE_UNIT ( ) );
#10168=CARTESIAN_POINT ( 'NONE',  ( 10.98647152928294446, 17.30743895948372213, -29.99999999999999289 ) ) ;
#10171=CARTESIAN_POINT ( 'NONE',  ( 16.91443829427942092, 17.27418336307699320, -14.80451719960429102 ) ) ;
#10172=AXIS2_PLACEMENT_3D ( 'NONE', #36485, #15145, #36089 ) ;
#10173=CARTESIAN_POINT ( 'NONE',  ( 6.063091157267137099, 20.95441350364335875, -24.44308551677271879 ) ) ;
#10176=CARTESIAN_POINT ( 'NONE',  ( 11.03529696084846456, -19.42597325127027830, -22.66960005987283466 ) ) ;
#10180=CARTESIAN_POINT ( 'NONE',  ( -11.19888719761758722, 17.74582991396291831, -26.22643622722658563 ) ) ;
#10182=CARTESIAN_POINT ( 'NONE',  ( 9.268250591559597851, -18.42220998856590697, -28.09379604205451741 ) ) ;
#10184=ORIENTED_EDGE ( 'NONE', *, *, #7842, .F. ) ;
#10186=CARTESIAN_POINT ( 'NONE',  ( -8.267738057345434655, 18.77097771606736032, -29.99999999999997868 ) ) ;
#10187=DIRECTION ( 'NONE',  ( -1.000000000000000000, 0.000000000000000000, 0.000000000000000000 ) ) ;
#10189=CARTESIAN_POINT ( 'NONE',  ( -34.15174964376215883, -8.447579901654981072, -8.931880151306236471 ) ) ;
#10192=CARTESIAN_POINT ( 'NONE',  ( 27.01856200969307054, 0.4099118485097461573, -14.48824044023039015 ) ) ;
#10196=CARTESIAN_POINT ( 'NONE',  ( -29.80962035732523674, 0.03519742696252582681, -9.709001665780544243 ) ) ;
#10199=CARTESIAN_POINT ( 'NONE',  ( 31.72491548083144508, -2.179369429322845164, -9.120202422530157449 ) ) ;
#10201=CARTESIAN_POINT ( 'NONE',  ( 19.79988521532547807, 5.489632757569235189, -30.00000000000001421 ) ) ;
#10205=CARTESIAN_POINT ( 'NONE',  ( 37.48557158514988430, -11.25000000000009237, 3.000000000000000000 ) ) ;
#10212=CARTESIAN_POINT ( 'NONE',  ( -22.92528781977826569, 9.871412332755808094, -6.451104567815622914 ) ) ;
#10213=CARTESIAN_POINT ( 'NONE',  ( 14.50529647024089286, -17.03828888122068363, -23.33609894585849531 ) ) ;
#10214=CARTESIAN_POINT ( 'NONE',  ( -22.57773860910944919, -27.07565175416711512, -4.999999999999999112 ) ) ;
#10215=CARTESIAN_POINT ( 'NONE',  ( 10.93330143339572125, 17.49474783767401220, -28.07104482051876815 ) ) ;
#10218=CARTESIAN_POINT ( 'NONE',  ( -14.60464479478044808, 23.69115059860245864, -12.58079236048715188 ) ) ;
#10222=CARTESIAN_POINT ( 'NONE',  ( 15.25363860433223806, 26.33374284506462715, -7.828164261976985117 ) ) ;
#10224=CARTESIAN_POINT ( 'NONE',  ( 20.31494021939268535, -10.42483993722323454, -22.98956373470440440 ) ) ;
#10227=CARTESIAN_POINT ( 'NONE',  ( -14.65523368257949066, 26.15792607398499570, -10.14769008996043986 ) ) ;
#10229=CARTESIAN_POINT ( 'NONE',  ( -15.03157439599174694, -25.19314163198803769, -11.55082534625164037 ) ) ;
#10232=ORIENTED_EDGE ( 'NONE', *, *, #39941, .F. ) ;
#10233=CARTESIAN_POINT ( 'NONE',  ( -31.52559900738557985, -12.98691925735731978, -11.99846548842175586 ) ) ;
#10234=CARTESIAN_POINT ( 'NONE',  ( -12.90570201017717267, -24.02570373875013843, -13.54976151863601785 ) ) ;
#10236=CARTESIAN_POINT ( 'NONE',  ( 14.11158459539261401, 18.94724806458638255, -18.68180965987205866 ) ) ;
#10238=CARTESIAN_POINT ( 'NONE',  ( 20.01208193039519756, 4.507116686654150328, -29.40064677792853232 ) ) ;
#10243=CARTESIAN_POINT ( 'NONE',  ( -30.98040994848943086, -0.4068539715029224624, -7.344088399820972057 ) ) ;
#10244=CARTESIAN_POINT ( 'NONE',  ( 30.98810501497172964, -0.5565724573307553324, -7.804721584860615735 ) ) ;
#10245=ADVANCED_FACE ( 'NONE', ( #1793 ), #14176, .F. ) ;
#10250=CARTESIAN_POINT ( 'NONE',  ( 17.81784622497951176, -13.85677843414110555, -30.00000000000001421 ) ) ;
#10264=CARTESIAN_POINT ( 'NONE',  ( 23.83838753405464317, -22.06766206393824703, -12.96906389866784259 ) ) ;
#10267=CARTESIAN_POINT ( 'NONE',  ( 14.07479620741808191, 25.02281174304687639, -12.50432048929940976 ) ) ;
#10269=ORIENTED_EDGE ( 'NONE', *, *, #32149, .F. ) ;
#10270=CARTESIAN_POINT ( 'NONE',  ( -16.58243014776942204, 17.87902810744316184, -14.77884403044956763 ) ) ;
#10273=CARTESIAN_POINT ( 'NONE',  ( 14.94392118707002126, -25.98235010733188588, -9.238761082775399203 ) ) ;
#10275=CARTESIAN_POINT ( 'NONE',  ( 12.93407688617792495, 21.64341771708264517, -17.43892928429220035 ) ) ;
#10277=CARTESIAN_POINT ( 'NONE',  ( 15.01557101168928909, 25.97699093630907541, -9.238213213168704030 ) ) ;
#10279=CARTESIAN_POINT ( 'NONE',  ( -14.50572258746885623, 25.04706427101906741, -11.59331239428562021 ) ) ;
#10281=CARTESIAN_POINT ( 'NONE',  ( -15.03457768504921610, -26.13549839691439658, -8.768128526806304279 ) ) ;
#10284=CARTESIAN_POINT ( 'NONE',  ( -20.67042552518347875, -15.19177032836172003, -19.66260926008852650 ) ) ;
#10285=CARTESIAN_POINT ( 'NONE',  ( -2.438111228425578592, -23.95987689082008743, -11.87913270965556123 ) ) ;
#10286=CARTESIAN_POINT ( 'NONE',  ( 11.33961468246317139, 17.07831742606941461, -30.00000000000000000 ) ) ;
#10288=CARTESIAN_POINT ( 'NONE',  ( 23.89591241149270218, 8.281799400457325433, -7.415685632315970999 ) ) ;
#10289=CARTESIAN_POINT ( 'NONE',  ( 32.65693615964542573, -20.41475057477927280, -4.999999999999999112 ) ) ;
#10294=CARTESIAN_POINT ( 'NONE',  ( -24.11176595098584841, -2.272178682370984415, -20.18870583158593490 ) ) ;
#10301=CARTESIAN_POINT ( 'NONE',  ( 23.73065287294122783, -9.570089218292375577, -19.68554350756277671 ) ) ;
#10311=CARTESIAN_POINT ( 'NONE',  ( -1.918774233022853437, 38.27677537973431043, -6.276859307182877323 ) ) ;
#10313=FACE_OUTER_BOUND ( 'NONE', #28838, .T. ) ;
#10319=CARTESIAN_POINT ( 'NONE',  ( 10.10147183288163220, 20.27820810593225076, -22.48066845728959251 ) ) ;
#10320=CARTESIAN_POINT ( 'NONE',  ( 16.00000000000000000, 22.50000000000000711, 6.000000000000000000 ) ) ;
#10322=CARTESIAN_POINT ( 'NONE',  ( -16.91065988350933935, 11.83293620019187919, -27.16773465279506894 ) ) ;
#10325=CARTESIAN_POINT ( 'NONE',  ( 9.596601641187952225, -18.16644679415211172, -28.70396621286603533 ) ) ;
#10328=CARTESIAN_POINT ( 'NONE',  ( 15.08754104065838497, 26.18438373079535708, -8.765583629728475046 ) ) ;
#10329=CARTESIAN_POINT ( 'NONE',  ( -22.45323650136969462, -2.382502413133420038, -30.00000000000000000 ) ) ;
#10331=CARTESIAN_POINT ( 'NONE',  ( -19.21792407943181757, -19.17370927486487275, -17.77733382730791334 ) ) ;
#10332=CARTESIAN_POINT ( 'NONE',  ( 5.642336087577458414, -23.56041604079663898, -13.82695612366311266 ) ) ;
#10333=CARTESIAN_POINT ( 'NONE',  ( 11.58115104542198637, 18.35365690391862614, -23.86862541693199802 ) ) ;
#10334=CARTESIAN_POINT ( 'NONE',  ( 30.18028009888747221, -21.81123660786073870, -8.413970242988657589 ) ) ;
#10338=CARTESIAN_POINT ( 'NONE',  ( -5.356379776258165748, 22.86463390630803261, -22.00052314567535561 ) ) ;
#10344=CARTESIAN_POINT ( 'NONE',  ( 20.97320688508112596, 0.7727878754155812491, -26.22179187276591961 ) ) ;
#10347=EDGE_CURVE ( 'NONE', #21571, #31788, #25604, .T. ) ;
#10352=CARTESIAN_POINT ( 'NONE',  ( -27.07907469388687716, 0.3230542143888946449, -14.48244227824745245 ) ) ;
#10355=CARTESIAN_POINT ( 'NONE',  ( 31.01063626114513738, -8.317636515201035863, -13.00212388364185223 ) ) ;
#10367=ADVANCED_FACE ( 'NONE', ( #33686 ), #21669, .T. ) ;
#10370=CARTESIAN_POINT ( 'NONE',  ( 13.82201771817531544, 15.33810796475532356, -27.62586602732605101 ) ) ;
#10371=CARTESIAN_POINT ( 'NONE',  ( 8.507170864035593638, 26.45108214636019639, -16.86777324031742253 ) ) ;
#10376=CARTESIAN_POINT ( 'NONE',  ( 16.02147964071269115, -26.56717389092953852, -7.803345548162054612 ) ) ;
#10380=CARTESIAN_POINT ( 'NONE',  ( -13.77848933305083712, 23.37701899211078072, -14.47715019980521411 ) ) ;
#10382=CARTESIAN_POINT ( 'NONE',  ( 13.20637083253811461, -24.05908822848580897, -13.53613500056979291 ) ) ;
#10385=ORIENTED_EDGE ( 'NONE', *, *, #31204, .F. ) ;
#10386=CARTESIAN_POINT ( 'NONE',  ( -8.874894838237054273, 18.54570556417430538, -28.62091128729561973 ) ) ;
#10391=CARTESIAN_POINT ( 'NONE',  ( -33.05153516003798586, -7.169066213692435241, -10.30292366904723700 ) ) ;
#10394=CARTESIAN_POINT ( 'NONE',  ( 30.81169820973430973, 0.05224243800113868852, -5.474171594225969883 ) ) ;
#10395=ADVANCED_FACE ( 'NONE', ( #24519 ), #36922, .F. ) ;
#10399=CARTESIAN_POINT ( 'NONE',  ( -20.52752421040557351, 0.8457101814844484311, -28.70654326211919027 ) ) ;
#10403=CARTESIAN_POINT ( 'NONE',  ( 20.47947323059178260, -0.9304062671392134831, -30.00000000000000000 ) ) ;
#10405=CARTESIAN_POINT ( 'NONE',  ( 18.58489934068024141, 8.677531291371142430, -30.00000000000000355 ) ) ;
#10417=CARTESIAN_POINT ( 'NONE',  ( -20.06104095114847041, 7.248907926436412019, -23.26760403684622602 ) ) ;
#10418=CARTESIAN_POINT ( 'NONE',  ( 21.07929656120333917, -26.04002531597158310, -9.455788634464944664 ) ) ;
#10421=CARTESIAN_POINT ( 'NONE',  ( 12.01797261908369840, 20.05841915129454733, -20.51811533202489102 ) ) ;
#10423=CARTESIAN_POINT ( 'NONE',  ( -15.74234945116950790, 25.02555085579499305, -7.363867029611805393 ) ) ;
#10426=CARTESIAN_POINT ( 'NONE',  ( 14.86957149986643145, 25.52042674580396309, -10.18200345931521866 ) ) ;
#10428=CARTESIAN_POINT ( 'NONE',  ( 33.57338286677032357, -18.51555322403216053, -6.276315919122906983 ) ) ;
#10432=CARTESIAN_POINT ( 'NONE',  ( -10.88717731418932289, 17.62612854685823649, -27.43333487934502557 ) ) ;
#10434=CARTESIAN_POINT ( 'NONE',  ( -15.89382728895068553, -26.44918619828455775, -8.270623719106945160 ) ) ;
#10437=CARTESIAN_POINT ( 'NONE',  ( -33.03998026049733028, -13.61677984810819275, -10.19367267226056484 ) ) ;
#10438=CARTESIAN_POINT ( 'NONE',  ( -9.521033199116716972, -19.40341469932255691, -23.93640817374758711 ) ) ;
#10440=CARTESIAN_POINT ( 'NONE',  ( 15.98076197519813668, 18.99300102774612498, -14.72676035881280043 ) ) ;
#10442=CARTESIAN_POINT ( 'NONE',  ( 26.35545874991313653, 3.770332275510887232, -10.75732149805491034 ) ) ;
#10447=CARTESIAN_POINT ( 'NONE',  ( -21.74228451847596588, 0.5523326501866797633, -23.83255557727324714 ) ) ;
#10448=CARTESIAN_POINT ( 'NONE',  ( 31.38436285448675989, -0.5902540978377334158, -5.938636948564323781 ) ) ;
#10451=AXIS2_PLACEMENT_3D ( 'NONE', #23999, #33762, #18310 ) ;
#10453=CARTESIAN_POINT ( 'NONE',  ( 6.023418944065099367, 39.81932404830325112, -4.999999999999995559 ) ) ;
#10455=DIRECTION ( 'NONE',  ( -0.000000000000000000, -0.000000000000000000, 1.000000000000000000 ) ) ;
#10465=CARTESIAN_POINT ( 'NONE',  ( 28.23631333451608683, -24.52731714411232744, -6.292009388830251737 ) ) ;
#10468=CARTESIAN_POINT ( 'NONE',  ( 15.18041152575273500, 27.55477496851653640, -5.000000000000000000 ) ) ;
#10472=CARTESIAN_POINT ( 'NONE',  ( -17.83076603928403969, 19.73132804355285685, -5.477525253067689448 ) ) ;
#10475=CARTESIAN_POINT ( 'NONE',  ( 13.36832410447146380, -23.62212012520782523, -14.47646263800011113 ) ) ;
#10478=CARTESIAN_POINT ( 'NONE',  ( 11.05197910185074583, 17.41712326167257885, -28.07812360280739838 ) ) ;
#10480=CARTESIAN_POINT ( 'NONE',  ( 14.93249212465000397, 25.80697923307498698, -9.708869224783416740 ) ) ;
#10482=CARTESIAN_POINT ( 'NONE',  ( -10.97676730033676407, 17.36694328198177573, -28.70573505724077989 ) ) ;
#10484=CARTESIAN_POINT ( 'NONE',  ( -15.12588299545583403, -26.27105592520571520, -8.298080420248476585 ) ) ;
#10486=CARTESIAN_POINT ( 'NONE',  ( -16.96436027188408602, -11.67839957979620280, -28.44978934027107087 ) ) ;
#10487=CARTESIAN_POINT ( 'NONE',  ( -3.323560782785250911, -20.43354657522463214, -27.15214811866635358 ) ) ;
#10488=CARTESIAN_POINT ( 'NONE',  ( 15.30101822393199029, 24.69709018996960737, -9.726406352004691058 ) ) ;
#10490=CARTESIAN_POINT ( 'NONE',  ( 19.25042232574495671, 7.324643854277566923, -27.70922511033380076 ) ) ;
#10497=CARTESIAN_POINT ( 'NONE',  ( -27.02112178989742119, -1.880880936477675069, -16.19440878182897237 ) ) ;
#10503=CARTESIAN_POINT ( 'NONE',  ( 33.50338741967450318, -14.65902325991027411, -9.295247887544057619 ) ) ;
#10508=CARTESIAN_POINT ( 'NONE',  ( -15.58309971386584536, 26.19172985869298742, -5.000000000000001776 ) ) ;
#10511=CARTESIAN_POINT ( 'NONE',  ( -1.824030652502988792, 36.09425736751438052, -10.17475919037218546 ) ) ;
#10518=CARTESIAN_POINT ( 'NONE',  ( 9.787798997179907090, 18.68458674667809660, -26.07733087769958047 ) ) ;
#10521=AXIS2_PLACEMENT_3D ( 'NONE', #16337, #7381, #1100 ) ;
#10522=CARTESIAN_POINT ( 'NONE',  ( -17.23503577783534624, 11.12556197759191967, -29.42916173689316039 ) ) ;
#10524=EDGE_CURVE ( 'NONE', #19243, #31932, #7452, .T. ) ;
#10526=CARTESIAN_POINT ( 'NONE',  ( 14.42086957103650668, -25.08249617576892732, -11.59459791273149065 ) ) ;
#10529=CARTESIAN_POINT ( 'NONE',  ( 13.18496159700378811, 22.28102628015067666, -16.43839240474340713 ) ) ;
#10530=CARTESIAN_POINT ( 'NONE',  ( -3.091399026088746727, 22.35909668862748134, -19.80438750953544513 ) ) ;
#10532=CARTESIAN_POINT ( 'NONE',  ( -27.61224229448858836, -24.44226837637327421, -7.577694500159308788 ) ) ;
#10534=CARTESIAN_POINT ( 'NONE',  ( 6.261531442577396689, -25.09448364857072633, -5.000000000000002665 ) ) ;
#10535=CARTESIAN_POINT ( 'NONE',  ( 14.12972245875639032, 23.70285533380211263, -13.52451117403163217 ) ) ;
#10537=CARTESIAN_POINT ( 'NONE',  ( 19.31783821962531533, 13.01333379127007817, -14.91341792948933787 ) ) ;
#10541=CARTESIAN_POINT ( 'NONE',  ( -8.213440145680040771, 34.88663893459818155, -8.900416981694739604 ) ) ;
#10543=CARTESIAN_POINT ( 'NONE',  ( -14.92561699251189999, -26.11061048198896017, -8.769174845341428437 ) ) ;
#10546=CARTESIAN_POINT ( 'NONE',  ( 30.94149296799522020, -0.08026563842153495998, -5.473949085746474097 ) ) ;
#10553=CARTESIAN_POINT ( 'NONE',  ( -20.96089682640939600, 0.8916499400121695729, -26.23216352804135099 ) ) ;
#10555=CARTESIAN_POINT ( 'NONE',  ( 35.07953814774953827, -9.478878833152338146, -7.167510118368202399 ) ) ;
#10570=CARTESIAN_POINT ( 'NONE',  ( 14.83043047287890559, 14.27182183044933694, -28.25080419411967725 ) ) ;
#10572=CARTESIAN_POINT ( 'NONE',  ( 9.099779625626309709, 28.28310968578335505, -14.93302891365372886 ) ) ;
#10577=CARTESIAN_POINT ( 'NONE',  ( 15.87182004195441110, -26.02674557003009426, -9.657777150000830702 ) ) ;
#10581=CARTESIAN_POINT ( 'NONE',  ( -12.93600697479300621, 21.64018247274085027, -17.43937243684336735 ) ) ;
#10584=CARTESIAN_POINT ( 'NONE',  ( 9.344739644993655503, -18.38529687660023271, -28.08976026156862105 ) ) ;
#10588=CARTESIAN_POINT ( 'NONE',  ( -8.438355134513948030, 19.20186035763207855, -26.59191105792285015 ) ) ;
#10589=CARTESIAN_POINT ( 'NONE',  ( -18.98517869367844924, -25.27528659947290990, -11.33194675744996971 ) ) ;
#10592=CARTESIAN_POINT ( 'NONE',  ( -19.91373213366430761, -4.906168661338282888, -29.99999999999999645 ) ) ;
#10596=CARTESIAN_POINT ( 'NONE',  ( 20.95770388837388865, 0.9215809845027531644, -26.23473912195051838 ) ) ;
#10597=CARTESIAN_POINT ( 'NONE',  ( 13.76592227337845209, 23.41050468301912346, -14.45573797668741634 ) ) ;
#10600=CARTESIAN_POINT ( 'NONE',  ( -25.21984550008777148, 0.3633275739477161981, -17.43674445742407997 ) ) ;
#10602=ORIENTED_EDGE ( 'NONE', *, *, #12309, .F. ) ;
#10604=CARTESIAN_POINT ( 'NONE',  ( 33.84582931909603332, -4.187585590875373853, -5.904510056914596738 ) ) ;
#10605=VECTOR ( 'NONE', #7445, 1000.000000000000000 ) ;
#10606=CARTESIAN_POINT ( 'NONE',  ( 13.96856925441951880, 15.00887706487568352, -30.00000000000001066 ) ) ;
#10621=CARTESIAN_POINT ( 'NONE',  ( -19.47111235004281937, 7.144292970305836654, -26.58057671234093888 ) ) ;
#10622=CARTESIAN_POINT ( 'NONE',  ( 19.81334941875573108, -24.54698869046120535, -12.19926732474853814 ) ) ;
#10623=CARTESIAN_POINT ( 'NONE',  ( -32.54675706181794936, -20.70611888103728049, -4.999999999999999112 ) ) ;
#10624=CARTESIAN_POINT ( 'NONE',  ( 11.34939637619692121, 18.55308824603512363, -23.83256028268874260 ) ) ;
#10627=CARTESIAN_POINT ( 'NONE',  ( -15.81425778636113755, 25.16710388755963024, -6.419180666290403181 ) ) ;
#10631=CARTESIAN_POINT ( 'NONE',  ( 11.34936283256858225, 18.00731010319261927, -25.01985386284653146 ) ) ;
#10633=CARTESIAN_POINT ( 'NONE',  ( 18.16597811475082835, -10.02368442138252114, -27.70584967217684280 ) ) ;
#10636=CARTESIAN_POINT ( 'NONE',  ( -15.22095580511879120, 27.34682230800605751, -5.939933693853666874 ) ) ;
#10638=CARTESIAN_POINT ( 'NONE',  ( -16.64260134343204101, -26.86770968575480012, -6.862158467649761562 ) ) ;
#10642=CARTESIAN_POINT ( 'NONE',  ( -35.33747858074038817, -13.37758297739395452, -5.862854311016519659 ) ) ;
#10643=CARTESIAN_POINT ( 'NONE',  ( -14.73998792673631542, -26.43434547851132166, -6.889327648708172269 ) ) ;
#10645=CARTESIAN_POINT ( 'NONE',  ( 15.31670499384548023, 17.89843587122107493, -17.77664689643157558 ) ) ;
#10647=CARTESIAN_POINT ( 'NONE',  ( 20.04042991074784652, 4.507464788493477315, -28.80730530478267681 ) ) ;
#10652=CARTESIAN_POINT ( 'NONE',  ( -25.35686378040836075, 0.1132805088522348264, -17.40355568153567134 ) ) ;
#10654=CARTESIAN_POINT ( 'NONE',  ( 20.83961557846457424, 0.5176935620071271282, -26.80626269608042023 ) ) ;
#10658=CARTESIAN_POINT ( 'NONE',  ( -26.53302367738332279, 1.838442054519318525, -13.60518866641464442 ) ) ;
#10659=CARTESIAN_POINT ( 'NONE',  ( -15.29245034862075769, 32.56469986091995850, -4.999999999999987566 ) ) ;
#10672=CARTESIAN_POINT ( 'NONE',  ( 18.46250793368027487, -16.02721248873823612, -20.80436923686731632 ) ) ;
#10675=CARTESIAN_POINT ( 'NONE',  ( 12.32516380029041159, 21.52845440364069063, -18.38234602673094287 ) ) ;
#10678=CARTESIAN_POINT ( 'NONE',  ( -17.03554767930629410, 20.20091378400016424, -9.804406882113656962 ) ) ;
#10680=CARTESIAN_POINT ( 'NONE',  ( 15.33814677726094189, -26.70409432335911859, -5.474165994462620866 ) ) ;
#10682=CARTESIAN_POINT ( 'NONE',  ( 14.29780702217399657, 24.45410663696299736, -12.55099008032420471 ) ) ;
#10684=CARTESIAN_POINT ( 'NONE',  ( 11.30219353822485395, 18.04414504934459984, -25.01352393563159282 ) ) ;
#10686=CARTESIAN_POINT ( 'NONE',  ( -13.72666537043441615, 23.49252283158499921, -14.46614592794059284 ) ) ;
#10688=CARTESIAN_POINT ( 'NONE',  ( -10.80461807628140392, -19.99823691242070467, -21.62132452699231422 ) ) ;
#10691=CARTESIAN_POINT ( 'NONE',  ( -29.53691847232408918, -17.84505293552917493, -11.97318411411579575 ) ) ;
#10692=CARTESIAN_POINT ( 'NONE',  ( -9.209455750247457217, -25.27647548880431216, -7.390589557538877585 ) ) ;
#10693=CARTESIAN_POINT ( 'NONE',  ( 15.55043953303557380, 24.72954629399698590, -8.782262712390135562 ) ) ;
#10695=CARTESIAN_POINT ( 'NONE',  ( 23.51665520216067051, 8.202378042728126317, -9.863491397679609918 ) ) ;
#10696=CARTESIAN_POINT ( 'NONE',  ( 23.90699799611010334, -26.67493067552189601, -4.999999999999999112 ) ) ;
#10701=CARTESIAN_POINT ( 'NONE',  ( -31.30770620205629129, -1.570573974800437700, -9.148545248552471421 ) ) ;
#10703=ORIENTED_EDGE ( 'NONE', *, *, #16004, .T. ) ;
#10704=FACE_OUTER_BOUND ( 'NONE', #25092, .T. ) ;
#10708=CARTESIAN_POINT ( 'NONE',  ( 32.17432900182389943, -14.06792078237634414, -11.08295527558030180 ) ) ;
#10716=CARTESIAN_POINT ( 'NONE',  ( -0.7281348173785022748, 36.90684702921205940, -9.281235812587201650 ) ) ;
#10717=DIRECTION ( 'NONE',  ( 0.000000000000000000, 0.000000000000000000, 1.000000000000000000 ) ) ;
#10718=DIRECTION ( 'NONE',  ( -0.000000000000000000, -0.000000000000000000, 1.000000000000000000 ) ) ;
#10723=CARTESIAN_POINT ( 'NONE',  ( 13.74729660097108663, 28.63478031050133410, -9.567228944388832090 ) ) ;
#10727=CARTESIAN_POINT ( 'NONE',  ( -20.16920377049624591, 14.63653134085040541, -6.451392141180062545 ) ) ;
#10731=CARTESIAN_POINT ( 'NONE',  ( 15.49955545918230548, -26.71975771321320181, -5.945739302876239307 ) ) ;
#10733=CARTESIAN_POINT ( 'NONE',  ( 14.51660510353637257, 25.01588927535994955, -11.59567232272055470 ) ) ;
#10734=CARTESIAN_POINT ( 'NONE',  ( -35.84808252048276955, -3.038699442442197807, -13.99876745781545218 ) ) ;
#10736=CARTESIAN_POINT ( 'NONE',  ( -17.00128974941928917, -15.01612503178150071, -23.10570941354218633 ) ) ;
#10737=CARTESIAN_POINT ( 'NONE',  ( 7.126221445658505793, -19.51322017656814722, -27.01549118789370141 ) ) ;
#10738=CARTESIAN_POINT ( 'NONE',  ( 14.95545557393707092, 25.26472974152139983, -10.18678968210642566 ) ) ;
#10739=CARTESIAN_POINT ( 'NONE',  ( 17.11772138832456847, 11.31348593724026053, -28.86057714366049609 ) ) ;
#10743=CARTESIAN_POINT ( 'NONE',  ( -6.386588552221052595, 37.17016244130430636, -5.438612508982328286 ) ) ;
#10745=CARTESIAN_POINT ( 'NONE',  ( -13.90807750521352304, -24.59146351958235144, -12.55541049602243575 ) ) ;
#10753=CARTESIAN_POINT ( 'NONE',  ( -30.79543237407852985, 0.06882123448303990865, -5.474165231917279328 ) ) ;
#10755=CARTESIAN_POINT ( 'NONE',  ( 34.24879707383919936, -9.221469049884310820, -8.917830257142501438 ) ) ;
#10757=AXIS2_PLACEMENT_3D ( 'NONE', #34963, #4682, #16680 ) ;
#10767=DIRECTION ( 'NONE',  ( 0.000000000000000000, 0.000000000000000000, 1.000000000000000000 ) ) ;
#10768=DIRECTION ( 'NONE',  ( 1.000000000000000000, 0.000000000000000000, 0.000000000000000000 ) ) ;
#10771=CARTESIAN_POINT ( 'NONE',  ( 18.84172639249922909, 16.68708957390086312, -8.877532344250958829 ) ) ;
#10772=CARTESIAN_POINT ( 'NONE',  ( 6.542235822104545129, 20.26185204575804022, -25.79941729011566309 ) ) ;
#10778=CARTESIAN_POINT ( 'NONE',  ( 13.65807228238010573, -23.12680062072891118, -15.38534464500674659 ) ) ;
#10784=CARTESIAN_POINT ( 'NONE',  ( -11.11991152073464484, 17.61650879674641246, -26.82993365721759460 ) ) ;
#10787=CARTESIAN_POINT ( 'NONE',  ( 15.03800791059918396, -26.62802654356141119, -5.474101061827365555 ) ) ;
#10792=CARTESIAN_POINT ( 'NONE',  ( -10.94743835640653806, 25.45487626883825172, -16.07729632899789962 ) ) ;
#10795=CARTESIAN_POINT ( 'NONE',  ( -33.91433556152139062, -7.380049849088682556, -8.955366286169795131 ) ) ;
#10798=CARTESIAN_POINT ( 'NONE',  ( 20.51905432487639303, 1.011595284947182982, -28.71231566379986688 ) ) ;
#10799=CARTESIAN_POINT ( 'NONE',  ( -14.51034691152591805, -19.54383025136282725, -20.13759940192544562 ) ) ;
#10804=CARTESIAN_POINT ( 'NONE',  ( -21.71245050099948415, 0.7107615646682705624, -23.85198221761060822 ) ) ;
#10807=VERTEX_POINT ( 'NONE', #28025 ) ;
#10808=CARTESIAN_POINT ( 'NONE',  ( 32.87498921192744206, -3.141057219873002904, -7.719697989364024515 ) ) ;
#10820=CARTESIAN_POINT ( 'NONE',  ( 4.786734853113896904, 35.82772156925080509, -9.744462803125076178 ) ) ;
#10823=CARTESIAN_POINT ( 'NONE',  ( -19.17389268837527538, 8.645407496481396947, -24.39727980451651845 ) ) ;
#10824=ADVANCED_FACE ( 'NONE', ( #27624 ), #8745, .F. ) ;
#10825=CARTESIAN_POINT ( 'NONE',  ( 19.29636281975407641, -23.92107482882588698, -13.13705708359962898 ) ) ;
#10829=CARTESIAN_POINT ( 'NONE',  ( 13.71091892849755389, 23.52758077876742604, -14.46248064163161118 ) ) ;
#10831=CARTESIAN_POINT ( 'NONE',  ( -13.53743224670682110, 20.67868719046468939, -17.53536389037096299 ) ) ;
#10834=CARTESIAN_POINT ( 'NONE',  ( 11.53052341169412287, 18.39746216749503205, -23.86097604571838815 ) ) ;
#10836=CARTESIAN_POINT ( 'NONE',  ( 32.50613532488242896, -16.64577724727427466, -9.727483418184714736 ) ) ;
#10838=CARTESIAN_POINT ( 'NONE',  ( -11.45602697265520042, 19.13019776967873398, -22.69526440986508575 ) ) ;
#10840=CARTESIAN_POINT ( 'NONE',  ( -16.07798611810649092, -26.06690065413934221, -9.647245371388256885 ) ) ;
#10845=CARTESIAN_POINT ( 'NONE',  ( -34.43511996550268606, -14.21315942988885084, -7.987749063897047641 ) ) ;
#10846=CARTESIAN_POINT ( 'NONE',  ( -9.288332648570273520, -18.50011473801034612, -27.47095926884810169 ) ) ;
#10848=CARTESIAN_POINT ( 'NONE',  ( 13.37783513257456036, 15.99063134506573824, -26.42944179521041903 ) ) ;
#10849=VERTEX_POINT ( 'NONE', #30487 ) ;
#10850=CARTESIAN_POINT ( 'NONE',  ( 28.12338329411292648, 2.888959741955042571, -6.424895456845277408 ) ) ;
#10854=CARTESIAN_POINT ( 'NONE',  ( -30.80141499821036533, -0.2118792597572127512, -7.350865256546702753 ) ) ;
#10856=CARTESIAN_POINT ( 'NONE',  ( 22.29505466895832555, 0.3560692172932813371, -22.69527732140045728 ) ) ;
#10862=CARTESIAN_POINT ( 'NONE',  ( -24.38535528688051102, 1.937739723335398567, -17.58705028769485423 ) ) ;
#10863=CARTESIAN_POINT ( 'NONE',  ( -27.08779848459120743, 7.221796966026712283, -13.42901749168596481 ) ) ;
#10866=CARTESIAN_POINT ( 'NONE',  ( 17.34253826607186255, 27.32041144404028543, -5.000000000000000000 ) ) ;
#10869=DIRECTION ( 'NONE',  ( 0.000000000000000000, 0.000000000000000000, 1.000000000000000000 ) ) ;
#10873=CARTESIAN_POINT ( 'NONE',  ( -24.66395718121962233, 6.133371777919307100, -10.81519827307880277 ) ) ;
#10876=CARTESIAN_POINT ( 'NONE',  ( 26.18580253464329033, -24.21476188511185157, -9.337349200188750586 ) ) ;
#10883=CARTESIAN_POINT ( 'NONE',  ( 14.40939021871823300, 25.31363344341408350, -11.57339647497523671 ) ) ;
#10887=CARTESIAN_POINT ( 'NONE',  ( -17.31397306521514423, 20.64508075850899615, -7.389967135817093968 ) ) ;
#10889=CARTESIAN_POINT ( 'NONE',  ( 13.98758249977653634, -24.60317294295146695, -12.55250303098777032 ) ) ;
#10891=CARTESIAN_POINT ( 'NONE',  ( 15.40702647791744617, 26.72275646984359199, -5.946082907002145923 ) ) ;
#10893=CARTESIAN_POINT ( 'NONE',  ( 14.84111742463147010, 25.60591702902530997, -10.18041830445567442 ) ) ;
#10895=CARTESIAN_POINT ( 'NONE',  ( -13.17768508386178006, 22.29448265875752355, -16.43670467243796551 ) ) ;
#10897=CARTESIAN_POINT ( 'NONE',  ( -10.50283404165479162, -19.58549042586600919, -22.73910474386799407 ) ) ;
#10899=CARTESIAN_POINT ( 'NONE',  ( -32.47674537595472799, -19.61558511033160457, -7.544019131575042003 ) ) ;
#10900=CARTESIAN_POINT ( 'NONE',  ( -4.880576112647466935, -20.34275454070125733, -25.40727637649297677 ) ) ;
#10901=CARTESIAN_POINT ( 'NONE',  ( 11.81800289456031727, 17.11319857350586204, -26.89243828160074301 ) ) ;
#10903=CARTESIAN_POINT ( 'NONE',  ( 18.88780196539459055, 8.001059241770983377, -29.42544452779240416 ) ) ;
#10908=CARTESIAN_POINT ( 'NONE',  ( -32.83526622438716913, -2.536178072473608935, -6.372889071231118585 ) ) ;
#10919=CARTESIAN_POINT ( 'NONE',  ( 18.51815053109030629, -8.815588134695454769, -30.00000000000002487 ) ) ;
#10924=CARTESIAN_POINT ( 'NONE',  ( -14.98890121934610242, -28.67928442654176635, -5.000000000000000000 ) ) ;
#10927=CARTESIAN_POINT ( 'NONE',  ( 1.098729202488071710, 26.81952012603705526, -18.61434905906123305 ) ) ;
#10934=CARTESIAN_POINT ( 'NONE',  ( 9.649540945264268643, 19.20465645623720974, -24.79630837131278298 ) ) ;
#10938=CARTESIAN_POINT ( 'NONE',  ( -17.24968974221940599, 11.13640497999314150, -28.86202543690495759 ) ) ;
#10940=CARTESIAN_POINT ( 'NONE',  ( 12.30764836806737961, -22.02250499063774214, -17.43528973058483800 ) ) ;
#10941=DIRECTION ( 'NONE',  ( -0.000000000000000000, -0.000000000000000000, -1.000000000000000000 ) ) ;
#10942=CARTESIAN_POINT ( 'NONE',  ( 15.39755691330850951, 26.84919286949167017, -4.999999999999998224 ) ) ;
#10944=CARTESIAN_POINT ( 'NONE',  ( -17.81784622497958281, -13.85677843414106292, -30.00000000000001421 ) ) ;
#10946=AXIS2_PLACEMENT_3D ( 'NONE', #37134, #15198, #27588 ) ;
#10947=CARTESIAN_POINT ( 'NONE',  ( -20.57193854740110339, -18.21112165086101342, -17.70184765716385300 ) ) ;
#10948=CARTESIAN_POINT ( 'NONE',  ( 2.809657567551183455, -20.57247227728830907, -26.60406814968515832 ) ) ;
#10949=CARTESIAN_POINT ( 'NONE',  ( 15.28216090130213267, 25.92595189827088475, -8.300399430041283111 ) ) ;
#10950=CARTESIAN_POINT ( 'NONE',  ( 16.70239018954916332, 11.94149278131882497, -28.85809821401793229 ) ) ;
#10952=ORIENTED_EDGE ( 'NONE', *, *, #11589, .F. ) ;
#10953=CARTESIAN_POINT ( 'NONE',  ( -6.284372354627114632, 36.40390034292152421, -7.999116229162498648 ) ) ;
#10960=CARTESIAN_POINT ( 'NONE',  ( -30.32825103788703203, 0.1531031937912943341, -7.828961834450372415 ) ) ;
#10962=CARTESIAN_POINT ( 'NONE',  ( 27.17184055267051335, -8.181037515565595442, -16.75553878453715839 ) ) ;
#10963=AXIS2_PLACEMENT_3D ( 'NONE', #11512, #20663, #17214 ) ;
#10965=EDGE_LOOP ( 'NONE', ( #28268, #19947, #12841, #37426, #9180, #23783, #7117, #27890 ) ) ;
#10977=CARTESIAN_POINT ( 'NONE',  ( 15.67651070409536018, 15.51254429634443888, -21.03034014038798460 ) ) ;
#10978=CARTESIAN_POINT ( 'NONE',  ( 6.469800813340902401, 20.02804225434012508, -26.45432154560951332 ) ) ;
#10980=CARTESIAN_POINT ( 'NONE',  ( -19.48557158514985588, -11.25000000000002309, 0.000000000000000000 ) ) ;
#10981=CYLINDRICAL_SURFACE ( 'NONE', #30508, 18.00000000000002842 ) ;
#10983=CARTESIAN_POINT ( 'NONE',  ( 10.28494437836259401, -18.68278944082468840, -24.97709700113341214 ) ) ;
#10984=CARTESIAN_POINT ( 'NONE',  ( 35.36940577612500647, -20.42053594592276866, -5.000000000000000000 ) ) ;
#10987=ORIENTED_EDGE ( 'NONE', *, *, #6611, .T. ) ;
#10988=CARTESIAN_POINT ( 'NONE',  ( -14.02656482509936353, 23.94253483213065437, -13.51260121954110183 ) ) ;
#10991=CARTESIAN_POINT ( 'NONE',  ( 9.221110303372956452, -18.35701242422515378, -28.71846602907799451 ) ) ;
#10998=CARTESIAN_POINT ( 'NONE',  ( -12.01180344372764530, 30.47904674458951035, -10.37449900079057485 ) ) ;
#11001=CARTESIAN_POINT ( 'NONE',  ( -34.80117605982864148, -8.634413430420472935, -7.612578086861918614 ) ) ;
#11004=CARTESIAN_POINT ( 'NONE',  ( 22.70770152948616882, 0.6873525397408100091, -21.62692844155446181 ) ) ;
#11009=CARTESIAN_POINT ( 'NONE',  ( -30.80677756886225183, -0.04596665832818841446, -6.416728566985741011 ) ) ;
#11012=CARTESIAN_POINT ( 'NONE',  ( 26.90501378883225314, -1.666325082333041552, -16.21919210836066227 ) ) ;
#11017=EDGE_CURVE ( 'NONE', #30187, #32040, #3699, .T. ) ;
#11022=B_SPLINE_CURVE_WITH_KNOTS ( 'NONE', 3,
 ( #19763, #10214, #32159, #7158, #4319, #10623, #1482, #32772, #1893, #7770 ),
 .UNSPECIFIED., .F., .F.,
 ( 4, 2, 2, 2, 4 ),
 ( 0.1234515740337736034, 0.2679468505892486085, 0.4124421271447235582, 0.5569374037001986188, 0.7014326802556738460 ),
 .UNSPECIFIED. ) ;
#11027=CARTESIAN_POINT ( 'NONE',  ( 6.092423932518094887, 37.33975570695338320, -4.999999999999998224 ) ) ;
#11030=CARTESIAN_POINT ( 'NONE',  ( 19.66234726371370201, -27.08195440243529006, -6.812183372440195228 ) ) ;
#11036=CARTESIAN_POINT ( 'NONE',  ( 10.96848842646544853, 17.47186599299789123, -28.07314336957281142 ) ) ;
#11038=CARTESIAN_POINT ( 'NONE',  ( -15.58277398399269131, 26.10415450534656046, -5.946235503377694798 ) ) ;
#11041=CARTESIAN_POINT ( 'NONE',  ( 11.73655712706644572, 18.86307847280393091, -22.74338934216403629 ) ) ;
#11042=EDGE_CURVE ( 'NONE', #31785, #33916, #5419, .T. ) ;
#11044=CARTESIAN_POINT ( 'NONE',  ( 23.11556285573274394, -13.67656654032385966, -18.60984667135146253 ) ) ;
#11046=CARTESIAN_POINT ( 'NONE',  ( -11.80048683308201518, 20.30964621748999122, -20.47546970256553678 ) ) ;
#11048=CARTESIAN_POINT ( 'NONE',  ( -13.64307358185168439, -21.94662204693058172, -17.28659994694505997 ) ) ;
#11051=CARTESIAN_POINT ( 'NONE',  ( -30.37997259716803100, -13.60122796121996203, -12.90426562829724055 ) ) ;
#11052=CARTESIAN_POINT ( 'NONE',  ( -14.59935253407961930, -26.03713580996503296, -8.772365449628392042 ) ) ;
#11054=CARTESIAN_POINT ( 'NONE',  ( 16.58472503010262145, 19.97504727872816943, -11.75017852518634776 ) ) ;
#11056=CARTESIAN_POINT ( 'NONE',  ( 20.18678365231757255, 3.805571786065587769, -28.79240286594302489 ) ) ;
#11061=CARTESIAN_POINT ( 'NONE',  ( -24.01208527996724840, 0.3188823248074318939, -19.47337513750245819 ) ) ;
#11062=CARTESIAN_POINT ( 'NONE',  ( 20.63344826760219775, 0.3739914392306604163, -28.05361808214927066 ) ) ;
#11065=ORIENTED_EDGE ( 'NONE', *, *, #27652, .T. ) ;
#11066=CARTESIAN_POINT ( 'NONE',  ( -28.96942539544459549, 1.744189647663177523, -7.367551979210757551 ) ) ;
#11068=CARTESIAN_POINT ( 'NONE',  ( -30.41237130417910706, 3.314011747244096195, -5.000000000000000000 ) ) ;
#11076=CARTESIAN_POINT ( 'NONE',  ( -25.54365046647732029, 5.272554438015793821, -9.817126893295599288 ) ) ;
#11079=CARTESIAN_POINT ( 'NONE',  ( 26.88891980231563394, -23.41974722532487974, -9.768121312577717319 ) ) ;
#11084=CARTESIAN_POINT ( 'NONE',  ( 14.57748215141210757, 25.86296597815312737, -10.62311630137386587 ) ) ;
#11086=CARTESIAN_POINT ( 'NONE',  ( -13.90277657046047288, 15.06583648262319031, -30.00000000000000711 ) ) ;
#11088=CARTESIAN_POINT ( 'NONE',  ( 13.95448054433643392, -24.59828557378244085, -12.55371339440786116 ) ) ;
#11090=CARTESIAN_POINT ( 'NONE',  ( 13.49780444981478844, 22.80326206385345245, -15.45136375860262845 ) ) ;
#11094=CARTESIAN_POINT ( 'NONE',  ( -15.20842241300166009, 26.48812948757255015, -7.825058628721806464 ) ) ;
#11096=CARTESIAN_POINT ( 'NONE',  ( -15.40614666684921552, -26.59809411392278733, -6.887480037654896137 ) ) ;
#11098=CARTESIAN_POINT ( 'NONE',  ( -16.89362134160771944, -11.62925611732713804, -30.00000000000001421 ) ) ;
#11099=CARTESIAN_POINT ( 'NONE',  ( -5.350130231482848941, -21.35397508028911773, -21.04018493678614377 ) ) ;
#11100=CARTESIAN_POINT ( 'NONE',  ( 14.54495187225327868, 22.76206543785304248, -13.57072665076263185 ) ) ;
#11102=CARTESIAN_POINT ( 'NONE',  ( 23.31974132639167863, 9.208228383191446653, -6.934278112824287632 ) ) ;
#11105=CARTESIAN_POINT ( 'NONE',  ( 3.863783140547853712E-14, -86.77689918168233874, 3.000000000000000000 ) ) ;
#11108=CARTESIAN_POINT ( 'NONE',  ( -21.08730904962191133, -1.198901753354387534, -26.04825129587869270 ) ) ;
#11113=CARTESIAN_POINT ( 'NONE',  ( 33.88951946378950453, -17.36670660975930147, -7.118497633377743661 ) ) ;
#11121=CARTESIAN_POINT ( 'NONE',  ( 1.552613142282920355, 37.67816372275503767, -7.972283367467844606 ) ) ;
#11128=CARTESIAN_POINT ( 'NONE',  ( 11.14360014059721848, 20.13980330270795349, -21.48012828381845196 ) ) ;
#11131=CARTESIAN_POINT ( 'NONE',  ( -18.12326418384769866, 12.88339258814709964, -19.04514329360673486 ) ) ;
#11136=CARTESIAN_POINT ( 'NONE',  ( 9.550008964001319711, -18.19057619834521233, -28.70580708904410372 ) ) ;
#11138=CARTESIAN_POINT ( 'NONE',  ( 14.82211149595034350, 25.66540809471278806, -10.17682616307655330 ) ) ;
#11142=CARTESIAN_POINT ( 'NONE',  ( -27.75902213711245636, -24.56286694941507420, -7.146441665128197229 ) ) ;
#11143=CARTESIAN_POINT ( 'NONE',  ( 3.937535457903849068, -24.55738665131292819, -8.888856001756707315 ) ) ;
#11144=CARTESIAN_POINT ( 'NONE',  ( 13.92524374386434971, 23.06449320611515574, -14.49605255741758114 ) ) ;
#11145=CARTESIAN_POINT ( 'NONE',  ( 17.26157349013544007, 11.42543953884226759, -26.61627152139759289 ) ) ;
#11147=CARTESIAN_POINT ( 'NONE',  ( -6.310829074464455068, 36.59364124554614506, -7.568975181432845645 ) ) ;
#11149=AXIS2_PLACEMENT_3D ( 'NONE', #38749, #10718, #32667 ) ;
#11155=CARTESIAN_POINT ( 'NONE',  ( -21.67682104884834970, 0.8966140999393611422, -23.87369810390991631 ) ) ;
#11158=CARTESIAN_POINT ( 'NONE',  ( 20.35255112268399458, -5.483977284129752050, -26.39574775961089514 ) ) ;
#11159=ADVANCED_FACE ( 'NONE', ( #26939 ), #1968, .T. ) ;
#11174=CARTESIAN_POINT ( 'NONE',  ( 15.82467753361613205, 14.38668779758848082, -23.23502576981553602 ) ) ;
#11175=CARTESIAN_POINT ( 'NONE',  ( 8.609117341516606459, 22.13848295504110197, -21.12116105944807032 ) ) ;
#11177=DIRECTION ( 'NONE',  ( 1.000000000000000000, 0.000000000000000000, 0.000000000000000000 ) ) ;
#11181=CARTESIAN_POINT ( 'NONE',  ( 13.82053027212990592, -23.66662816038719441, -14.43394760191610615 ) ) ;
#11182=CARTESIAN_POINT ( 'NONE',  ( 14.98890121934609532, -28.67928442654221044, -5.000000000000000000 ) ) ;
#11184=CARTESIAN_POINT ( 'NONE',  ( -15.29018876279933536, 26.53061139393243550, -7.357746246747966623 ) ) ;
#11186=CARTESIAN_POINT ( 'NONE',  ( 9.552484026374298054, -19.39438616658035031, -23.93357300817531552 ) ) ;
#11192=CARTESIAN_POINT ( 'NONE',  ( -11.39446229461578852, 31.55080954265326199, -9.887314613259318818 ) ) ;
#11196=CARTESIAN_POINT ( 'NONE',  ( -34.33172124301603390, -5.488825450266375583, -6.338420623816570121 ) ) ;
#11199=CARTESIAN_POINT ( 'NONE',  ( 21.69624659619600138, 0.7958053819504173898, -23.86200436752996623 ) ) ;
#11204=CARTESIAN_POINT ( 'NONE',  ( -29.57198801820384659, 0.07677956331076821184, -10.18105163486785436 ) ) ;
#11208=CARTESIAN_POINT ( 'NONE',  ( 33.62952761534187118, -5.089175442527881899, -8.119193510173552397 ) ) ;
#11214=CARTESIAN_POINT ( 'NONE',  ( 15.41558956984165363, 26.78481017248027740, -5.000000000000000000 ) ) ;
#11222=CARTESIAN_POINT ( 'NONE',  ( 2.056640691923211417, 20.39672081104026802, -30.00000000000001066 ) ) ;
#11225=CARTESIAN_POINT ( 'NONE',  ( 14.71739798221114626, -19.47888500857317240, -20.11316221547454219 ) ) ;
#11231=CARTESIAN_POINT ( 'NONE',  ( 11.09749326504985056, 17.81885627187519816, -26.21546615232898958 ) ) ;
#11233=CARTESIAN_POINT ( 'NONE',  ( -15.21277803108789328, 25.35827226598801687, -9.246070508268418919 ) ) ;
#11237=CARTESIAN_POINT ( 'NONE',  ( 14.96898239447578760, 25.69415526101390057, -9.710597112631324634 ) ) ;
#11239=CARTESIAN_POINT ( 'NONE',  ( 17.86600798541212143, -10.56832063488048945, -27.70419187582904641 ) ) ;
#11241=CARTESIAN_POINT ( 'NONE',  ( -10.58469681223512637, 17.55611623359288131, -29.33974004713073214 ) ) ;
#11243=CARTESIAN_POINT ( 'NONE',  ( -10.63103180431346395, -17.81178731582381403, -27.37356996827503863 ) ) ;
#11247=CARTESIAN_POINT ( 'NONE',  ( -28.92757974739110693, -10.91245307248345853, -14.78116652952236443 ) ) ;
#11248=CARTESIAN_POINT ( 'NONE',  ( -14.83165383358532452, -26.38547499157037990, -7.359629187061518252 ) ) ;
#11251=CARTESIAN_POINT ( 'NONE',  ( 27.31176527514317343, 2.051244179470905760, -11.67027739895878646 ) ) ;
#11256=CARTESIAN_POINT ( 'NONE',  ( -30.71039170661696716, -0.1163676949505514646, -7.354338998695498120 ) ) ;
#11257=CARTESIAN_POINT ( 'NONE',  ( 31.58308575085905190, -0.9855460381432907813, -6.862365370586210211 ) ) ;
#11262=CARTESIAN_POINT ( 'NONE',  ( -29.11873305926894417, 1.737964268060802953, -6.420677056849690700 ) ) ;
#11263=CARTESIAN_POINT ( 'NONE',  ( 17.34253826539385201, 27.32041144647958575, -5.000000000000000000 ) ) ;
#11266=CLOSED_SHELL ( 'NONE', ( #32511, #27404, #33361, #39597, #3196, #28429, #286, #2573, #10245, #13818, #39785, #24293, #12740, #20490, #13362, #36345, #14309, #24138, #10824, #30987, #24396, #33386, #22885, #9298, #36994, #37308, #10367, #35893, #23208, #9613, #25246, #16383, #16718, #17622, #32763, #37083, #1609, #6655, #38946, #319, #3655, #15061, #10395, #3957, #11159, #13101, #13671, #26772, #3360 ) ) ;
#11276=CARTESIAN_POINT ( 'NONE',  ( -20.12887129416308696, 5.733943412042154186, -25.39721956534479119 ) ) ;
#11279=CARTESIAN_POINT ( 'NONE',  ( 15.24725239375168329, -14.05410354436919285, -27.77140347803001319 ) ) ;
#11283=CARTESIAN_POINT ( 'NONE',  ( 14.98650480333069979, 26.50796964270606537, -8.751387093918793880 ) ) ;
#11287=CARTESIAN_POINT ( 'NONE',  ( -14.96418064126415715, 20.04621382461933976, -15.64591645429735678 ) ) ;
#11293=CARTESIAN_POINT ( 'NONE',  ( 11.49255140715953338, 18.43021842612911598, -23.85520735916814772 ) ) ;
#11297=CARTESIAN_POINT ( 'NONE',  ( -14.97507841241774784, 26.10841250006580339, -9.231366820537651563 ) ) ;
#11299=CARTESIAN_POINT ( 'NONE',  ( -14.99851249572590106, -25.99467288956163813, -9.237413589426980209 ) ) ;
#11301=CARTESIAN_POINT ( 'NONE',  ( -33.71484418225002599, -17.65950029506896612, -7.118567158664396821 ) ) ;
#11303=CARTESIAN_POINT ( 'NONE',  ( -6.123308122133267695, -19.62006737319780569, -29.40205820084093702 ) ) ;
#11304=CARTESIAN_POINT ( 'NONE',  ( 14.78937771930062262, 23.24318486792957117, -12.59837077348300660 ) ) ;
#11305=ORIENTED_EDGE ( 'NONE', *, *, #16868, .T. ) ;
#11306=CARTESIAN_POINT ( 'NONE',  ( 24.38209929399536335, 7.347059586047067548, -8.383116823341570267 ) ) ;
#11311=CARTESIAN_POINT ( 'NONE',  ( -32.95954470968036532, -2.553576478305152886, -5.000000000000000000 ) ) ;
#11312=CARTESIAN_POINT ( 'NONE',  ( 28.35484778630695502, 0.1198746217886747789, -12.54935875910663157 ) ) ;
#11325=CARTESIAN_POINT ( 'NONE',  ( 0.8578242162873520593, 21.13533821733210871, -26.25769815819063524 ) ) ;
#11326=CARTESIAN_POINT ( 'NONE',  ( -18.00000000000003197, 22.50000000000001066, 3.000000000000000000 ) ) ;
#11332=CARTESIAN_POINT ( 'NONE',  ( 14.30190381450494286, 27.90070721307182566, -9.148110432232169131 ) ) ;
#11335=CARTESIAN_POINT ( 'NONE',  ( -18.85571089263951450, 16.25964530329961022, -9.864473642832360056 ) ) ;
#11338=CARTESIAN_POINT ( 'NONE',  ( 15.10121951614408253, -26.15095910722338601, -8.766956026588630380 ) ) ;
#11341=CARTESIAN_POINT ( 'NONE',  ( 15.00671440964051939, 26.00632701074570008, -9.236423267190737363 ) ) ;
#11342=CARTESIAN_POINT ( 'NONE',  ( 12.05832241004688399, 18.99596958976722760, -30.00000000000000000 ) ) ;
#11346=CARTESIAN_POINT ( 'NONE',  ( -24.87365189169005575, -23.40965842456435908, -11.14002769881621724 ) ) ;
#11347=CARTESIAN_POINT ( 'NONE',  ( 2.790632566740769871, -20.50748363971857913, -27.16196803510360169 ) ) ;
#11348=CARTESIAN_POINT ( 'NONE',  ( 14.67493102267895466, 24.58460314029640159, -11.61047959535504148 ) ) ;
#11349=CARTESIAN_POINT ( 'NONE',  ( 19.59303125460614226, 10.94001574543910138, -18.02074012208363385 ) ) ;
#11352=CARTESIAN_POINT ( 'NONE',  ( -4.809622099922509442, 20.53902726650351340, -26.36567314579518850 ) ) ;
#11359=CARTESIAN_POINT ( 'NONE',  ( -23.26829119944321178, 0.6879608890881370176, -20.55845448473494486 ) ) ;
#11362=CARTESIAN_POINT ( 'NONE',  ( 31.86584383545969246, -10.62267807593470259, -12.03292509902580854 ) ) ;
#11368=DIRECTION ( 'NONE',  ( 0.000000000000000000, 0.000000000000000000, 1.000000000000000000 ) ) ;
#11378=CARTESIAN_POINT ( 'NONE',  ( 18.58187274253394605, 17.94739436884781369, -5.960075704151572396 ) ) ;
#11379=CARTESIAN_POINT ( 'NONE',  ( 7.608710298680324335, 19.37355573834689437, -27.20130433680634141 ) ) ;
#11383=CARTESIAN_POINT ( 'NONE',  ( 12.48110824329010171, -22.01890908291360205, -17.41505214487477105 ) ) ;
#11384=DIRECTION ( 'NONE',  ( 0.000000000000000000, 0.000000000000000000, 1.000000000000000000 ) ) ;
#11389=CARTESIAN_POINT ( 'NONE',  ( -14.53044073688932869, 24.97606202870426628, -11.59869272441059174 ) ) ;
#11391=CARTESIAN_POINT ( 'NONE',  ( 9.824869631482991750, -19.77893024222395368, -22.81952676811747693 ) ) ;
#11395=CARTESIAN_POINT ( 'NONE',  ( -11.90375846996125020, 33.19065507634929446, -5.000000000000001776 ) ) ;
#11402=CARTESIAN_POINT ( 'NONE',  ( 20.81180504415543808, 0.8748342307719589872, -26.83400273307002237 ) ) ;
#11407=CARTESIAN_POINT ( 'NONE',  ( -27.72708288707136148, 0.2041362863144290662, -13.51430501883785595 ) ) ;
#11411=CARTESIAN_POINT ( 'NONE',  ( 20.84830255071761584, -2.293361874497828357, -26.59171325517713669 ) ) ;
#11413=EDGE_CURVE ( 'NONE', #33916, #37897, #15941, .T. ) ;
#11417=CARTESIAN_POINT ( 'NONE',  ( -26.35691893567060617, -28.22903657647675857, -5.000000000000004441 ) ) ;
#11425=CARTESIAN_POINT ( 'NONE',  ( 4.004005824709742534, 20.71913140499757588, -26.33338948413068792 ) ) ;
#11426=CARTESIAN_POINT ( 'NONE',  ( 32.33143948541783885, 1.358872982501748927, -5.000000000000000000 ) ) ;
#11429=CARTESIAN_POINT ( 'NONE',  ( 12.74496003955331602, -18.08351565856460041, -23.53601421872712862 ) ) ;
#11434=CARTESIAN_POINT ( 'NONE',  ( 12.32426020000443678, 20.57966432427881287, -19.48222999790586130 ) ) ;
#11436=CARTESIAN_POINT ( 'NONE',  ( -13.56937750933248843, 21.60099091529283655, -16.49869329321488465 ) ) ;
#11439=CARTESIAN_POINT ( 'NONE',  ( 11.95881310940501052, 19.31147990981001428, -21.62860280665383428 ) ) ;
#11441=CARTESIAN_POINT ( 'NONE',  ( 18.61388091722034943, -11.78005302609667737, -24.22059683775887606 ) ) ;
#11443=CARTESIAN_POINT ( 'NONE',  ( -14.70800301661877363, 26.47766101481222378, -9.672390817437571897 ) ) ;
#11445=CARTESIAN_POINT ( 'NONE',  ( -11.32445066732773142, -18.74575232930073554, -23.71343054792953708 ) ) ;
#11448=CARTESIAN_POINT ( 'NONE',  ( -26.01876133091875687, -8.953118292131030387, -17.69243264847248653 ) ) ;
#11449=CARTESIAN_POINT ( 'NONE',  ( -11.44614701672549728, -21.52147791799877652, -18.49673592605288874 ) ) ;
#11452=CARTESIAN_POINT ( 'NONE',  ( 28.22673339625941935, 2.021307961998640490, -9.272653165744820569 ) ) ;
#11457=CARTESIAN_POINT ( 'NONE',  ( -25.24992131713657884, 0.3092178984780983853, -17.42948113351768669 ) ) ;
#11458=CARTESIAN_POINT ( 'NONE',  ( 32.12080372859628596, -1.419867088699604984, -5.000000000000000888 ) ) ;
#11463=CARTESIAN_POINT ( 'NONE',  ( -21.41754555983938602, 3.564190076994790068, -23.03422754373932335 ) ) ;
#11473=CARTESIAN_POINT ( 'NONE',  ( -25.65838226093921648, 5.279357062076430296, -9.330829415115919900 ) ) ;
#11476=CARTESIAN_POINT ( 'NONE',  ( 23.26876723194845908, -24.22783250195383076, -11.17799550874850567 ) ) ;
#11479=CARTESIAN_POINT ( 'NONE',  ( 12.43688989749638907, 21.37114209746378179, -18.40534107864847968 ) ) ;
#11483=CARTESIAN_POINT ( 'NONE',  ( -13.41783481295519564, 15.62964107709064976, -28.19920321125439244 ) ) ;
#11488=CARTESIAN_POINT ( 'NONE',  ( 11.50098969431590668, 18.42294700796338702, -23.85649179623154481 ) ) ;
#11490=CARTESIAN_POINT ( 'NONE',  ( 12.93090914344497122, 21.64873284080849203, -17.43820100889084657 ) ) ;
#11492=CARTESIAN_POINT ( 'NONE',  ( -11.22930476693127311, 18.10080634600636529, -25.00346310164814767 ) ) ;
#11494=CARTESIAN_POINT ( 'NONE',  ( -9.533178660976551200, -18.19926881236112592, -28.70647124653801896 ) ) ;
#11496=CARTESIAN_POINT ( 'NONE',  ( -32.33767308879468771, -16.92829965255246449, -9.727596525381697390 ) ) ;
#11497=CARTESIAN_POINT ( 'NONE',  ( -9.023319067658404080, -24.92662452266139184, -9.321921292790742442 ) ) ;
#11499=CARTESIAN_POINT ( 'NONE',  ( 12.21661684832558237, 18.39671740363510466, -22.81900652314237732 ) ) ;
#11502=CARTESIAN_POINT ( 'NONE',  ( 20.02700736633234868, 6.692680301631161122, -24.33429107806700742 ) ) ;
#11508=CARTESIAN_POINT ( 'NONE',  ( -20.50243331965346627, -0.1390943044478715751, -29.32999314426240289 ) ) ;
#11509=CARTESIAN_POINT ( 'NONE',  ( 20.48330953517068664, 0.8273339926270942835, -29.34778729633271510 ) ) ;
#11512=CARTESIAN_POINT ( 'NONE',  ( 3.863783140547853712E-14, -86.77689918168233874, -0.000000000000000000 ) ) ;
#11523=CARTESIAN_POINT ( 'NONE',  ( 1.575354112968664566, 38.41398891768359647, -5.855932988374854098 ) ) ;
#11524=LINE ( 'NONE', #11326, #8108 ) ;
#11530=CARTESIAN_POINT ( 'NONE',  ( 14.52179210396188758, 28.39636537094187574, -7.765798819039245515 ) ) ;
#11533=CARTESIAN_POINT ( 'NONE',  ( -16.43970055640401640, 12.42160327418225663, -27.72196673367218622 ) ) ;
#11536=CARTESIAN_POINT ( 'NONE',  ( 10.85850211433846013, -19.98559300887557555, -21.61446395924937036 ) ) ;
#11537=CARTESIAN_POINT ( 'NONE',  ( 15.41558956916362000, 26.78481017491965233, -5.000000000000000000 ) ) ;
#11538=CARTESIAN_POINT ( 'NONE',  ( 12.38021073363059799, 20.50496940924477229, -19.49405221216574091 ) ) ;
#11544=CARTESIAN_POINT ( 'NONE',  ( -27.52659592799652444, -22.96876690456295123, -9.758689385506642111 ) ) ;
#11545=CARTESIAN_POINT ( 'NONE',  ( 4.025418116673052715, -24.86707171575129038, -5.000000000000002665 ) ) ;
#11546=CARTESIAN_POINT ( 'NONE',  ( 14.65085127499396478, 24.64916743084969042, -11.60854621773958684 ) ) ;
#11547=CARTESIAN_POINT ( 'NONE',  ( 20.78558868895880707, 12.80151593431163093, -9.395610594804281845 ) ) ;
#11550=CARTESIAN_POINT ( 'NONE',  ( -4.067729689095753720, 20.10162097886301780, -29.99999999999998934 ) ) ;
#11552=ORIENTED_EDGE ( 'NONE', *, *, #33839, .F. ) ;
#11559=CARTESIAN_POINT ( 'NONE',  ( -30.40797137996420929, 0.1992154573447958432, -7.358886591698631463 ) ) ;
#11560=CARTESIAN_POINT ( 'NONE',  ( 20.01479607499403812, -5.392035505496489023, -27.79632597738025623 ) ) ;
#11575=CARTESIAN_POINT ( 'NONE',  ( 16.14253851327366363, 13.55324706950144886, -24.35198715851059248 ) ) ;
#11577=CARTESIAN_POINT ( 'NONE',  ( 10.13695427535512117, 26.23223918441782843, -16.00337151103656552 ) ) ;
#11579=CARTESIAN_POINT ( 'NONE',  ( -21.66453300257672154, 11.69411660682930787, -7.917832817197552053 ) ) ;
#11582=CARTESIAN_POINT ( 'NONE',  ( 15.98679081489500575, -26.83810770539577106, -5.940741301600179547 ) ) ;
#11586=CARTESIAN_POINT ( 'NONE',  ( -11.11125591800278478, 17.62252618941018056, -26.82911783566601116 ) ) ;
#11587=CARTESIAN_POINT ( 'NONE',  ( -15.42415429988070841, -17.33959852952462910, -22.15376138321191490 ) ) ;
#11588=CARTESIAN_POINT ( 'NONE',  ( 14.27123303369756790, -26.41390335293325009, -5.946466403055868710 ) ) ;
#11589=EDGE_CURVE ( 'NONE', #13116, #6755, #31779, .T. ) ;
#11595=CARTESIAN_POINT ( 'NONE',  ( -10.66039439689632395, 26.89947780815539247, -15.04199405158239600 ) ) ;
#11603=CARTESIAN_POINT ( 'NONE',  ( 29.72646830413813390, 0.1273344848627241122, -9.710811668020681964 ) ) ;
#11608=CARTESIAN_POINT ( 'NONE',  ( -30.87691200222618804, -0.01437998035276856316, -5.474195421119384619 ) ) ;
#11611=CARTESIAN_POINT ( 'NONE',  ( 32.29142382855410176, -3.921780356570798709, -9.954602144452415757 ) ) ;
#11613=VERTEX_POINT ( 'NONE', #38882 ) ;
#11625=CARTESIAN_POINT ( 'NONE',  ( 4.474472994054608854, 23.12859998392846705, -21.95241731158036202 ) ) ;
#11629=CARTESIAN_POINT ( 'NONE',  ( 13.15139800428180727, -18.60661763037684224, -22.40227382322720118 ) ) ;
#11636=CARTESIAN_POINT ( 'NONE',  ( 13.72215835960534314, 23.50258046650561283, -14.46509339062811250 ) ) ;
#11638=CARTESIAN_POINT ( 'NONE',  ( -15.42052737914556637, 25.77605439453884273, -7.831307328786774491 ) ) ;
#11642=CARTESIAN_POINT ( 'NONE',  ( 15.34434150811012465, 26.34414864991459737, -7.358482492565846300 ) ) ;
#11644=CARTESIAN_POINT ( 'NONE',  ( 32.27861313376966734, -19.10088880322608418, -8.403838041204926057 ) ) ;
#11646=CARTESIAN_POINT ( 'NONE',  ( -12.92543041999867803, 22.74201982050020376, -16.38141219968167306 ) ) ;
#11648=CARTESIAN_POINT ( 'NONE',  ( -16.98077657287944220, -25.38500131946631200, -11.42923376808981928 ) ) ;
#11652=CARTESIAN_POINT ( 'NONE',  ( -26.89345970280778175, -10.16057822180111536, -16.68776630141959316 ) ) ;
#11653=CARTESIAN_POINT ( 'NONE',  ( -15.26455680675359972, -26.65982646153380031, -5.946113180645928864 ) ) ;
#11656=CARTESIAN_POINT ( 'NONE',  ( 21.79450343673522639, 2.315575432259290523, -22.92150830105099146 ) ) ;
#11660=CARTESIAN_POINT ( 'NONE',  ( -21.28869832545893814, 0.6870496981110076895, -25.00484597054681757 ) ) ;
#11662=CARTESIAN_POINT ( 'NONE',  ( 32.00254677347309951, -1.406971461693646397, -6.390648070956889804 ) ) ;
#11666=CARTESIAN_POINT ( 'NONE',  ( -27.39893270769881184, 2.645307716681419397, -10.24383054656171765 ) ) ;
#11674=CARTESIAN_POINT ( 'NONE',  ( -22.74773350093838431, 5.112260648264027374, -17.82922536596295160 ) ) ;
#11677=CARTESIAN_POINT ( 'NONE',  ( 17.90862233137103132, -16.51690928828630689, -20.84349936702684047 ) ) ;
#11679=CARTESIAN_POINT ( 'NONE',  ( 11.43364758157541949, 19.15105928248557987, -22.69143459194921064 ) ) ;
#11683=CARTESIAN_POINT ( 'NONE',  ( -14.25469411907181261, 18.74119916489544124, -18.70450738159251713 ) ) ;
#11687=CARTESIAN_POINT ( 'NONE',  ( 15.41486640184582235, 26.69476953482462989, -5.946086842317699350 ) ) ;
#11692=CARTESIAN_POINT ( 'NONE',  ( -15.35726121420015211, 26.89840538448078888, -5.944526096835159201 ) ) ;
#11694=CARTESIAN_POINT ( 'NONE',  ( -14.77304657029772805, -25.65973629052345828, -10.17934284075853490 ) ) ;
#11696=CARTESIAN_POINT ( 'NONE',  ( -32.89633676153053443, -18.52163263618783162, -7.970821576684871346 ) ) ;
#11697=CARTESIAN_POINT ( 'NONE',  ( -12.68866578116655397, -24.42420696973755767, -12.60002993717948172 ) ) ;
#11699=CARTESIAN_POINT ( 'NONE',  ( 12.23345151996672264, 16.79682170085633430, -26.92720819876614158 ) ) ;
#11701=CARTESIAN_POINT ( 'NONE',  ( 24.72357752798934882, 6.416377239431996671, -9.837715644156144634 ) ) ;
#11706=CARTESIAN_POINT ( 'NONE',  ( -26.47597712984326890, -0.7517266478712665290, -16.31359411516780966 ) ) ;
#11707=CARTESIAN_POINT ( 'NONE',  ( 28.39060983474474753, 0.07700895002038117554, -12.54401228622873354 ) ) ;
#11720=CARTESIAN_POINT ( 'NONE',  ( 0.4051383682548583276, 37.70807721162720583, -7.971661926679036725 ) ) ;
#11724=LINE ( 'NONE', #40141, #34967 ) ;
#11728=CARTESIAN_POINT ( 'NONE',  ( 10.21381146793931549, 18.84016815455725080, -24.86718924084146565 ) ) ;
#11732=CARTESIAN_POINT ( 'NONE',  ( -19.14596416633794718, 16.58431542591694097, -6.930462030153276665 ) ) ;
#11736=CARTESIAN_POINT ( 'NONE',  ( 15.36829843292950848, -26.58855099483750806, -6.887934304372063110 ) ) ;
#11738=CARTESIAN_POINT ( 'NONE',  ( 15.35679505265130373, 26.72643039084889338, -6.416339992001557135 ) ) ;
#11740=CARTESIAN_POINT ( 'NONE',  ( 12.05832241004688399, 18.99596958976722760, -21.04195414767209726 ) ) ;
#11742=CARTESIAN_POINT ( 'NONE',  ( -16.64620719159282913, -13.00137674719640835, -26.29768302675261182 ) ) ;
#11743=CARTESIAN_POINT ( 'NONE',  ( 4.003204069988485436, -24.78938737036088824, -6.934010167115818746 ) ) ;
#11744=CARTESIAN_POINT ( 'NONE',  ( 12.64121829060639968, 20.16165939183971290, -19.53956656712336581 ) ) ;
#11745=CARTESIAN_POINT ( 'NONE',  ( 18.17819536212576281, 10.17765543567462494, -25.51248847685047849 ) ) ;
#11749=CARTESIAN_POINT ( 'NONE',  ( -4.163637899402453435, 37.39365738118117832, -7.553763481216830833 ) ) ;
#11755=CARTESIAN_POINT ( 'NONE',  ( -20.68510868473422804, 0.9644064859642085263, -27.45587699270683402 ) ) ;
#11756=CARTESIAN_POINT ( 'NONE',  ( 35.33511270614809519, -11.84873732983155925, -6.293930992841885619 ) ) ;
#11772=CARTESIAN_POINT ( 'NONE',  ( 26.24913643253236373, -20.23034912788282469, -12.91558456940952837 ) ) ;
#11773=CARTESIAN_POINT ( 'NONE',  ( 17.45454598098198673, 15.08987660865141933, -16.91469807549161075 ) ) ;
#11774=CARTESIAN_POINT ( 'NONE',  ( 7.745869706829908274, 19.75473637109295311, -25.89095885954563769 ) ) ;
#11776=CARTESIAN_POINT ( 'NONE',  ( -21.71367720907299770, 11.71909836743509636, -7.427745397021046969 ) ) ;
#11779=CARTESIAN_POINT ( 'NONE',  ( 14.99950937118286021, -25.70747749863527076, -10.16616245189924506 ) ) ;
#11782=CARTESIAN_POINT ( 'NONE',  ( -15.38932783545047478, 26.78602940361181339, -5.945706122906532443 ) ) ;
#11784=CARTESIAN_POINT ( 'NONE',  ( -24.93964139829124704, -26.28816300898122194, -5.879745673036421927 ) ) ;
#11785=CARTESIAN_POINT ( 'NONE',  ( 13.51079035047422749, -25.25079545357177935, -10.67726867737688323 ) ) ;
#11792=CARTESIAN_POINT ( 'NONE',  ( -12.54669116579298027, 32.01363879718496719, -7.228269468828303346 ) ) ;
#11797=CARTESIAN_POINT ( 'NONE',  ( 30.86596729670053563, -0.003225903683491798332, -5.474191125761192822 ) ) ;
#11799=VECTOR ( 'NONE', #39416, 1000.000000000000000 ) ;
#11802=CARTESIAN_POINT ( 'NONE',  ( -23.93377115618524442, 0.5022394957162249485, -19.49836098978260068 ) ) ;
#11805=CARTESIAN_POINT ( 'NONE',  ( 34.09142973781642638, -5.184893016320399006, -6.786029529690497775 ) ) ;
#11814=ORIENTED_EDGE ( 'NONE', *, *, #15504, .F. ) ;
#11817=CARTESIAN_POINT ( 'NONE',  ( 7.586125664261425428, 33.43449133166674869, -11.13268412101803939 ) ) ;
#11821=CARTESIAN_POINT ( 'NONE',  ( 18.83296736436365393, -24.71623834213119153, -12.24355243440530749 ) ) ;
#11822=SURFACE_SIDE_STYLE ('',( #37405 ) ) ;
#11824=CARTESIAN_POINT ( 'NONE',  ( -19.48557158514988785, -11.24999999999987743, 10.00000000000000000 ) ) ;
#11826=CARTESIAN_POINT ( 'NONE',  ( 15.30964094714013690, 26.71768783952137483, -6.885809892569045410 ) ) ;
#11828=CARTESIAN_POINT ( 'NONE',  ( -14.94032676572743767, 24.81194212842451563, -10.66625999421779269 ) ) ;
#11831=CARTESIAN_POINT ( 'NONE',  ( 12.96194030760161375, -23.08917773356923675, -15.45381493534388717 ) ) ;
#11833=CARTESIAN_POINT ( 'NONE',  ( 14.78413089825309434, 25.26060220695678993, -10.65622333237480923 ) ) ;
#11835=CARTESIAN_POINT ( 'NONE',  ( 31.39467639332050553, -19.90237361881552403, -8.844072599137296820 ) ) ;
#11837=CARTESIAN_POINT ( 'NONE',  ( -14.85775003842022102, 28.53279358564904555, -5.466018984421181948 ) ) ;
#11839=CARTESIAN_POINT ( 'NONE',  ( -17.29263770120802945, -27.09866115540251030, -5.466300565429026648 ) ) ;
#11843=CARTESIAN_POINT ( 'NONE',  ( -33.72599793200199514, -11.57189992363034570, -9.767970167873338383 ) ) ;
#11844=CARTESIAN_POINT ( 'NONE',  ( -15.28548941152575225, -26.69066991962944257, -5.474153390693990318 ) ) ;
#11848=CARTESIAN_POINT ( 'NONE',  ( 28.97648499451679527, 1.995013090243813236, -4.999999999999998224 ) ) ;
#11852=CARTESIAN_POINT ( 'NONE',  ( -28.41653591125160006, 0.04529035542138026837, -12.54075237691299094 ) ) ;
#11854=CARTESIAN_POINT ( 'NONE',  ( 31.92511577782137522, -1.398606727016608042, -6.852345169075132247 ) ) ;
#11858=CARTESIAN_POINT ( 'NONE',  ( -23.56736984768613041, 3.521302623928285858, -17.71584685096988565 ) ) ;
#11870=CARTESIAN_POINT ( 'NONE',  ( -22.91382620985103102, 6.848442421757915177, -14.83700933217039797 ) ) ;
#11873=CARTESIAN_POINT ( 'NONE',  ( 14.64330500336448004, -14.34584279044560162, -29.99999999999999289 ) ) ;
#11875=CARTESIAN_POINT ( 'NONE',  ( 10.80899027733819295, 17.41890095272876593, -29.34456996907283610 ) ) ;
#11878=CARTESIAN_POINT ( 'NONE',  ( -16.97879685541396455, 21.84934419274153683, -5.951441372114004480 ) ) ;
#11882=CARTESIAN_POINT ( 'NONE',  ( 15.38118955599525428, 26.63999108931288617, -6.417037871327162968 ) ) ;
#11886=CARTESIAN_POINT ( 'NONE',  ( -15.37369053509020667, 26.93276585663874556, -5.000000000000001776 ) ) ;
#11889=CARTESIAN_POINT ( 'NONE',  ( -14.12857205807981842, -24.62559611294807382, -12.54400053039158713 ) ) ;
#11893=CARTESIAN_POINT ( 'NONE',  ( -27.74053922457303401, -14.52380522957474795, -14.73393910564032616 ) ) ;
#11894=CARTESIAN_POINT ( 'NONE',  ( -10.35672055835056860, -23.76937265673268840, -13.66394602354463572 ) ) ;
#11896=CARTESIAN_POINT ( 'NONE',  ( 14.86260783703185417, 22.06351504111470874, -13.60475557901546750 ) ) ;
#11898=CARTESIAN_POINT ( 'NONE',  ( 22.11552067476606354, 6.995634713880600764, -16.89582745047114543 ) ) ;
#11903=CARTESIAN_POINT ( 'NONE',  ( -31.05298752102547155, -0.7743630725552020921, -8.259985541401292153 ) ) ;
#11905=CARTESIAN_POINT ( 'NONE',  ( 25.29308743037763918, 0.2312469298496797332, -17.41904786010038109 ) ) ;
#11918=CARTESIAN_POINT ( 'NONE',  ( 3.596573278996550993, 34.97522925885748180, -11.08051460049237491 ) ) ;
#11926=CARTESIAN_POINT ( 'NONE',  ( 14.69098151597639834, 28.78426858804810351, -5.926310556595937307 ) ) ;
#11929=CARTESIAN_POINT ( 'NONE',  ( -16.52500823362143834, 12.50774690784832543, -26.60145339744036264 ) ) ;
#11933=CARTESIAN_POINT ( 'NONE',  ( 9.631034963941338845, -18.33589862961692774, -27.44708460917885517 ) ) ;
#11934=CARTESIAN_POINT ( 'NONE',  ( -18.50896748101629541, -23.35909915790261948, -14.08898525485408904 ) ) ;
#11935=CARTESIAN_POINT ( 'NONE',  ( 12.39413036303996307, 20.48625930257312433, -19.49701620399656932 ) ) ;
#11936=CARTESIAN_POINT ( 'NONE',  ( 11.87498658133518248, 19.40059169592226240, -21.61373574364315076 ) ) ;
#11938=CARTESIAN_POINT ( 'NONE',  ( 11.31392148919589680, 36.91540483778863546, -14.26382729546508088 ) ) ;
#11941=CARTESIAN_POINT ( 'NONE',  ( -28.00154710540513392, -23.35202446123746256, -8.873473656866229575 ) ) ;
#11942=CARTESIAN_POINT ( 'NONE',  ( -0.2676006149246174526, -20.58428938002466779, -27.73625193941130007 ) ) ;
#11943=CARTESIAN_POINT ( 'NONE',  ( 15.58410715161808824, 26.18909738223269557, -5.000000000000000888 ) ) ;
#11944=CARTESIAN_POINT ( 'NONE',  ( 19.35653844823029246, 10.81242967103833763, -19.06682279225362819 ) ) ;
#11947=CARTESIAN_POINT ( 'NONE',  ( -2.848530395113701985, 20.31062432315956201, -29.22165717386838679 ) ) ;
#11949=CARTESIAN_POINT ( 'NONE',  ( -34.69811016863992137, -6.555196379703267517, -6.328619236691829464 ) ) ;
#11955=CARTESIAN_POINT ( 'NONE',  ( -29.42040707488883555, 0.4686144674514792219, -9.717579686123906768 ) ) ;
#11956=CARTESIAN_POINT ( 'NONE',  ( 26.94378894143373770, -9.905954980331337367, -16.69510737975683057 ) ) ;
#11970=CARTESIAN_POINT ( 'NONE',  ( 16.27615822911637622, -12.47890632334475747, -29.22043922964566676 ) ) ;
#11971=CARTESIAN_POINT ( 'NONE',  ( 17.93403218016955591, 14.29091524181443518, -16.94358179346269466 ) ) ;
#11972=CARTESIAN_POINT ( 'NONE',  ( 7.524521118624930338, 19.14141286767502947, -28.57295515480274517 ) ) ;
#11975=CARTESIAN_POINT ( 'NONE',  ( -18.67511144159872316, 8.486512637698147898, -29.42713777807604458 ) ) ;
#11977=CARTESIAN_POINT ( 'NONE',  ( 13.88701526290651422, -24.14100214001190281, -13.49798790650252833 ) ) ;
#11980=CARTESIAN_POINT ( 'NONE',  ( -11.04466200716893276, 17.52154582185139020, -27.44559064709055818 ) ) ;
#11981=CARTESIAN_POINT ( 'NONE',  ( -18.24003512488236467, -21.72694636099543075, -15.96283982311370941 ) ) ;
#11982=CARTESIAN_POINT ( 'NONE',  ( 13.09383889318130301, -26.15137312895040722, -5.947571630415806609 ) ) ;
#11985=ORIENTED_EDGE ( 'NONE', *, *, #21993, .T. ) ;
#11987=CARTESIAN_POINT ( 'NONE',  ( -9.942109246833966907, 33.34287839135563303, -9.382223997254289571 ) ) ;
#11993=CARTESIAN_POINT ( 'NONE',  ( 27.14326651887064656, 0.2312572436680407628, -14.47629528729547133 ) ) ;
#12000=CARTESIAN_POINT ( 'NONE',  ( -28.33198621730845446, 0.1486562545012954650, -12.55068749093940639 ) ) ;
#12002=ORIENTED_EDGE ( 'NONE', *, *, #34823, .F. ) ;
#12003=CARTESIAN_POINT ( 'NONE',  ( 26.67980387914269969, -3.134049882918540142, -17.05610665002131299 ) ) ;
#12004=CIRCLE ( 'NONE', #34704, 22.50000000000000355 ) ;
#12014=CARTESIAN_POINT ( 'NONE',  ( -15.41558956984166251, 26.78481017248024898, -5.000000000000000000 ) ) ;
#12017=CARTESIAN_POINT ( 'NONE',  ( 4.106875433146082166, 25.19931270338924989, -19.70517226477189965 ) ) ;
#12020=CARTESIAN_POINT ( 'NONE',  ( 10.69198779663409304, -17.56583795296588235, -28.65972484765404005 ) ) ;
#12027=CARTESIAN_POINT ( 'NONE',  ( -14.95102318841846412, 25.74959356765882390, -9.709746325769389230 ) ) ;
#12030=CARTESIAN_POINT ( 'NONE',  ( 9.727834406736230122, -18.58976127751570573, -26.23031535258787628 ) ) ;
#12034=CARTESIAN_POINT ( 'NONE',  ( -10.51657528416702370, 20.72986206170195800, -21.37251766699545996 ) ) ;
#12036=CARTESIAN_POINT ( 'NONE',  ( -18.32806035864107841, -25.83311609833614853, -10.45574956145189560 ) ) ;
#12038=DIRECTION ( 'NONE',  ( -1.000000000000000000, 0.000000000000000000, 0.000000000000000000 ) ) ;
#12040=CARTESIAN_POINT ( 'NONE',  ( -33.38534935071415788, -11.45126148588078330, -10.21694987028886636 ) ) ;
#12041=CARTESIAN_POINT ( 'NONE',  ( -12.38214629039859282, -22.55476777646130415, -16.46447605962150362 ) ) ;
#12044=CARTESIAN_POINT ( 'NONE',  ( 28.68541928171654831, 0.3475515138929626269, -11.60796932871038756 ) ) ;
#12048=CARTESIAN_POINT ( 'NONE',  ( -30.93630827890108037, -0.1109845943994294815, -5.945062553525370497 ) ) ;
#12050=CARTESIAN_POINT ( 'NONE',  ( 20.72896443152828283, 0.1975693286415366734, -27.40608702327256907 ) ) ;
#12053=CARTESIAN_POINT ( 'NONE',  ( -20.56177667423478894, 2.892092975756595408, -26.97112085952661431 ) ) ;
#12063=CARTESIAN_POINT ( 'NONE',  ( 37.48557158514985588, -11.25000000000009415, -5.000000000000000000 ) ) ;
#12064=ORIENTED_EDGE ( 'NONE', *, *, #3943, .T. ) ;
#12065=CARTESIAN_POINT ( 'NONE',  ( -20.93482781216526689, 6.580497575008867450, -21.07328139004194156 ) ) ;
#12068=B_SPLINE_CURVE_WITH_KNOTS ( 'NONE', 3,
 ( #37094, #27746, #31584, #15752, #25294, #34250 ),
 .UNSPECIFIED., .F., .F.,
 ( 4, 2, 4 ),
 ( 0.000000000000000000, 0.5000000000000000000, 1.000000000000000000 ),
 .UNSPECIFIED. ) ;
#12069=CARTESIAN_POINT ( 'NONE',  ( 15.08063968188699633, -13.89948965651085544, -29.99999999999999645 ) ) ;
#12071=CARTESIAN_POINT ( 'NONE',  ( 14.74369174452469089, 25.90307666149954713, -10.16263518668779398 ) ) ;
#12073=ORIENTED_EDGE ( 'NONE', *, *, #7911, .F. ) ;
#12074=CARTESIAN_POINT ( 'NONE',  ( -12.35093606704898228, 16.57560007382403455, -27.53901265143020183 ) ) ;
#12077=CARTESIAN_POINT ( 'NONE',  ( 13.50121191754509908, 22.79660094963672634, -15.45185408499526680 ) ) ;
#12082=CARTESIAN_POINT ( 'NONE',  ( -13.71542125295547088, 23.51752206020428915, -14.46353376464415774 ) ) ;
#12084=CARTESIAN_POINT ( 'NONE',  ( -10.63009531068781577, -19.54863766215186516, -22.72267709242899869 ) ) ;
#12088=CARTESIAN_POINT ( 'NONE',  ( -30.07688550757283608, -16.93187886526812136, -11.97280104394458711 ) ) ;
#12089=CARTESIAN_POINT ( 'NONE',  ( -10.49402848346364259, -21.11063220854802935, -19.60472159036592288 ) ) ;
#12091=CARTESIAN_POINT ( 'NONE',  ( 12.89744199737797992, 19.01286579302862734, -20.67027483038949498 ) ) ;
#12094=CARTESIAN_POINT ( 'NONE',  ( 21.14538636724398657, 6.850996120451639193, -20.02713119748161930 ) ) ;
#12101=CARTESIAN_POINT ( 'NONE',  ( -31.86521589244229702, -1.232139016781935492, -6.393609547768853929 ) ) ;
#12102=CARTESIAN_POINT ( 'NONE',  ( 23.96264080723695500, 0.4348472519531068614, -19.48932385422077118 ) ) ;
#12117=CARTESIAN_POINT ( 'NONE',  ( 2.078853377173544903, 28.96599879814208123, -16.63595397449693536 ) ) ;
#12124=CARTESIAN_POINT ( 'NONE',  ( 14.81731206233621023, 27.65607728349727523, -7.787956928312406824 ) ) ;
#12127=CARTESIAN_POINT ( 'NONE',  ( -17.62030008941222547, 17.79749385453288113, -11.80820510887239827 ) ) ;
#12130=CARTESIAN_POINT ( 'NONE',  ( 15.15893967609533455, -26.27887000457485200, -8.297842270817525900 ) ) ;
#12131=CARTESIAN_POINT ( 'NONE',  ( -12.63282099796252034, -16.15870876741617579, -29.28150700448700405 ) ) ;
#12132=CARTESIAN_POINT ( 'NONE',  ( 15.10138251737945936, 26.13808434145727944, -8.767643565617390777 ) ) ;
#12133=CARTESIAN_POINT ( 'NONE',  ( 10.99175044165756709, 17.35733570206949494, -28.70635921313413164 ) ) ;
#12139=CARTESIAN_POINT ( 'NONE',  ( -18.83962338116515056, -15.66599860280581602, -20.78005700281575230 ) ) ;
#12140=CARTESIAN_POINT ( 'NONE',  ( -0.3299534963231213758, -22.70197746772678826, -16.98173616913636508 ) ) ;
#12141=CARTESIAN_POINT ( 'NONE',  ( 13.76173484786665391, 22.29158688768309560, -15.48881288112352017 ) ) ;
#12143=CARTESIAN_POINT ( 'NONE',  ( 17.53305258709997716, 10.68547909316169608, -28.86305607330305634 ) ) ;
#12144=CARTESIAN_POINT ( 'NONE',  ( 2.485571585149743523, -11.24999999999995737, 6.000000000000000000 ) ) ;
#12145=CARTESIAN_POINT ( 'NONE',  ( -5.326384147119485490, 37.63231972733477448, -5.437470600199088899 ) ) ;
#12147=CARTESIAN_POINT ( 'NONE',  ( -20.17828169183510667, -3.673208557823401943, -30.00000000000000355 ) ) ;
#12154=CARTESIAN_POINT ( 'NONE',  ( -28.36600098059368236, 0.7354731085742703955, -11.62209496411426812 ) ) ;
#12155=CARTESIAN_POINT ( 'NONE',  ( 19.43389763942624882, -6.523976669268586548, -29.23235429811387576 ) ) ;
#12164=CARTESIAN_POINT ( 'NONE',  ( -2.944636116024315520, 26.57046322055783349, -18.64425712812955993 ) ) ;
#12165=FACE_OUTER_BOUND ( 'NONE', #36868, .T. ) ;
#12168=CARTESIAN_POINT ( 'NONE',  ( 18.29362116886485978, -14.93416125425190977, -21.91937720398613720 ) ) ;
#12169=CARTESIAN_POINT ( 'NONE',  ( 15.76482823105918385, 13.10325120709816105, -29.42076664285941590 ) ) ;
#12171=CARTESIAN_POINT ( 'NONE',  ( 11.09465891820651784, 26.43777197077398355, -15.08134290002067246 ) ) ;
#12174=CARTESIAN_POINT ( 'NONE',  ( -21.78527990638771072, 10.57721431994490935, -10.88166847450601438 ) ) ;
#12176=CARTESIAN_POINT ( 'NONE',  ( 14.93814303287626544, -25.69500553019197042, -10.16968976574983685 ) ) ;
#12179=CARTESIAN_POINT ( 'NONE',  ( -16.77267017469754151, -29.13948811618693924, -5.000000000000000000 ) ) ;
#12181=CARTESIAN_POINT ( 'NONE',  ( -15.35363586822866289, 26.73755632045413932, -6.416160081111284441 ) ) ;
#12182=CARTESIAN_POINT ( 'NONE',  ( -23.85290253531346849, -26.59866202527626555, -5.885430692555547516 ) ) ;
#12183=CARTESIAN_POINT ( 'NONE',  ( 10.51335036728116279, -22.08948547754980751, -17.58519077309815870 ) ) ;
#12187=CARTESIAN_POINT ( 'NONE',  ( -10.30584816049105257, 34.79301137796964127, -5.000000000000004441 ) ) ;
#12192=CARTESIAN_POINT ( 'NONE',  ( 30.34016821446444823, 0.008728377367246306986, -8.297816611031924694 ) ) ;
#12193=CARTESIAN_POINT ( 'NONE',  ( 12.26832665498864294, 32.91590888319125696, -4.999999999999999112 ) ) ;
#12194=DIRECTION ( 'NONE',  ( 0.000000000000000000, 0.000000000000000000, 1.000000000000000000 ) ) ;
#12197=CARTESIAN_POINT ( 'NONE',  ( -30.31183173745759873, 0.03880945276234878255, -8.298106778462893018 ) ) ;
#12200=CARTESIAN_POINT ( 'NONE',  ( 34.59626701887397360, -6.235679855831036456, -6.331402358434438327 ) ) ;
#12217=CARTESIAN_POINT ( 'NONE',  ( 7.105293529131195385, 36.67938314382616483, -6.292395027995508094 ) ) ;
#12221=CARTESIAN_POINT ( 'NONE',  ( 16.88068922968714247, -26.18916093630494757, -9.608643031638695930 ) ) ;
#12226=CARTESIAN_POINT ( 'NONE',  ( -11.02974916714818043, 17.33288907044355298, -28.70794164723638175 ) ) ;
#12229=CARTESIAN_POINT ( 'NONE',  ( 14.83593602140731882, -25.95848014736257880, -9.240082701127958487 ) ) ;
#12233=CARTESIAN_POINT ( 'NONE',  ( -11.04724669754545729, 20.25032463904771163, -21.46035140199475322 ) ) ;
#12234=CARTESIAN_POINT ( 'NONE',  ( -11.59581746604265184, -16.91849113041673647, -29.30341980017526993 ) ) ;
#12237=ORIENTED_EDGE ( 'NONE', *, *, #25247, .F. ) ;
#12238=CARTESIAN_POINT ( 'NONE',  ( -34.01910795266670817, -9.469880945013516182, -9.355061796818153752 ) ) ;
#12239=CARTESIAN_POINT ( 'NONE',  ( -9.320207966883044648, -18.25898334416423197, -30.00000000000000000 ) ) ;
#12242=CARTESIAN_POINT ( 'NONE',  ( 25.83939409753097749, 1.310542756611064785, -15.53056140694106091 ) ) ;
#12247=CARTESIAN_POINT ( 'NONE',  ( -20.82134614922586024, 0.7609143916134510910, -26.82519756432694180 ) ) ;
#12248=VERTEX_POINT ( 'NONE', #32746 ) ;
#12249=CARTESIAN_POINT ( 'NONE',  ( 32.63163926239240453, -2.293081498025231202, -6.377226414710281510 ) ) ;
#12250=FACE_OUTER_BOUND ( 'NONE', #8331, .T. ) ;
#12253=CARTESIAN_POINT ( 'NONE',  ( -20.41719577202367475, 3.595984569019347710, -27.00753783791186535 ) ) ;
#12254=LINE ( 'NONE', #30752, #13840 ) ;
#12267=CARTESIAN_POINT ( 'NONE',  ( -22.24749944600915441, 6.755814336694140110, -16.88571461955177355 ) ) ;
#12271=CARTESIAN_POINT ( 'NONE',  ( 24.17850601201823935, -26.54311662592617438, -5.883534236263519901 ) ) ;
#12273=CARTESIAN_POINT ( 'NONE',  ( 13.91919597197520808, 24.20150807187953390, -13.48820975930131461 ) ) ;
#12275=CARTESIAN_POINT ( 'NONE',  ( -12.55985620789771318, 17.00768640634399276, -25.16950739431023365 ) ) ;
#12278=CARTESIAN_POINT ( 'NONE',  ( 14.54626310194416305, 24.93267370481178347, -11.60010698176134447 ) ) ;
#12282=CARTESIAN_POINT ( 'NONE',  ( -13.38683417315264279, 23.02748639848019607, -15.42644061306512171 ) ) ;
#12284=CARTESIAN_POINT ( 'NONE',  ( -15.64016700958762307, -26.70521847281657202, -6.413594158090527131 ) ) ;
#12287=CARTESIAN_POINT ( 'NONE',  ( -19.79882239781932540, -9.636344326736496768, -24.23038216571381653 ) ) ;
#12288=CARTESIAN_POINT ( 'NONE',  ( -9.348295649430010457, -19.45916671671450970, -23.95518150547726322 ) ) ;
#12290=CARTESIAN_POINT ( 'NONE',  ( 16.11351922548164950, 24.44051152376729519, -5.000000000000000888 ) ) ;
#12292=CARTESIAN_POINT ( 'NONE',  ( 26.70883441844552664, 4.675912117059606743, -5.476516349963133301 ) ) ;
#12293=DIRECTION ( 'NONE',  ( 1.000000000000000000, 0.000000000000000000, 0.000000000000000000 ) ) ;
#12297=CARTESIAN_POINT ( 'NONE',  ( -19.72832818285809253, -26.19953226489505127, -9.498077945716184800 ) ) ;
#12299=VERTEX_POINT ( 'NONE', #37583 ) ;
#12300=CARTESIAN_POINT ( 'NONE',  ( -20.87864677930795310, -0.1800933656229730950, -26.75177554836502125 ) ) ;
#12301=CARTESIAN_POINT ( 'NONE',  ( 30.40872510205566925, -0.06348338061482104722, -8.294560979537857648 ) ) ;
#12304=EDGE_LOOP ( 'NONE', ( #12002, #7142 ) ) ;
#12305=CARTESIAN_POINT ( 'NONE',  ( 13.47223693944937750, 18.09844039693851769, -30.00000000000000355 ) ) ;
#12309=EDGE_CURVE ( 'NONE', #10807, #31289, #5702, .T. ) ;
#12312=CARTESIAN_POINT ( 'NONE',  ( 37.48530129358654506, -10.40311727728359692, -5.000000000000010658 ) ) ;
#12313=CARTESIAN_POINT ( 'NONE',  ( 2.706689172267205290, 26.59357338535925308, -18.64150033707969811 ) ) ;
#12314=CYLINDRICAL_SURFACE ( 'NONE', #13323, 17.00000000000000000 ) ;
#12316=DIRECTION ( 'NONE',  ( -0.000000000000000000, -0.000000000000000000, -1.000000000000000000 ) ) ;
#12321=CARTESIAN_POINT ( 'NONE',  ( 13.66396806110179973, 24.77360163986799435, -13.43593853470100186 ) ) ;
#12324=CARTESIAN_POINT ( 'NONE',  ( -15.42551642139064327, 13.50153766309080616, -30.00000000000001421 ) ) ;
#12327=CARTESIAN_POINT ( 'NONE',  ( 11.18307060885532600, -20.46872301250157022, -20.54176180563865373 ) ) ;
#12328=CARTESIAN_POINT ( 'NONE',  ( -21.68568904104562023, -27.13690135270087822, -5.452393508887768192 ) ) ;
#12329=CARTESIAN_POINT ( 'NONE',  ( 15.33694215129139948, 26.62211003415151467, -6.887897498730077395 ) ) ;
#12330=CARTESIAN_POINT ( 'NONE',  ( 15.09448029680397241, 26.16123611564987428, -8.766612590816048822 ) ) ;
#12333=CARTESIAN_POINT ( 'NONE',  ( -9.432189322962019062, -18.20121415529274600, -29.34969478843057544 ) ) ;
#12335=CARTESIAN_POINT ( 'NONE',  ( -15.95852086734116071, -13.25472829660814789, -27.74404909499182637 ) ) ;
#12336=CARTESIAN_POINT ( 'NONE',  ( 1.306219793455511313, -21.01157610766281891, -24.41760533827341817 ) ) ;
#12337=CARTESIAN_POINT ( 'NONE',  ( 15.39253874130542776, 25.56879223000222723, -8.303194391403303953 ) ) ;
#12338=CARTESIAN_POINT ( 'NONE',  ( 21.87469278667276384, 10.95211447422776985, -9.392538902003625623 ) ) ;
#12340=CARTESIAN_POINT ( 'NONE',  ( -3.458130042104726076, 20.20612265101129168, -29.99999999999998579 ) ) ;
#12342=CARTESIAN_POINT ( 'NONE',  ( -34.46511719672074747, -5.518907050001597092, -5.451568486426576321 ) ) ;
#12343=EDGE_CURVE ( 'NONE', #17337, #26123, #1830, .T. ) ;
#12349=CARTESIAN_POINT ( 'NONE',  ( -20.93293132456442152, 1.148100751203120939, -26.25406389234631988 ) ) ;
#12350=CARTESIAN_POINT ( 'NONE',  ( 33.48600411488287421, -13.44844601827948694, -9.747306394059473078 ) ) ;
#12358=DIRECTION ( 'NONE',  ( -1.000000000000000000, 0.000000000000000000, 0.000000000000000000 ) ) ;
#12361=CARTESIAN_POINT ( 'NONE',  ( -2.233363292134739275, 27.76951152815063395, -17.61292157057414443 ) ) ;
#12366=CARTESIAN_POINT ( 'NONE',  ( 18.06868231757531618, -13.86363220686757458, -23.03522161772968957 ) ) ;
#12367=CARTESIAN_POINT ( 'NONE',  ( 19.62469028259190651, 14.57143679938034353, -10.37640014583656978 ) ) ;
#12368=CARTESIAN_POINT ( 'NONE',  ( 8.965364566908062827, 21.09711902998411404, -22.32596467695269382 ) ) ;
#12369=EDGE_LOOP ( 'NONE', ( #37726, #4002 ) ) ;
#12371=CARTESIAN_POINT ( 'NONE',  ( -20.70514017605514923, 13.67614408150934580, -5.967130309997563664 ) ) ;
#12373=CARTESIAN_POINT ( 'NONE',  ( 13.83086666455825053, -24.13364333532040007, -13.50291250830041889 ) ) ;
#12376=CARTESIAN_POINT ( 'NONE',  ( -8.937590682902627037, -20.71651963383551731, -21.24786896499727007 ) ) ;
#12378=CARTESIAN_POINT ( 'NONE',  ( -12.37187468849621474, 20.51614643895100087, -19.49228216629809651 ) ) ;
#12379=CARTESIAN_POINT ( 'NONE',  ( -24.87088375429694054, -26.22384022550785687, -6.313645004022516716 ) ) ;
#12380=CARTESIAN_POINT ( 'NONE',  ( 8.607094368180748134, -18.65170925544331126, -28.74046143688874366 ) ) ;
#12383=CARTESIAN_POINT ( 'NONE',  ( -11.00990894457517477, 33.49669252407993270, -7.634107675710282592 ) ) ;
#12391=CARTESIAN_POINT ( 'NONE',  ( 27.71930269395751623, 0.2145384403578754484, -13.51489228889109029 ) ) ;
#12395=CARTESIAN_POINT ( 'NONE',  ( -30.57930627834187831, 0.02004245076167957690, -7.358024370966995242 ) ) ;
#12398=CARTESIAN_POINT ( 'NONE',  ( 34.34316617829726681, -7.172350984383295547, -8.073188482078531791 ) ) ;
#12406=DIRECTION ( 'NONE',  ( 1.000000000000000000, 0.000000000000000000, -0.000000000000000000 ) ) ;
#12413=CARTESIAN_POINT ( 'NONE',  ( 5.157905742752888045, 22.93259919978908457, -21.98816088478811182 ) ) ;
#12414=AXIS2_PLACEMENT_3D ( 'NONE', #30262, #36956, #9121 ) ;
#12417=CARTESIAN_POINT ( 'NONE',  ( 15.60024655210046163, -23.09233175402551197, -15.20950988053776420 ) ) ;
#12422=CARTESIAN_POINT ( 'NONE',  ( -15.35173535111459131, 26.57026200220170509, -6.888001712493197815 ) ) ;
#12424=CARTESIAN_POINT ( 'NONE',  ( 15.17959409457666098, -26.46972997935209904, -7.358350661662780290 ) ) ;
#12426=LINE ( 'NONE', #24818, #34758 ) ;
#12429=CARTESIAN_POINT ( 'NONE',  ( -13.93864121817066248, 26.51574797513629989, -11.48636496174305499 ) ) ;
#12430=CARTESIAN_POINT ( 'NONE',  ( -13.98800961053418490, -21.23703842434798972, -18.20997924916034805 ) ) ;
#12433=CARTESIAN_POINT ( 'NONE',  ( -29.12014979997558228, -9.039752278382179540, -14.83108018992303023 ) ) ;
#12434=CARTESIAN_POINT ( 'NONE',  ( -9.523195312559730397, -18.67992273108535528, -26.24930059924759718 ) ) ;
#12437=CARTESIAN_POINT ( 'NONE',  ( 22.66673786582151706, 0.8234316233675766927, -21.64362386725597176 ) ) ;
#12442=CARTESIAN_POINT ( 'NONE',  ( -23.32581642294337598, 0.5282185752115819977, -20.53879718575241142 ) ) ;
#12444=CARTESIAN_POINT ( 'NONE',  ( 23.80926127916344726, -0.9845178533687296563, -20.33980794348563492 ) ) ;
#12451=CARTESIAN_POINT ( 'NONE',  ( -26.19606766578834467, 4.393075645995596190, -9.799521558767215978 ) ) ;
#12454=CARTESIAN_POINT ( 'NONE',  ( -18.87179230188976220, -27.32956261471019133, -4.999999999999999112 ) ) ;
#12460=CARTESIAN_POINT ( 'NONE',  ( -19.88990440888141009, 6.451044192260599885, -25.43228481840965216 ) ) ;
#12461=DIRECTION ( 'NONE',  ( 1.000000000000000000, 0.000000000000000000, 0.000000000000000000 ) ) ;
#12464=CARTESIAN_POINT ( 'NONE',  ( 16.74526845675677578, -17.41194385859613902, -20.93759567407294853 ) ) ;
#12466=CARTESIAN_POINT ( 'NONE',  ( 14.85865438977763375, 26.03933603557532095, -9.695787514185630229 ) ) ;
#12468=CARTESIAN_POINT ( 'NONE',  ( -13.10226789136070380, 16.53484623785779561, -25.23106048629698961 ) ) ;
#12472=CARTESIAN_POINT ( 'NONE',  ( 14.86387305504814726, 25.53751346079465989, -10.18168596463881137 ) ) ;
#12476=CARTESIAN_POINT ( 'NONE',  ( -12.53799127256666956, 21.22453523357990335, -18.42692599694124667 ) ) ;
#12478=CARTESIAN_POINT ( 'NONE',  ( -13.56363600825507199, -23.64209565141708325, -14.45832144993096691 ) ) ;
#12481=CARTESIAN_POINT ( 'NONE',  ( -34.55317057183779639, -15.49588746005725959, -7.124090691308525791 ) ) ;
#12482=CARTESIAN_POINT ( 'NONE',  ( -11.15263382927128966, -25.10807195756887467, -9.767712422240766301 ) ) ;
#12484=CARTESIAN_POINT ( 'NONE',  ( 14.12418929389014011, 20.63997023270749054, -16.57871110594469855 ) ) ;
#12486=CARTESIAN_POINT ( 'NONE',  ( 25.71414162338313858, 4.640216332958793544, -10.78049592915970400 ) ) ;
#12490=DIRECTION ( 'NONE',  ( -0.000000000000000000, -0.000000000000000000, -1.000000000000000000 ) ) ;
#12492=CARTESIAN_POINT ( 'NONE',  ( -25.40327909237853632, 0.02527255523525553590, -17.39221788563712678 ) ) ;
#12493=EDGE_CURVE ( 'NONE', #7370, #31948, #24526, .T. ) ;
#12494=CARTESIAN_POINT ( 'NONE',  ( 25.38697857826957005, 0.05609946110438526062, -17.39619723301043663 ) ) ;
#12501=CARTESIAN_POINT ( 'NONE',  ( 19.79815887584821610, 19.84782313723624370, -5.000000000000007994 ) ) ;
#12507=LINE ( 'NONE', #40136, #30513 ) ;
#12508=CARTESIAN_POINT ( 'NONE',  ( 37.48538792151179422, -11.24999995791135809, -5.000000000000002665 ) ) ;
#12509=CARTESIAN_POINT ( 'NONE',  ( 2.647469807785585605, 36.69595272411527986, -9.286360570462178998 ) ) ;
#12519=CARTESIAN_POINT ( 'NONE',  ( 14.40253865757656904, 26.32860937628373676, -10.59413652422460217 ) ) ;
#12523=CARTESIAN_POINT ( 'NONE',  ( -18.56076843189209313, 17.44795389765408444, -8.382486478387699336 ) ) ;
#12526=CARTESIAN_POINT ( 'NONE',  ( 9.796177435753577356, -18.55921797199988532, -26.22383286036198768 ) ) ;
#12527=CARTESIAN_POINT ( 'NONE',  ( -22.70315127378580300, -26.84338220279167331, -6.331427942688537591 ) ) ;
#12528=CARTESIAN_POINT ( 'NONE',  ( 10.99090272494190046, 17.30462611091308034, -30.00000000000000711 ) ) ;
#12529=CARTESIAN_POINT ( 'NONE',  ( 15.36357391709072040, 26.70243454889372003, -6.416728717100916413 ) ) ;
#12532=CARTESIAN_POINT ( 'NONE',  ( -15.23883232513551533, -26.48425076293248281, -7.358141420259828536 ) ) ;
#12535=CARTESIAN_POINT ( 'NONE',  ( -27.45201627647075426, -18.96585292318375693, -12.89829047187982525 ) ) ;
#12536=CARTESIAN_POINT ( 'NONE',  ( -0.3875490619503205725, -24.70434061326229269, -6.939883883725533664 ) ) ;
#12537=CARTESIAN_POINT ( 'NONE',  ( 11.46070356447341076, 17.55389630813125024, -26.25396252495082905 ) ) ;
#12538=CARTESIAN_POINT ( 'NONE',  ( 21.01290135064779463, 10.57244385225932781, -13.90025499387392216 ) ) ;
#12542=CARTESIAN_POINT ( 'NONE',  ( -20.35866630304074221, -2.409458700188494618, -29.28927096481215031 ) ) ;
#12549=CARTESIAN_POINT ( 'NONE',  ( -21.20053173203535835, 1.290506853206223381, -25.06817133786373475 ) ) ;
#12550=CARTESIAN_POINT ( 'NONE',  ( 19.65282344174659457, -6.596692726057402645, -27.76040915297549461 ) ) ;
#12561=CARTESIAN_POINT ( 'NONE',  ( -3.812539336066663065, 34.03298746155307697, -11.98968657202452448 ) ) ;
#12562=CYLINDRICAL_SURFACE ( 'NONE', #31456, 18.00000000000003553 ) ;
#12568=CARTESIAN_POINT ( 'NONE',  ( 8.747848026427400114, 18.74166680801365104, -27.94534499906865221 ) ) ;
#12570=CARTESIAN_POINT ( 'NONE',  ( -20.71763460597477291, 13.68537009249746461, -4.999999999999996447 ) ) ;
#12572=CARTESIAN_POINT ( 'NONE',  ( 15.55607442552794950, -26.68487202370114630, -6.414919209907756326 ) ) ;
#12573=CARTESIAN_POINT ( 'NONE',  ( 37.48557158514984167, -11.25000000000009237, 3.000000000000000000 ) ) ;
#12574=CARTESIAN_POINT ( 'NONE',  ( 10.93327523444657778, 17.34109439532409525, -29.99999999999999289 ) ) ;
#12575=CARTESIAN_POINT ( 'NONE',  ( 21.88499642459564143, -5.528038495964486820, -29.99999999999998224 ) ) ;
#12577=CARTESIAN_POINT ( 'NONE',  ( -11.15585325849543707, 17.77692559745511858, -26.22179184702690691 ) ) ;
#12579=CARTESIAN_POINT ( 'NONE',  ( -25.75211752115588126, -25.63936478115028450, -7.167472985298198651 ) ) ;
#12580=CARTESIAN_POINT ( 'NONE',  ( 8.739015621761494046, -22.16521160953498182, -17.72474713041751215 ) ) ;
#12581=CARTESIAN_POINT ( 'NONE',  ( 11.07558645076263737, 17.30325621831820371, -28.70984248050030985 ) ) ;
#12582=CARTESIAN_POINT ( 'NONE',  ( 22.56924115802582875, -16.29358669976124219, -17.62083569142466288 ) ) ;
#12585=CARTESIAN_POINT ( 'NONE',  ( -7.826018490237524716, 23.62355187122631506, -19.93686502536784033 ) ) ;
#12587=EDGE_CURVE ( 'NONE', #38149, #27435, #29714, .T. ) ;
#12592=CARTESIAN_POINT ( 'NONE',  ( 22.72806502780237992, 0.6194066608261846740, -21.61851103361042803 ) ) ;
#12594=CARTESIAN_POINT ( 'NONE',  ( 11.06069781764610305, 34.19033620402622375, -5.000000000000000888 ) ) ;
#12597=CARTESIAN_POINT ( 'NONE',  ( -28.85991493692416299, 0.1377318499120018247, -11.60034766336565504 ) ) ;
#12600=CARTESIAN_POINT ( 'NONE',  ( 32.11642246959483771, -5.701442053666191612, -11.24895573057437481 ) ) ;
#12601=( GEOMETRIC_REPRESENTATION_CONTEXT ( 3 ) GLOBAL_UNCERTAINTY_ASSIGNED_CONTEXT ( ( #4703 ) ) GLOBAL_UNIT_ASSIGNED_CONTEXT ( ( #37207, #30717, #34164 ) ) REPRESENTATION_CONTEXT ( 'NONE', 'WORKASPACE' ) );
#12605=DIRECTION ( 'NONE',  ( 1.000000000000000000, 0.000000000000000000, 0.000000000000000000 ) ) ;
#12608=VECTOR ( 'NONE', #2377, 1000.000000000000000 ) ;
#12612=CARTESIAN_POINT ( 'NONE',  ( -18.30496497598766581, 9.321025232647617287, -29.99999999999999289 ) ) ;
#12618=CARTESIAN_POINT ( 'NONE',  ( 4.627278376603056742, 20.58541896761892431, -26.35737439622670664 ) ) ;
#12619=CARTESIAN_POINT ( 'NONE',  ( 10.75002496752869341, -17.64495920642993454, -28.01020103939122308 ) ) ;
#12624=CARTESIAN_POINT ( 'NONE',  ( -15.11672449564866128, 26.08808756446744681, -8.768129095627141822 ) ) ;
#12626=CARTESIAN_POINT ( 'NONE',  ( 14.58906216886622431, -25.77273076839362886, -9.713267811317372491 ) ) ;
#12630=CARTESIAN_POINT ( 'NONE',  ( -11.71558024193440062, 23.44492113552537660, -17.20205828893062616 ) ) ;
#12632=CARTESIAN_POINT ( 'NONE',  ( -15.73389691588134376, -22.37440482904794337, -16.14369830803590844 ) ) ;
#12637=CARTESIAN_POINT ( 'NONE',  ( -27.20412735585551900, -7.570742992334142940, -16.78134040425078410 ) ) ;
#12638=CARTESIAN_POINT ( 'NONE',  ( -13.24729829976488205, -23.61164488198660294, -14.48312679232910760 ) ) ;
#12641=CARTESIAN_POINT ( 'NONE',  ( 21.67083567045098746, 0.9273911989265315459, -23.87724168837842242 ) ) ;
#12646=CARTESIAN_POINT ( 'NONE',  ( -22.23112559094391827, 0.6234443325065696095, -22.72982244255366524 ) ) ;
#12648=CARTESIAN_POINT ( 'NONE',  ( 20.55275704333539011, -0.2804796770642928316, -28.66667438445236726 ) ) ;
#12649=CARTESIAN_POINT ( 'NONE',  ( 17.84039878628271936, -10.10400010744520571, -30.00000000000005329 ) ) ;
#12652=CARTESIAN_POINT ( 'NONE',  ( -20.85387373749717810, 4.297652806957183103, -24.19551209732460606 ) ) ;
#12661=CARTESIAN_POINT ( 'NONE',  ( -19.69137326279327027, 5.702251777040514114, -30.00000000000000355 ) ) ;
#12664=CARTESIAN_POINT ( 'NONE',  ( 23.94622488899277712, -26.31671797062173113, -7.190667588222269480 ) ) ;
#12666=CARTESIAN_POINT ( 'NONE',  ( 10.97710528508702765, 17.90433831621321303, -26.20245233466055623 ) ) ;
#12668=CARTESIAN_POINT ( 'NONE',  ( -14.77449872868504421, 22.25468481093715312, -13.59554605823010931 ) ) ;
#12671=CARTESIAN_POINT ( 'NONE',  ( 12.42496545568594968, 20.44575147035703822, -19.50238972058703268 ) ) ;
#12675=CARTESIAN_POINT ( 'NONE',  ( -15.02016821374818534, 26.40324407494122028, -8.755937702507523568 ) ) ;
#12677=CARTESIAN_POINT ( 'NONE',  ( -15.46270586958304172, -26.44519224899418575, -7.820922189861058804 ) ) ;
#12680=CARTESIAN_POINT ( 'NONE',  ( -23.75646719861951439, -12.44796170920469613, -18.61696717325561323 ) ) ;
#12681=CARTESIAN_POINT ( 'NONE',  ( -14.16578816422650711, -25.94200127604465678, -8.776735216617021607 ) ) ;
#12683=CARTESIAN_POINT ( 'NONE',  ( 14.11166830150711426, 19.77494500827953772, -17.62012407019295779 ) ) ;
#12684=ORIENTED_EDGE ( 'NONE', *, *, #32149, .T. ) ;
#12685=CARTESIAN_POINT ( 'NONE',  ( 19.82805615916967312, 5.207665154685881426, -30.00000000000000355 ) ) ;
#12691=CARTESIAN_POINT ( 'NONE',  ( -21.32151666823140701, 0.4344076493211833645, -24.97710971221515663 ) ) ;
#12692=CARTESIAN_POINT ( 'NONE',  ( 25.34039414564677983, 0.1439692079819893111, -17.40756292650477022 ) ) ;
#12696=CARTESIAN_POINT ( 'NONE',  ( 5.636483973512840251, -22.01575377102106046, -21.50719306941234876 ) ) ;
#12702=CARTESIAN_POINT ( 'NONE',  ( 3.826396457843638022, 37.43840591691041908, -7.552972810893269440 ) ) ;
#12703=DIRECTION ( 'NONE',  ( -1.000000000000000000, 0.000000000000000000, 0.000000000000000000 ) ) ;
#12711=CARTESIAN_POINT ( 'NONE',  ( 10.15111435463817280, 17.86907098534008043, -28.67154087780474470 ) ) ;
#12715=CARTESIAN_POINT ( 'NONE',  ( -15.04174557779704635, 14.20451568885117588, -27.10768944337526065 ) ) ;
#12721=CARTESIAN_POINT ( 'NONE',  ( 9.562392075367188937, -18.27749775416154066, -28.07786222914176477 ) ) ;
#12723=CARTESIAN_POINT ( 'NONE',  ( -19.98910163558307573, -25.17004345428989609, -11.28674626201566511 ) ) ;
#12724=CARTESIAN_POINT ( 'NONE',  ( 15.33919115406833278, 26.61414219747821619, -6.888072233219839191 ) ) ;
#12725=CARTESIAN_POINT ( 'NONE',  ( 13.75833282284662751, 23.42126009408847409, -14.47362935452958155 ) ) ;
#12728=CARTESIAN_POINT ( 'NONE',  ( -15.16405052498309836, -26.37334731087130990, -7.828243992827849773 ) ) ;
#12730=CARTESIAN_POINT ( 'NONE',  ( -16.15747483659607298, -12.61697622026560772, -30.00000000000000711 ) ) ;
#12731=CARTESIAN_POINT ( 'NONE',  ( -2.540214017920780165, -24.49585459483449412, -8.898735351503297863 ) ) ;
#12732=CARTESIAN_POINT ( 'NONE',  ( 15.75662360411219787, 25.59993261007102561, -4.999999999999999112 ) ) ;
#12733=CARTESIAN_POINT ( 'NONE',  ( 20.75214263285785421, 9.441152523992672130, -16.96792007788538115 ) ) ;
#12736=CARTESIAN_POINT ( 'NONE',  ( -28.94549850962602378, -2.870772275164490850, -14.18330164410991401 ) ) ;
#12740=ADVANCED_FACE ( 'NONE', ( #20707 ), #33305, .T. ) ;
#12743=CARTESIAN_POINT ( 'NONE',  ( -27.43844334215360448, 0.5923872920799873043, -13.53615638127614318 ) ) ;
#12744=CARTESIAN_POINT ( 'NONE',  ( 35.11830485971632498, -14.14517689978181103, -6.284369114096038267 ) ) ;
#12747=AXIS2_PLACEMENT_3D ( 'NONE', #7176, #296, #3932 ) ;
#12756=CARTESIAN_POINT ( 'NONE',  ( -3.992774750912768678, 35.67860805316688300, -10.18623164847826423 ) ) ;
#12764=CARTESIAN_POINT ( 'NONE',  ( 13.73220224370217579, 30.78478150535875457, -5.457670766714417532 ) ) ;
#12766=CARTESIAN_POINT ( 'NONE',  ( -17.99203688690355207, 9.826896140120286560, -29.99999999999999289 ) ) ;
#12768=CARTESIAN_POINT ( 'NONE',  ( 9.772342709178570175, -18.26604441824505187, -27.43687354787681087 ) ) ;
#12770=CARTESIAN_POINT ( 'NONE',  ( 14.81731930227308425, 25.68027610000711292, -10.17593115926348091 ) ) ;
#12771=CARTESIAN_POINT ( 'NONE',  ( 35.36940577612500647, -20.42053594592276866, -4.999999999999997335 ) ) ;
#12775=CARTESIAN_POINT ( 'NONE',  ( -20.65407906065966515, -20.62528606208020321, -15.83079615351305058 ) ) ;
#12776=CARTESIAN_POINT ( 'NONE',  ( 9.344820083231123675, -20.32964934627687015, -21.78656791573911633 ) ) ;
#12777=CARTESIAN_POINT ( 'NONE',  ( 13.59683655979047145, 22.61026046561213576, -15.46554287034021158 ) ) ;
#12778=CARTESIAN_POINT ( 'NONE',  ( 29.83403652028378517, -20.21430139748671806, -10.17890540654461695 ) ) ;
#12782=CARTESIAN_POINT ( 'NONE',  ( -7.438509353473058638, 24.90914914033339755, -18.85218860379452366 ) ) ;
#12788=CARTESIAN_POINT ( 'NONE',  ( 21.70460829199038244, 0.7520035140130953977, -23.85688495828296496 ) ) ;
#12794=CARTESIAN_POINT ( 'NONE',  ( -30.86332187973009056, -0.0005132856539958949174, -4.999999999999999112 ) ) ;
#12797=CARTESIAN_POINT ( 'NONE',  ( 29.92351859954650095, -6.183656610847034329, -13.99975621931235636 ) ) ;
#12805=ORIENTED_EDGE ( 'NONE', *, *, #31466, .T. ) ;
#12807=CARTESIAN_POINT ( 'NONE',  ( -20.39749650821323712, -2.159697320963449130, -30.00000000000000355 ) ) ;
#12812=CARTESIAN_POINT ( 'NONE',  ( 13.91075386486431320, 15.49308367278315046, -26.46882179040325056 ) ) ;
#12814=CARTESIAN_POINT ( 'NONE',  ( 5.194277563714346790, 20.21734125709076224, -27.07613456391705853 ) ) ;
#12816=CARTESIAN_POINT ( 'NONE',  ( 13.32124143939226713, -19.97798892781937141, -20.26999631390010848 ) ) ;
#12820=CARTESIAN_POINT ( 'NONE',  ( -14.93905414659889352, 25.78616324827421735, -9.709672390330473135 ) ) ;
#12822=CARTESIAN_POINT ( 'NONE',  ( 9.420782162276523763, -18.34804325365140798, -28.08566532578938180 ) ) ;
#12826=AXIS2_PLACEMENT_3D ( 'NONE', #11824, #30522, #2682 ) ;
#12827=CARTESIAN_POINT ( 'NONE',  ( -13.71280609171516218, 27.90080846771834544, -10.50245461074293196 ) ) ;
#12828=CARTESIAN_POINT ( 'NONE',  ( -11.29934442612571388, -17.60818932157431149, -26.68958922436052106 ) ) ;
#12833=CARTESIAN_POINT ( 'NONE',  ( -20.38661749552379732, -6.361484682545848202, -25.69238726493766833 ) ) ;
#12834=CARTESIAN_POINT ( 'NONE',  ( -10.13786778044513959, -19.19472683054627637, -23.86456005356567545 ) ) ;
#12837=CARTESIAN_POINT ( 'NONE',  ( 21.53391398595842077, 1.629941546267092756, -23.95798976520841705 ) ) ;
#12841=ORIENTED_EDGE ( 'NONE', *, *, #11042, .T. ) ;
#12843=CARTESIAN_POINT ( 'NONE',  ( -28.91287382066377631, 0.07518806480736967002, -11.59674810764759201 ) ) ;
#12846=CARTESIAN_POINT ( 'NONE',  ( 31.83309823342235489, -1.783519987017442077, -8.218906981704529713 ) ) ;
#12847=CARTESIAN_POINT ( 'NONE',  ( 19.82764311455687078, -5.383684237423299379, -29.99999999999997513 ) ) ;
#12859=CARTESIAN_POINT ( 'NONE',  ( -23.50810587197001311, 8.940726895909143934, -6.932906322231784380 ) ) ;
#12860=CARTESIAN_POINT ( 'NONE',  ( 20.78048496889905650, -24.27834333958334412, -12.16204984203799988 ) ) ;
#12863=CARTESIAN_POINT ( 'NONE',  ( 15.35355722042785054, 26.91131673440186844, -5.944390809853191904 ) ) ;
#12865=CARTESIAN_POINT ( 'NONE',  ( -13.53391903102045113, 18.98539088064760705, -19.68245357048784783 ) ) ;
#12869=CARTESIAN_POINT ( 'NONE',  ( 14.55518902956964666, 24.90832010759994120, -11.60082918595498036 ) ) ;
#12873=CARTESIAN_POINT ( 'NONE',  ( -12.27358052226857765, 20.64665722953253635, -19.47164098058547665 ) ) ;
#12875=CARTESIAN_POINT ( 'NONE',  ( -15.63755959170095089, -26.78052150289263622, -5.000000000000000888 ) ) ;
#12878=CARTESIAN_POINT ( 'NONE',  ( -34.54285066864272835, -16.78341526201209533, -5.000000000000000000 ) ) ;
#12879=CARTESIAN_POINT ( 'NONE',  ( -13.78313613767150692, -25.73547777514550106, -9.253468020048730480 ) ) ;
#12881=CARTESIAN_POINT ( 'NONE',  ( 12.67230126945890412, 16.91222923427146085, -25.18277393341357850 ) ) ;
#12883=CARTESIAN_POINT ( 'NONE',  ( 19.64403038794415224, 5.908213622717614300, -29.41334968421891816 ) ) ;
#12889=CARTESIAN_POINT ( 'NONE',  ( -21.36309669107243892, 0.09765983062926059111, -24.94016949773846292 ) ) ;
#12892=CARTESIAN_POINT ( 'NONE',  ( 20.48743909015156106, 0.7225425954259894201, -30.00000000000000000 ) ) ;
#12895=ORIENTED_EDGE ( 'NONE', *, *, #12587, .T. ) ;
#12897=CARTESIAN_POINT ( 'NONE',  ( -16.77267017469754151, -29.13948811618693924, -5.000000000000000000 ) ) ;
#12903=CARTESIAN_POINT ( 'NONE',  ( 4.462315839921594751, 27.28163392174084123, -17.66356109337273494 ) ) ;
#12912=CARTESIAN_POINT ( 'NONE',  ( 10.62804704006517653, 18.54916539939932463, -24.92187189847329165 ) ) ;
#12916=CARTESIAN_POINT ( 'NONE',  ( -18.31827171329678450, 17.14654578878874602, -10.34362890045172279 ) ) ;
#12919=CARTESIAN_POINT ( 'NONE',  ( 10.82536310076888952, -19.99331871519654769, -21.61878681921504608 ) ) ;
#12921=CARTESIAN_POINT ( 'NONE',  ( 11.31067235875530130, 18.03752733997335511, -25.01467926984602030 ) ) ;
#12922=CARTESIAN_POINT ( 'NONE',  ( 12.64338984711987379, 21.06830844464534991, -18.45004776435698446 ) ) ;
#12927=CARTESIAN_POINT ( 'NONE',  ( -15.37705579490140195, -26.68840604134194194, -5.946092059939837249 ) ) ;
#12929=CARTESIAN_POINT ( 'NONE',  ( -17.04493828242456033, -12.50648979017474538, -26.27989544973046421 ) ) ;
#12930=CARTESIAN_POINT ( 'NONE',  ( -3.977639621222068378, -22.37851689048354942, -17.96835865857241643 ) ) ;
#12931=CARTESIAN_POINT ( 'NONE',  ( 11.52998930085336937, 17.50220035821725162, -26.26108509606446617 ) ) ;
#12933=CARTESIAN_POINT ( 'NONE',  ( 21.27561741872812462, 9.625452138548039827, -14.90836893165563914 ) ) ;
#12937=CARTESIAN_POINT ( 'NONE',  ( -32.22282324793545172, -3.298326783855909827, -9.525552920251982414 ) ) ;
#12943=CARTESIAN_POINT ( 'NONE',  ( -21.22731311515731534, 1.116805269015000990, -25.05052939645603516 ) ) ;
#12944=CARTESIAN_POINT ( 'NONE',  ( 22.78213498135489701, -9.193927964998984237, -20.75049135688346169 ) ) ;
#12955=CARTESIAN_POINT ( 'NONE',  ( -2.308138231165596466, 21.01458932961489978, -26.27989553671341483 ) ) ;
#12956=DIRECTION ( 'NONE',  ( -0.000000000000000000, -0.000000000000000000, -1.000000000000000000 ) ) ;
#12961=CARTESIAN_POINT ( 'NONE',  ( 13.01198037208728842, 31.38676150821800803, -7.241395499289373205 ) ) ;
#12963=CARTESIAN_POINT ( 'NONE',  ( -19.72377957101126711, 11.77771347321402651, -15.94900687590660660 ) ) ;
#12966=CARTESIAN_POINT ( 'NONE',  ( 15.04210785476277934, -26.00471334787457067, -9.235286766544799519 ) ) ;
#12968=CARTESIAN_POINT ( 'NONE',  ( 11.07830671788882881, 17.64536026459691342, -26.82601358146755999 ) ) ;
#12969=CARTESIAN_POINT ( 'NONE',  ( 37.49625565938770677, -14.69322820095493221, -4.999999999999991118 ) ) ;
#12972=CARTESIAN_POINT ( 'NONE',  ( -26.86432650658507271, -25.19322975956973920, -6.728586538145628460 ) ) ;
#12973=CARTESIAN_POINT ( 'NONE',  ( 8.383450201187182316, -25.09682772003503359, -7.878769048704421074 ) ) ;
#12974=CARTESIAN_POINT ( 'NONE',  ( 15.16724506842761500, 25.92448480984241144, -8.769736773116987294 ) ) ;
#12975=CARTESIAN_POINT ( 'NONE',  ( 27.61701753510086021, -18.71320982384436959, -12.89761149929025663 ) ) ;
#12980=CARTESIAN_POINT ( 'NONE',  ( -8.453943144716905778, 36.13191751627968529, -5.441173800798977389 ) ) ;
#12984=CARTESIAN_POINT ( 'NONE',  ( 23.95345493350577826, 0.4562929689794089083, -19.49228041339053519 ) ) ;
#12989=CARTESIAN_POINT ( 'NONE',  ( -30.75477483822581348, 0.007422296481196848095, -6.417047845488035307 ) ) ;
#12992=CARTESIAN_POINT ( 'NONE',  ( 23.50924913396118399, -4.123401132657353862, -21.07160444102285268 ) ) ;
#13004=CARTESIAN_POINT ( 'NONE',  ( -19.88226695332659588, 5.007750446913723508, -30.00000000000000000 ) ) ;
#13008=CARTESIAN_POINT ( 'NONE',  ( 14.33908007195274692, 14.82388666928050647, -27.64946332230921655 ) ) ;
#13009=CARTESIAN_POINT ( 'NONE',  ( 8.982065559873033678, 34.94785179831643518, -8.031862189828427034 ) ) ;
#13013=CARTESIAN_POINT ( 'NONE',  ( 11.89829529493479221, -20.33063158364313239, -20.44835590138199066 ) ) ;
#13017=CARTESIAN_POINT ( 'NONE',  ( -11.90856329309679218, 19.36478525622990787, -21.61991777980233920 ) ) ;
#13019=CARTESIAN_POINT ( 'NONE',  ( 13.25977140536878807, -23.61272118971784906, -14.48244016720286176 ) ) ;
#13020=DIRECTION ( 'NONE',  ( -0.000000000000000000, -0.000000000000000000, -1.000000000000000000 ) ) ;
#13023=CARTESIAN_POINT ( 'NONE',  ( -8.851921390983532589, 18.49121495627866452, -29.99999999999998579 ) ) ;
#13026=CARTESIAN_POINT ( 'NONE',  ( -32.71123478963491493, -10.14810845015363050, -11.13421304303691350 ) ) ;
#13027=CARTESIAN_POINT ( 'NONE',  ( -9.881661346875441509, -18.84796558037550795, -25.02421141044853670 ) ) ;
#13030=CARTESIAN_POINT ( 'NONE',  ( 30.21135594116120160, 0.1457432374558486343, -8.299147896465123964 ) ) ;
#13033=VECTOR ( 'NONE', #7667, 1000.000000000000000 ) ;
#13035=CARTESIAN_POINT ( 'NONE',  ( -27.18275240598519815, 0.1768051309694248507, -14.47033692342836098 ) ) ;
#13038=CARTESIAN_POINT ( 'NONE',  ( 26.73663087904732905, -1.280630175484808397, -16.25687896506618557 ) ) ;
#13046=VECTOR ( 'NONE', #23604, 1000.000000000000000 ) ;
#13050=CARTESIAN_POINT ( 'NONE',  ( -21.63082554306499716, 8.459712576583205745, -15.90695635898583404 ) ) ;
#13051=CARTESIAN_POINT ( 'NONE',  ( 17.08717224709219451, -21.22693275917435329, -16.97485990036564729 ) ) ;
#13054=CARTESIAN_POINT ( 'NONE',  ( 10.86351183210297400, 17.43903252575687546, -28.70101831061248987 ) ) ;
#13056=CARTESIAN_POINT ( 'NONE',  ( -12.17604136976394358, 17.00510967891084135, -26.32489337626220660 ) ) ;
#13059=CARTESIAN_POINT ( 'NONE',  ( 14.95773614117678996, 25.72884227512856370, -9.710064219024593157 ) ) ;
#13061=CARTESIAN_POINT ( 'NONE',  ( 19.59609834480663082, -10.05714783815784052, -24.22289641939408256 ) ) ;
#13064=CARTESIAN_POINT ( 'NONE',  ( -11.03568212627763678, 17.86295559657867216, -26.20877666994450550 ) ) ;
#13066=CARTESIAN_POINT ( 'NONE',  ( -14.04776079454142490, -23.13890183802322653, -15.34726994745094686 ) ) ;
#13070=CARTESIAN_POINT ( 'NONE',  ( -33.15023676467436786, -14.84419029601833806, -9.736194267565831950 ) ) ;
#13071=CARTESIAN_POINT ( 'NONE',  ( -11.58176784450557761, -22.04669522693308181, -17.49831374786357330 ) ) ;
#13073=CARTESIAN_POINT ( 'NONE',  ( 16.22052397401369461, 22.81938114578490584, -8.804735524812913994 ) ) ;
#13075=CARTESIAN_POINT ( 'NONE',  ( 26.70883441844552664, 4.675912117059606743, -5.000000000000001776 ) ) ;
#13081=CARTESIAN_POINT ( 'NONE',  ( -21.03058350190238457, 0.1347426989242972717, -26.16529232141537875 ) ) ;
#13083=CARTESIAN_POINT ( 'NONE',  ( 30.22740896235442776, -0.2270326147911990722, -9.222382858374048809 ) ) ;
#13087=CARTESIAN_POINT ( 'NONE',  ( -13.28992586503615847, -18.25382200079944539, -30.00000000000000711 ) ) ;
#13094=CARTESIAN_POINT ( 'NONE',  ( 3.503322964093031455, 26.44893706114941523, -18.65895197296932650 ) ) ;
#13095=DIRECTION ( 'NONE',  ( 1.000000000000000000, 0.000000000000000000, -0.000000000000000000 ) ) ;
#13099=CARTESIAN_POINT ( 'NONE',  ( 28.63180867286471809, -22.06108345148580696, -9.744445364747779337 ) ) ;
#13101=ADVANCED_FACE ( 'NONE', ( #31631, #3799 ), #10100, .T. ) ;
#13102=CARTESIAN_POINT ( 'NONE',  ( -14.23945615837876311, -31.58416516429889853, 3.000000000000000000 ) ) ;
#13106=CARTESIAN_POINT ( 'NONE',  ( 14.93523343043905882, 27.03121972480990820, -8.269414059510982185 ) ) ;
#13109=CARTESIAN_POINT ( 'NONE',  ( -16.11915739853855811, 18.74155883991118898, -14.73719238174496127 ) ) ;
#13112=AXIS2_PLACEMENT_3D ( 'NONE', #31731, #19536, #16293 ) ;
#13113=CARTESIAN_POINT ( 'NONE',  ( 9.950384810341901698, -18.82026468017858889, -25.01640556310974972 ) ) ;
#13115=CARTESIAN_POINT ( 'NONE',  ( 15.37331383236014126, 26.66785149480303119, -6.417008027727837849 ) ) ;
#13116=VERTEX_POINT ( 'NONE', #38126 ) ;
#13117=CARTESIAN_POINT ( 'NONE',  ( 14.73499465698446009, 25.40345112443975495, -10.65306111367642927 ) ) ;
#13120=CARTESIAN_POINT ( 'NONE',  ( -15.08926872483068315, -26.26244385881013699, -8.298346565395871011 ) ) ;
#13122=CARTESIAN_POINT ( 'NONE',  ( -16.73268231713828058, -12.27567335498239842, -27.72086002018244599 ) ) ;
#13123=CARTESIAN_POINT ( 'NONE',  ( -4.261170676688491810, -23.24522659430452265, -14.87884297781055842 ) ) ;
#13124=CARTESIAN_POINT ( 'NONE',  ( 13.01467249004550020, 20.52916449794418696, -18.51329633673889674 ) ) ;
#13125=ORIENTED_EDGE ( 'NONE', *, *, #31466, .F. ) ;
#13126=CARTESIAN_POINT ( 'NONE',  ( 22.62620251215892253, 10.10101068805073865, -7.914309724494427378 ) ) ;
#13130=CARTESIAN_POINT ( 'NONE',  ( -33.78064619886176700, -4.467697089185144854, -6.796441298519896534 ) ) ;
#13136=CYLINDRICAL_SURFACE ( 'NONE', #19276, 18.00000000000000000 ) ;
#13139=CARTESIAN_POINT ( 'NONE',  ( 32.85715722811898587, -14.37096278579205411, -10.18737089092998538 ) ) ;
#13145=CARTESIAN_POINT ( 'NONE',  ( -34.47241746879593904, 3.460351812918829761, 0.000000000000000000 ) ) ;
#13150=CARTESIAN_POINT ( 'NONE',  ( -1.226217677998840516, 24.65685218365392828, -20.69626040025250902 ) ) ;
#13156=CARTESIAN_POINT ( 'NONE',  ( 10.61980620388852969, 20.62470325590637898, -21.39191359161199202 ) ) ;
#13159=CARTESIAN_POINT ( 'NONE',  ( -18.06822122341611347, 9.865462442820332356, -27.73584775015774539 ) ) ;
#13162=CARTESIAN_POINT ( 'NONE',  ( 15.51572609547548254, -26.72387080533473380, -5.945569791504813573 ) ) ;
#13165=CARTESIAN_POINT ( 'NONE',  ( 13.73891004957165940, 23.46505885318682516, -14.46902604110928969 ) ) ;
#13166=CARTESIAN_POINT ( 'NONE',  ( -16.84920187454419960, 29.09530251867925443, -13.79123840944734170 ) ) ;
#13168=CARTESIAN_POINT ( 'NONE',  ( -25.11387969369502215, -25.04874519970718083, -8.917861276085261579 ) ) ;
#13169=CARTESIAN_POINT ( 'NONE',  ( 7.004305706416510624, -19.31551653162770776, -30.00000000000000000 ) ) ;
#13170=CARTESIAN_POINT ( 'NONE',  ( 15.49934645862682103, 26.48612375915841710, -4.999999999999998224 ) ) ;
#13171=CARTESIAN_POINT ( 'NONE',  ( 16.84105033895882642, -12.12787018219099089, -27.71828030521067632 ) ) ;
#13176=CARTESIAN_POINT ( 'NONE',  ( -8.269738542359823086, 35.15571153379752900, -8.458646650837764014 ) ) ;
#13180=CARTESIAN_POINT ( 'NONE',  ( 29.37565202589770763, 0.04982724068811738433, -10.65280254111669045 ) ) ;
#13184=CARTESIAN_POINT ( 'NONE',  ( -21.27098901970252598, 0.8144016237283049353, -25.01870527535232469 ) ) ;
#13185=CARTESIAN_POINT ( 'NONE',  ( -20.14086772481481447, -26.69671823294502744, -8.145045411856523643 ) ) ;
#13188=CARTESIAN_POINT ( 'NONE',  ( 35.24432775889728475, -8.480040233932975013, -5.445055975222005351 ) ) ;
#13200=CARTESIAN_POINT ( 'NONE',  ( 8.088808017670798378, 18.84043440346156473, -29.99999999999999645 ) ) ;
#13203=CARTESIAN_POINT ( 'NONE',  ( 17.30437301942612294, 17.82039300084830202, -12.79526519019998432 ) ) ;
#13204=CARTESIAN_POINT ( 'NONE',  ( 7.825189179823995644, 30.28281593568562258, -13.92036688199892680 ) ) ;
#13208=CARTESIAN_POINT ( 'NONE',  ( 12.48152888332789878, -21.43928621844884574, -18.38220065339488940 ) ) ;
#13212=CARTESIAN_POINT ( 'NONE',  ( -15.36719073388214341, 26.68956433499065994, -6.416937597740959731 ) ) ;
#13215=CARTESIAN_POINT ( 'NONE',  ( 11.84140825053389001, -22.03755937975082446, -17.47623322197002338 ) ) ;
#13221=CARTESIAN_POINT ( 'NONE',  ( -9.391599613247716860, 21.62240220123701917, -21.21144781721583072 ) ) ;
#13225=CARTESIAN_POINT ( 'NONE',  ( -20.24777750044549762, -4.334933572263888202, -27.83540287325038776 ) ) ;
#13228=CARTESIAN_POINT ( 'NONE',  ( 30.72030077726637032, 0.1104180286406396816, -5.946111898128993545 ) ) ;
#13229=CARTESIAN_POINT ( 'NONE',  ( 10.98647152928294446, 17.30743895948372213, -29.99999999999999289 ) ) ;
#13230=CARTESIAN_POINT ( 'NONE',  ( -12.33616729053609795, -27.99489201236593061, -4.999999999999999112 ) ) ;
#13233=CARTESIAN_POINT ( 'NONE',  ( -27.74642324427214390, 0.1782721915882912456, -13.51284498012490509 ) ) ;
#13236=CARTESIAN_POINT ( 'NONE',  ( 27.66764765329071807, -1.745514196759363035, -15.23339469188658235 ) ) ;
#13238=CARTESIAN_POINT ( 'NONE',  ( 11.56212933365550377, 16.94202105496415456, -30.00000000000001421 ) ) ;
#13253=CARTESIAN_POINT ( 'NONE',  ( -23.53973944703488286, 8.948669315374337074, -6.448443132398569588 ) ) ;
#13254=CARTESIAN_POINT ( 'NONE',  ( 19.67723955058091789, -23.00962397103849000, -14.03145724330032529 ) ) ;
#13258=CARTESIAN_POINT ( 'NONE',  ( 14.67936663452034907, 25.57073318950553542, -10.64181656390416286 ) ) ;
#13260=CARTESIAN_POINT ( 'NONE',  ( -15.03545123130942507, 24.54682575326017968, -10.67232211706494560 ) ) ;
#13263=CARTESIAN_POINT ( 'NONE',  ( 11.50520882153597846, 18.41930897395437938, -23.85713326318693106 ) ) ;
#13265=CARTESIAN_POINT ( 'NONE',  ( 33.70372332681250782, -18.58847439657466083, -4.999999999999997335 ) ) ;
#13268=CARTESIAN_POINT ( 'NONE',  ( -12.18834851601500269, 20.75798833321451653, -19.45407312999939009 ) ) ;
#13270=CARTESIAN_POINT ( 'NONE',  ( -12.06810631748702178, -20.91201952217128834, -19.43044751594679909 ) ) ;
#13273=CARTESIAN_POINT ( 'NONE',  ( -18.70070976566389831, -8.421454915599365876, -29.21689156567847334 ) ) ;
#13274=CARTESIAN_POINT ( 'NONE',  ( -14.25032268057046991, -26.07042913507176962, -8.304725559915748789 ) ) ;
#13276=CARTESIAN_POINT ( 'NONE',  ( 15.94966356142663777, 23.22048705160648652, -9.275927655557403284 ) ) ;
#13278=CARTESIAN_POINT ( 'NONE',  ( 26.66957287664490295, 3.773598562717486615, -9.786777780698315610 ) ) ;
#13279=DIRECTION ( 'NONE',  ( 0.000000000000000000, 0.000000000000000000, 1.000000000000000000 ) ) ;
#13282=CARTESIAN_POINT ( 'NONE',  ( -30.34199328301418674, -0.3569055445810484506, -9.214469955534525525 ) ) ;
#13283=AXIS2_PLACEMENT_3D ( 'NONE', #29217, #10941, #26975 ) ;
#13284=CARTESIAN_POINT ( 'NONE',  ( 21.76708849998995277, 0.4128473488999230834, -23.81551767858415047 ) ) ;
#13289=CARTESIAN_POINT ( 'NONE',  ( 15.72991998290128990, -16.18894361744929000, -29.99999999999998579 ) ) ;
#13296=LINE ( 'NONE', #29348, #19835 ) ;
#13300=CARTESIAN_POINT ( 'NONE',  ( 17.80350308363193079, -15.45044821450308703, -21.94968374958370916 ) ) ;
#13305=CARTESIAN_POINT ( 'NONE',  ( 14.02888686415674613, 25.13130688616161734, -12.49550152463516284 ) ) ;
#13308=CARTESIAN_POINT ( 'NONE',  ( -16.32417823649820932, 19.06887375611960067, -13.74019203237465625 ) ) ;
#13311=EDGE_CURVE ( 'NONE', #31854, #37897, #33045, .T. ) ;
#13312=CARTESIAN_POINT ( 'NONE',  ( 13.68675488944363394, -24.11442831246780472, -13.51430495698268253 ) ) ;
#13314=CARTESIAN_POINT ( 'NONE',  ( 11.47989394144907216, 18.44111857959351752, -23.85327845104777467 ) ) ;
#13316=CARTESIAN_POINT ( 'NONE',  ( 13.20572627864892290, 22.24225191886345598, -16.44350126499534426 ) ) ;
#13319=CARTESIAN_POINT ( 'NONE',  ( -13.44580646965103377, 22.90880309117785529, -15.44002879919819193 ) ) ;
#13321=CARTESIAN_POINT ( 'NONE',  ( -9.545403281521043226, -18.28601644545607030, -28.07880677660388358 ) ) ;
#13323=AXIS2_PLACEMENT_3D ( 'NONE', #34645, #28147, #12703 ) ;
#13326=CARTESIAN_POINT ( 'NONE',  ( -30.24448231779780372, -20.88974531296291914, -9.287890822320301609 ) ) ;
#13327=CARTESIAN_POINT ( 'NONE',  ( -4.167622576179086380, -22.95801459329689820, -15.90121958565441496 ) ) ;
#13328=CARTESIAN_POINT ( 'NONE',  ( 11.53991419820319919, 17.31783527090524899, -26.86815565160901897 ) ) ;
#13330=CARTESIAN_POINT ( 'NONE',  ( 21.49103779673273706, 8.702945238107675507, -15.91587550759767211 ) ) ;
#13331=CARTESIAN_POINT ( 'NONE',  ( 35.34645969586885172, -13.68099284068201982, -4.999999999999999112 ) ) ;
#13334=CARTESIAN_POINT ( 'NONE',  ( -30.42670526058322267, -3.055756317512598130, -12.29337351708506532 ) ) ;
#13340=EDGE_CURVE ( 'NONE', #2291, #35955, #36908, .T. ) ;
#13341=CARTESIAN_POINT ( 'NONE',  ( 26.48686316033968779, -11.60226487929934436, -16.65552626896159083 ) ) ;
#13348=CARTESIAN_POINT ( 'NONE',  ( -22.71238962429393382, 10.21442836285774902, -4.999999999999995559 ) ) ;
#13353=CARTESIAN_POINT ( 'NONE',  ( -1.024090966498643951, 20.73153308134275719, -27.70753136508054126 ) ) ;
#13361=CARTESIAN_POINT ( 'NONE',  ( 14.15549368817671372, 29.61663025949119188, -6.828959041903970295 ) ) ;
#13362=ADVANCED_FACE ( 'NONE', ( #12250 ), #30943, .T. ) ;
#13363=LINE ( 'NONE', #10320, #25679 ) ;
#13365=CARTESIAN_POINT ( 'NONE',  ( -17.63781053724814640, 11.42380641143947884, -24.41185227018100434 ) ) ;
#13369=CARTESIAN_POINT ( 'NONE',  ( 14.11138780488941435, -24.62265220140333355, -12.54540560345105860 ) ) ;
#13371=CARTESIAN_POINT ( 'NONE',  ( 11.45548560297930329, 18.46219990532805966, -23.84939050765756363 ) ) ;
#13372=CARTESIAN_POINT ( 'NONE',  ( -15.29245034862075769, 32.56469986091995850, -4.999999999999987566 ) ) ;
#13374=CARTESIAN_POINT ( 'NONE',  ( -22.41958926254718776, -23.75709256622344512, -12.10280908274594758 ) ) ;
#13375=CARTESIAN_POINT ( 'NONE',  ( 6.261531442577396689, -25.09448364857072633, -5.479386318545421020 ) ) ;
#13376=CARTESIAN_POINT ( 'NONE',  ( 15.48317245491042904, 26.45281331046393092, -5.946134839014572293 ) ) ;
#13377=CARTESIAN_POINT ( 'NONE',  ( 20.42207822710955512, -13.80760592411458454, -20.70725840310820232 ) ) ;
#13381=CARTESIAN_POINT ( 'NONE',  ( -7.784904364235317509, 29.15186949039238229, -14.87099986184792222 ) ) ;
#13386=CARTESIAN_POINT ( 'NONE',  ( 21.71688145637667233, 0.6875768534851390834, -23.84913670212286618 ) ) ;
#13391=CARTESIAN_POINT ( 'NONE',  ( -21.26491060988546167, 0.8575210262421062435, -25.02329962371140581 ) ) ;
#13394=CARTESIAN_POINT ( 'NONE',  ( 28.13023995446271286, -6.686838264236121709, -15.87225043224434806 ) ) ;
#13404=PRESENTATION_STYLE_ASSIGNMENT (( #37993 ) ) ;
#13405=CARTESIAN_POINT ( 'NONE',  ( -16.55039525318069593, 12.10030840459738499, -30.00000000000001066 ) ) ;
#13408=CARTESIAN_POINT ( 'NONE',  ( 15.38089657270912092, 16.48686376672722531, -19.92077768951681804 ) ) ;
#13410=CARTESIAN_POINT ( 'NONE',  ( 10.81548165185368404, 33.90032711218825767, -7.190669018737369633 ) ) ;
#13414=EDGE_CURVE ( 'NONE', #1290, #23669, #28621, .T. ) ;
#13415=CARTESIAN_POINT ( 'NONE',  ( 10.24602814327722555, -18.35173801110022040, -26.18014820733107939 ) ) ;
#13419=CARTESIAN_POINT ( 'NONE',  ( -11.02092554839851068, 17.33857933006403229, -28.70757483433319024 ) ) ;
#13421=CARTESIAN_POINT ( 'NONE',  ( 10.89336905877927464, -20.52105068520159037, -20.57499638152730270 ) ) ;
#13425=CARTESIAN_POINT ( 'NONE',  ( -10.54481009990373330, 22.58364347488284096, -19.17416471084009189 ) ) ;
#13426=CARTESIAN_POINT ( 'NONE',  ( -12.79957067206351162, -17.39491784009856090, -24.68155700537461072 ) ) ;
#13428=CARTESIAN_POINT ( 'NONE',  ( -33.60037199511394590, -8.295775768378332415, -9.823597468572941693 ) ) ;
#13431=CARTESIAN_POINT ( 'NONE',  ( 21.26058458131393891, 0.8877849191941595830, -25.02650145224686895 ) ) ;
#13435=CARTESIAN_POINT ( 'NONE',  ( -24.56473081290029015, 0.4207215009515258841, -18.45078781038499471 ) ) ;
#13438=CARTESIAN_POINT ( 'NONE',  ( 20.63680471757680124, -0.9487772221450848642, -27.98716435451661511 ) ) ;
#13447=DIRECTION ( 'NONE',  ( 0.000000000000000000, 0.000000000000000000, 1.000000000000000000 ) ) ;
#13454=CARTESIAN_POINT ( 'NONE',  ( -19.94779647907517983, 8.036049150339344749, -22.20456094153029625 ) ) ;
#13455=CARTESIAN_POINT ( 'NONE',  ( 12.98122511323041550, -16.28336372442720403, -27.20012430218251964 ) ) ;
#13458=CARTESIAN_POINT ( 'NONE',  ( 10.84452725066743106, 17.39679239189240434, -30.00000000000000000 ) ) ;
#13461=CARTESIAN_POINT ( 'NONE',  ( -12.07501055264735257, 16.79091931427930007, -27.52101582733411078 ) ) ;
#13466=CARTESIAN_POINT ( 'NONE',  ( 13.80613653353328196, 23.31784988260643132, -14.48073358026558211 ) ) ;
#13468=CARTESIAN_POINT ( 'NONE',  ( 20.80092188569423328, -11.47548207259838193, -21.83916146562154736 ) ) ;
#13472=CARTESIAN_POINT ( 'NONE',  ( -11.30680158603337482, 18.58912957429523871, -23.82584604873158085 ) ) ;
#13474=CARTESIAN_POINT ( 'NONE',  ( -14.80989234766682472, -24.23948810107563645, -13.42031711412986539 ) ) ;
#13478=CARTESIAN_POINT ( 'NONE',  ( -22.69874938501649098, -9.396075009901352360, -20.74577302956173241 ) ) ;
#13479=CARTESIAN_POINT ( 'NONE',  ( -13.22797251932733431, -24.88283229560302701, -11.63121411976873532 ) ) ;
#13481=CARTESIAN_POINT ( 'NONE',  ( 16.39331781465299898, 19.66495602315241698, -12.73500833637442398 ) ) ;
#13483=CARTESIAN_POINT ( 'NONE',  ( 27.43674297377669546, 3.779828424379618301, -5.475541599305136842 ) ) ;
#13487=CARTESIAN_POINT ( 'NONE',  ( -31.09037572277983230, -0.2342870890902534753, -4.999999999999999112 ) ) ;
#13488=CARTESIAN_POINT ( 'NONE',  ( 31.42341880231480644, -0.5937245782808076022, -5.000000000000000888 ) ) ;
#13492=CARTESIAN_POINT ( 'NONE',  ( -27.08779848459120743, 7.221796966026721165, -5.000000000000006217 ) ) ;
#13494=AXIS2_PLACEMENT_3D ( 'NONE', #7039, #3996, #16397 ) ;
#13507=CARTESIAN_POINT ( 'NONE',  ( 27.35186887652132626, -23.80825151756206637, -8.882026785022988591 ) ) ;
#13510=CARTESIAN_POINT ( 'NONE',  ( 12.95942736264239947, 22.68428619808883795, -16.38842958060721244 ) ) ;
#13513=CARTESIAN_POINT ( 'NONE',  ( -17.16260375762833590, 18.73914433653179756, -11.78407945085863062 ) ) ;
#13516=CARTESIAN_POINT ( 'NONE',  ( 9.512694695443267179, -18.20982909230496816, -28.70727928411922392 ) ) ;
#13519=CARTESIAN_POINT ( 'NONE',  ( 15.34485063204045829, 26.59437119930156967, -6.887952992160583321 ) ) ;
#13521=CARTESIAN_POINT ( 'NONE',  ( 14.28551598028751890, 24.48525218155484851, -12.54977972690513077 ) ) ;
#13523=CARTESIAN_POINT ( 'NONE',  ( -11.64607099366300780, 18.95003504881763590, -22.72817784514300143 ) ) ;
#13525=CARTESIAN_POINT ( 'NONE',  ( -12.27294156613012177, -22.02301600987046371, -17.43937061174498027 ) ) ;
#13529=CARTESIAN_POINT ( 'NONE',  ( -25.34274736433472697, -16.37843956862553085, -15.68371574493890286 ) ) ;
#13530=CARTESIAN_POINT ( 'NONE',  ( -6.988245995732859761, -25.03642915341433905, -7.403757448750240222 ) ) ;
#13531=CARTESIAN_POINT ( 'NONE',  ( 15.63852180243771528, 25.36448989093083384, -7.362413517827306464 ) ) ;
#13532=ORIENTED_EDGE ( 'NONE', *, *, #4858, .T. ) ;
#13533=CARTESIAN_POINT ( 'NONE',  ( 22.92399774901786458, 9.099773806377163154, -9.874741973018776875 ) ) ;
#13539=CARTESIAN_POINT ( 'NONE',  ( -32.91670029435780265, -2.547476605001916194, -5.917534263431005748 ) ) ;
#13545=CARTESIAN_POINT ( 'NONE',  ( 32.57092086225112837, -15.43378303256681505, -10.17932366030892588 ) ) ;
#13555=CARTESIAN_POINT ( 'NONE',  ( -1.740872439423108764, 34.41729727890611912, -11.97610320120729632 ) ) ;
#13562=CARTESIAN_POINT ( 'NONE',  ( 14.07960931274568672, 28.37400713639219418, -9.127921161272693595 ) ) ;
#13565=CARTESIAN_POINT ( 'NONE',  ( -16.95965515916876498, 11.87563068946122158, -26.61073229064057699 ) ) ;
#13568=CARTESIAN_POINT ( 'NONE',  ( 13.77482710089912210, -24.12599296267502069, -13.50787276857876229 ) ) ;
#13570=CARTESIAN_POINT ( 'NONE',  ( 12.90549922656808413, 21.69123041792454032, -17.43238391223398764 ) ) ;
#13571=CARTESIAN_POINT ( 'NONE',  ( -16.24796006241077961, 15.88921519459651499, -30.00000000000001421 ) ) ;
#13572=DIRECTION ( 'NONE',  ( -1.000000000000000000, 0.000000000000000000, 0.000000000000000000 ) ) ;
#13574=CARTESIAN_POINT ( 'NONE',  ( -25.65315598498527194, -24.12413061561075622, -9.790106673725071929 ) ) ;
#13575=CARTESIAN_POINT ( 'NONE',  ( 6.952732471630988620, -22.26205726029128584, -17.83880605057320423 ) ) ;
#13576=CARTESIAN_POINT ( 'NONE',  ( 15.46210322845357155, 26.52717532233935316, -5.946118077167572125 ) ) ;
#13577=CARTESIAN_POINT ( 'NONE',  ( 20.20733478970500840, 13.69637775999485640, -9.885393215995732064 ) ) ;
#13581=CARTESIAN_POINT ( 'NONE',  ( -6.014539584152595708, 22.60354644530256607, -22.04821685920930463 ) ) ;
#13586=CARTESIAN_POINT ( 'NONE',  ( 28.90646526158858265, 0.08205528372900385004, -11.59832840213325866 ) ) ;
#13592=CARTESIAN_POINT ( 'NONE',  ( -20.81252836718331167, 0.8663108682335884936, -26.83334811610091464 ) ) ;
#13594=ORIENTED_EDGE ( 'NONE', *, *, #17970, .F. ) ;
#13595=CARTESIAN_POINT ( 'NONE',  ( 35.44138113946621615, -9.599287445864765900, -5.000000000000010658 ) ) ;
#13610=CARTESIAN_POINT ( 'NONE',  ( 13.76818825652920353, 15.24450382255247050, -28.80311538815760031 ) ) ;
#13611=CARTESIAN_POINT ( 'NONE',  ( 5.765122233821920794, 19.89527052026323517, -27.81238314162991898 ) ) ;
#13614=DIRECTION ( 'NONE',  ( -1.000000000000000000, 0.000000000000000000, 0.000000000000000000 ) ) ;
#13616=CARTESIAN_POINT ( 'NONE',  ( 15.49271691873735968, -25.80169155014763405, -10.13838130885175559 ) ) ;
#13623=CARTESIAN_POINT ( 'NONE',  ( -12.65871080218516731, 21.04530515263928336, -18.45346255153580373 ) ) ;
#13625=CARTESIAN_POINT ( 'NONE',  ( 13.65683774811633455, -24.55498886789716551, -12.56460507296711349 ) ) ;
#13630=CARTESIAN_POINT ( 'NONE',  ( -9.954087448707369390, 21.17613213146948681, -21.29198274210564534 ) ) ;
#13633=CARTESIAN_POINT ( 'NONE',  ( -19.98679978234304144, -4.924167105727923044, -28.51946357198569970 ) ) ;
#13635=ORIENTED_EDGE ( 'NONE', *, *, #32717, .F. ) ;
#13636=CARTESIAN_POINT ( 'NONE',  ( 21.67939327573176911, 0.8834818022177464147, -23.87219493357654443 ) ) ;
#13641=CARTESIAN_POINT ( 'NONE',  ( -20.61058943125449971, 0.8469614167685917128, -28.07733840680127813 ) ) ;
#13645=CARTESIAN_POINT ( 'NONE',  ( 32.29748657415021995, -3.057573243849562861, -9.081205313942463775 ) ) ;
#13660=CARTESIAN_POINT ( 'NONE',  ( -21.05291937318205342, 8.312515282553865958, -17.97409977038949691 ) ) ;
#13661=CARTESIAN_POINT ( 'NONE',  ( 12.82234224798668976, -16.09375609578110655, -28.57231939863815739 ) ) ;
#13663=CARTESIAN_POINT ( 'NONE',  ( 11.80270328479468311, 19.47748869397488392, -21.59992045479478762 ) ) ;
#13665=CARTESIAN_POINT ( 'NONE',  ( -11.79678012972095047, 16.99765053083067556, -27.50177182085873540 ) ) ;
#13668=CARTESIAN_POINT ( 'NONE',  ( 14.31934378920023043, 24.39963677761549121, -12.55310820702660557 ) ) ;
#13670=CARTESIAN_POINT ( 'NONE',  ( 33.16930538569719999, -19.62507065308114917, -5.435330440035552435 ) ) ;
#13671=ADVANCED_FACE ( 'NONE', ( #784 ), #28412, .T. ) ;
#13675=CARTESIAN_POINT ( 'NONE',  ( -12.51073218500047801, 21.26417290573970220, -18.42108626876654043 ) ) ;
#13677=CARTESIAN_POINT ( 'NONE',  ( -16.20081666663972797, -26.89087236765021061, -5.938530992383368456 ) ) ;
#13680=CARTESIAN_POINT ( 'NONE',  ( -18.93673219582609946, -7.851978407254149417, -30.00000000000000711 ) ) ;
#13681=CARTESIAN_POINT ( 'NONE',  ( -9.018257521923398912, -18.41052938026230024, -29.35785334563086835 ) ) ;
#13683=CARTESIAN_POINT ( 'NONE',  ( 13.48020054446795868, 16.18221087160424432, -25.26925449299266901 ) ) ;
#13685=CARTESIAN_POINT ( 'NONE',  ( 20.70282115146825319, 3.793121191063287156, -25.28431974125459192 ) ) ;
#13689=CARTESIAN_POINT ( 'NONE',  ( -20.53452984402690973, 0.6885224814544792515, -28.70101917630290345 ) ) ;
#13690=CARTESIAN_POINT ( 'NONE',  ( 31.01929709654494260, -0.7441688249631136509, -8.261849393656827800 ) ) ;
#13695=CARTESIAN_POINT ( 'NONE',  ( -22.50952045769495413, 1.338071129232386802, -21.70479210668387182 ) ) ;
#13696=CARTESIAN_POINT ( 'NONE',  ( -3.091399026088746727, 22.35909668862748134, -19.80438750953544513 ) ) ;
#13707=CARTESIAN_POINT ( 'NONE',  ( 23.17521898255445834, -20.18490097291412155, -14.80311732295303351 ) ) ;
#13710=CARTESIAN_POINT ( 'NONE',  ( 12.90714127504553055, 22.77320297353917411, -16.37761627767333650 ) ) ;
#13714=CARTESIAN_POINT ( 'NONE',  ( -14.15788581485469422, 15.50092647220509612, -25.32911243468907614 ) ) ;
#13718=CARTESIAN_POINT ( 'NONE',  ( 9.465986449187253626, -18.23380396764607525, -28.70911249201515147 ) ) ;
#13719=LINE ( 'NONE', #19216, #18523 ) ;
#13720=CARTESIAN_POINT ( 'NONE',  ( 14.94370345678945888, 25.77223918896596189, -9.709399778286011085 ) ) ;
#13722=CARTESIAN_POINT ( 'NONE',  ( 12.13093762266853837, 19.92385368760829323, -20.54106352598588003 ) ) ;
#13724=CARTESIAN_POINT ( 'NONE',  ( -12.89788825750088819, 21.70392749762217122, -17.43064730788859507 ) ) ;
#13726=CARTESIAN_POINT ( 'NONE',  ( -11.50915682881853286, -20.98128273221263029, -19.50078698021883028 ) ) ;
#13728=CARTESIAN_POINT ( 'NONE',  ( -32.85619107660216542, -19.84207158267233595, -6.275925487822830995 ) ) ;
#13729=CARTESIAN_POINT ( 'NONE',  ( -1.793625933065454037, -20.61433429535822626, -27.17456019479941176 ) ) ;
#13730=CARTESIAN_POINT ( 'NONE',  ( 15.21005260476538190, 24.06451757296145999, -10.68341754272937649 ) ) ;
#13733=CARTESIAN_POINT ( 'NONE',  ( 23.94499769980229686, 8.291951293815612800, -6.930188724025407865 ) ) ;
#13736=CARTESIAN_POINT ( 'NONE',  ( 5.023663291607745940, -24.92826071495466067, -5.000000000000003553 ) ) ;
#13740=CARTESIAN_POINT ( 'NONE',  ( -21.07773708785227740, -1.860215743600160287, -25.99199685066085053 ) ) ;
#13746=CARTESIAN_POINT ( 'NONE',  ( 19.01366704504291150, -7.688495684904649963, -30.00000000000000355 ) ) ;
#13753=DIRECTION ( 'NONE',  ( 0.000000000000000000, 0.000000000000000000, 1.000000000000000000 ) ) ;
#13755=CARTESIAN_POINT ( 'NONE',  ( -1.059180177458202587, 21.41711868205623048, -25.58062077214095353 ) ) ;
#13762=CARTESIAN_POINT ( 'NONE',  ( 10.92821648837030679, 22.20508130926659263, -19.23066798073530848 ) ) ;
#13766=CARTESIAN_POINT ( 'NONE',  ( -19.70096002242896560, 14.23449510804272755, -10.87519445515239980 ) ) ;
#13770=CARTESIAN_POINT ( 'NONE',  ( 15.34394143031894409, -26.51021667783368230, -7.357393351511376522 ) ) ;
#13772=CARTESIAN_POINT ( 'NONE',  ( 15.00437511166292026, 26.01395306337788682, -9.236044269556060726 ) ) ;
#13773=CARTESIAN_POINT ( 'NONE',  ( -37.62663912510979003, -8.659558992827880886, -5.000000000000002665 ) ) ;
#13776=CARTESIAN_POINT ( 'NONE',  ( -26.34173717234437362, -23.36365984272380203, -10.22141036450111429 ) ) ;
#13778=CARTESIAN_POINT ( 'NONE',  ( 5.271459200338986406, -22.64434140958651653, -16.88279759715859640 ) ) ;
#13779=CARTESIAN_POINT ( 'NONE',  ( 15.07084970125951884, 25.38295622438022647, -9.715434860296623398 ) ) ;
#13780=CARTESIAN_POINT ( 'NONE',  ( 16.84128903688015200, 12.06818854907147021, -26.60985204580989105 ) ) ;
#13784=CARTESIAN_POINT ( 'NONE',  ( -8.090184229333063470, 34.30791569506543226, -9.788502965324324734 ) ) ;
#13786=CARTESIAN_POINT ( 'NONE',  ( -10.71251757019364348, -20.01999408326420493, -21.63251431787718460 ) ) ;
#13793=CARTESIAN_POINT ( 'NONE',  ( -24.51383308242704118, 0.5270737306155055535, -18.46259585337534403 ) ) ;
#13795=CARTESIAN_POINT ( 'NONE',  ( 34.31841886132467323, -8.208541541968717326, -8.495077349752200746 ) ) ;
#13806=CARTESIAN_POINT ( 'NONE',  ( -17.78456945130773192, -10.21696681478616497, -30.00000000000002487 ) ) ;
#13809=CARTESIAN_POINT ( 'NONE',  ( 14.79081071437772010, 14.21365739191439737, -30.00000000000000711 ) ) ;
#13811=CARTESIAN_POINT ( 'NONE',  ( 7.223745109598073810, 25.00395250381602708, -18.84027392568900083 ) ) ;
#13815=CARTESIAN_POINT ( 'NONE',  ( 15.60062348926549092, -25.63540424016351338, -10.59428648563043041 ) ) ;
#13816=CARTESIAN_POINT ( 'NONE',  ( 37.57549957648898697, 32.94422479542058824, 0.000000000000000000 ) ) ;
#13818=ADVANCED_FACE ( 'NONE', ( #25959 ), #22711, .F. ) ;
#13820=CARTESIAN_POINT ( 'NONE',  ( -11.18155517836364510, 17.75836668469307611, -26.22458058910422452 ) ) ;
#13822=CARTESIAN_POINT ( 'NONE',  ( 9.315390879746241026, -18.48740755290666371, -27.46912605503104032 ) ) ;
#13828=CARTESIAN_POINT ( 'NONE',  ( -13.46828150710210892, 29.48665142929467819, -9.082731696040140079 ) ) ;
#13833=CARTESIAN_POINT ( 'NONE',  ( -31.63542238863247036, -6.840584483190602860, -12.12705934607019209 ) ) ;
#13836=CARTESIAN_POINT ( 'NONE',  ( 25.11743899329887952, 0.5542468427327318370, -17.45589780009234104 ) ) ;
#13840=VECTOR ( 'NONE', #5955, 1000.000000000000000 ) ;
#13842=CARTESIAN_POINT ( 'NONE',  ( -30.48479298233587542, -0.01179609685226120329, -7.827771219771337385 ) ) ;
#13845=CARTESIAN_POINT ( 'NONE',  ( 23.19615353721358630, -1.261022845598870790, -21.37482308967549827 ) ) ;
#13846=AXIS2_PLACEMENT_3D ( 'NONE', #10980, #35155, #13614 ) ;
#13847=CARTESIAN_POINT ( 'NONE',  ( 12.11939247953937659, 16.54781379207330971, -30.00000000000001066 ) ) ;
#13862=CARTESIAN_POINT ( 'NONE',  ( 5.000626697282971378, 37.74343557191168941, -5.437187664831800937 ) ) ;
#13866=CARTESIAN_POINT ( 'NONE',  ( -20.67876391171101247, 10.11988510684650677, -15.94128652130671142 ) ) ;
#13867=CARTESIAN_POINT ( 'NONE',  ( 13.30843957427272173, -15.68464343207989842, -28.55404288184102768 ) ) ;
#13871=CARTESIAN_POINT ( 'NONE',  ( 13.98483810825139528, 24.04469065075334910, -13.50292141766080967 ) ) ;
#13874=CARTESIAN_POINT ( 'NONE',  ( -15.68533655378858249, 25.84264350341399208, -5.474052038806747511 ) ) ;
#13879=CARTESIAN_POINT ( 'NONE',  ( 13.52166927499705018, 22.75664420946326771, -15.45479374845303866 ) ) ;
#13881=CARTESIAN_POINT ( 'NONE',  ( 33.18780228327651827, -18.30041771095959291, -7.544762919428389836 ) ) ;
#13883=CARTESIAN_POINT ( 'NONE',  ( -15.27795965409528556, 27.25395738312943195, -5.471917110302146448 ) ) ;
#13885=CARTESIAN_POINT ( 'NONE',  ( -14.35348050961883182, -24.20068026153264640, -13.45728683335227771 ) ) ;
#13889=CARTESIAN_POINT ( 'NONE',  ( -35.09971422896161641, -14.51120324735615874, -5.860585196400803554 ) ) ;
#13890=CARTESIAN_POINT ( 'NONE',  ( -14.14189504131334374, -25.53275775165994332, -10.19155952056719450 ) ) ;
#13892=CARTESIAN_POINT ( 'NONE',  ( 14.88675176583543802, 17.17549405809297269, -19.86810751864282309 ) ) ;
#13894=CARTESIAN_POINT ( 'NONE',  ( 20.15589419559134754, 3.806103299124593775, -29.39287895154624763 ) ) ;
#13898=CARTESIAN_POINT ( 'NONE',  ( -20.62390181444667547, 0.5954859409029100714, -28.06474670757336654 ) ) ;
#13899=CARTESIAN_POINT ( 'NONE',  ( 29.47994304646902108, -0.6169278861223216337, -11.53523241178914560 ) ) ;
#13903=CARTESIAN_POINT ( 'NONE',  ( -28.39096675370102574, 2.624765294898354195, -5.948919365530221270 ) ) ;
#13904=CARTESIAN_POINT ( 'NONE',  ( 6.155076441694339096, 21.71698211341367468, -20.11584339644708308 ) ) ;
#13911=DIRECTION ( 'NONE',  ( 0.000000000000000000, 0.000000000000000000, 1.000000000000000000 ) ) ;
#13915=CARTESIAN_POINT ( 'NONE',  ( 26.60044679873302442, -24.57989799457884672, -8.454375987971554096 ) ) ;
#13918=CARTESIAN_POINT ( 'NONE',  ( 10.70408546242706826, 17.89813097114894447, -26.79091869943797377 ) ) ;
#13921=CARTESIAN_POINT ( 'NONE',  ( -16.36974882123188024, 17.56213386315149805, -15.79138196246351100 ) ) ;
#13923=CARTESIAN_POINT ( 'NONE',  ( 14.51912842374987456, -25.44048832947288474, -10.65547803431773843 ) ) ;
#13925=CARTESIAN_POINT ( 'NONE',  ( 14.94650803745857459, 25.76355683451345868, -9.709532534900402467 ) ) ;
#13927=CARTESIAN_POINT ( 'NONE',  ( 11.06383671253727563, 17.50867094151858794, -27.44708461513057074 ) ) ;
#13929=CARTESIAN_POINT ( 'NONE',  ( -15.38296630468078874, 26.90060637120896558, -5.000000000000001776 ) ) ;
#13930=CARTESIAN_POINT ( 'NONE',  ( -15.47550425816466380, -26.73936689671932143, -5.474270598677144939 ) ) ;
#13933=CARTESIAN_POINT ( 'NONE',  ( -27.79669695867223211, -16.79236872055855301, -13.80438657369478683 ) ) ;
#13934=CARTESIAN_POINT ( 'NONE',  ( -6.603877609327104103, -24.16432772825694641, -11.80673248872152037 ) ) ;
#13935=CARTESIAN_POINT ( 'NONE',  ( 11.70877560076256962, 16.87668805158687491, -28.73501782286896855 ) ) ;
#13937=CARTESIAN_POINT ( 'NONE',  ( 19.63124566570902019, 8.197596596637488631, -23.30003740157314951 ) ) ;
#13943=CARTESIAN_POINT ( 'NONE',  ( -32.13550794386147658, -2.443358523703948570, -8.649088748501414514 ) ) ;
#13944=CIRCLE ( 'NONE', #14615, 57.00000000000006395 ) ;
#13950=CARTESIAN_POINT ( 'NONE',  ( 27.23312197222509923, -12.91592730962168112, -15.69032973555321853 ) ) ;
#13960=CARTESIAN_POINT ( 'NONE',  ( -1.011306241801402273, 20.48440008317826511, -30.00000000000000711 ) ) ;
#13968=CARTESIAN_POINT ( 'NONE',  ( 12.42842755122037346, 24.68749237541469910, -15.24760426189488172 ) ) ;
#13971=CARTESIAN_POINT ( 'NONE',  ( -19.17049849529148986, 13.78076537144805513, -13.89096179552466914 ) ) ;
#13975=CARTESIAN_POINT ( 'NONE',  ( 15.50471485482113820, -26.74686345152265332, -5.474125567124247027 ) ) ;
#13977=CARTESIAN_POINT ( 'NONE',  ( 13.19104420233710506, 22.26977043259612188, -16.43980447468807782 ) ) ;
#13978=CARTESIAN_POINT ( 'NONE',  ( -27.08779848459120743, 7.221796966026721165, -5.000000000000006217 ) ) ;
#13980=CARTESIAN_POINT ( 'NONE',  ( -22.89426894111359090, -21.54803994364075237, -13.90284137355498828 ) ) ;
#13981=CARTESIAN_POINT ( 'NONE',  ( 4.259257232841775043, -20.22332097882593516, -27.12113025733162530 ) ) ;
#13982=CARTESIAN_POINT ( 'NONE',  ( 11.21461197269842636, 17.30895135427360287, -28.08770296027252655 ) ) ;
#13983=CARTESIAN_POINT ( 'NONE',  ( 20.99822950558156620, 12.93985014994555094, -7.428410497112117206 ) ) ;
#13988=CARTESIAN_POINT ( 'NONE',  ( -5.449788316150806722, 31.42540188369694931, -13.85748977810616545 ) ) ;
#13996=CARTESIAN_POINT ( 'NONE',  ( -30.79543237407852985, 0.06882123448304010294, -4.999999999999999112 ) ) ;
#13998=CARTESIAN_POINT ( 'NONE',  ( 26.15862945001307338, -7.884392761838899588, -17.73711950188741682 ) ) ;
#14014=CARTESIAN_POINT ( 'NONE',  ( 16.55956259488248961, 15.35177602386088402, -18.95873336413509946 ) ) ;
#14015=CARTESIAN_POINT ( 'NONE',  ( 10.66400708477075199, 33.33867412272209663, -8.508697681493581300 ) ) ;
#14019=CARTESIAN_POINT ( 'NONE',  ( 15.84172312148188944, -26.62845490554297001, -7.344013408899289885 ) ) ;
#14023=CARTESIAN_POINT ( 'NONE',  ( -10.98473797697927701, 17.30853926952405075, -29.99999999999999289 ) ) ;
#14026=CARTESIAN_POINT ( 'NONE',  ( 14.83010314187407275, -26.50386704626997414, -6.417717416243527317 ) ) ;
#14032=CARTESIAN_POINT ( 'NONE',  ( -7.785723730699082523, 19.30973503573152072, -27.21076142849720370 ) ) ;
#14035=CARTESIAN_POINT ( 'NONE',  ( -24.35358919934762412, -5.258831719696673623, -19.92280915639523187 ) ) ;
#14038=CARTESIAN_POINT ( 'NONE',  ( 22.71450242014743637, 0.6646934032305609197, -21.62413034359709485 ) ) ;
#14039=CARTESIAN_POINT ( 'NONE',  ( -12.79957064613986084, -17.39491786099972259, -24.68155699886624177 ) ) ;
#14043=CARTESIAN_POINT ( 'NONE',  ( -30.73544637638549659, -0.04073673089017386395, -6.887548030490833639 ) ) ;
#14046=CARTESIAN_POINT ( 'NONE',  ( 33.03334970784698044, -3.164777106519510497, -7.267418744076269199 ) ) ;
#14058=CARTESIAN_POINT ( 'NONE',  ( 2.056640691923212305, 20.39672081104026802, -29.21734360554237497 ) ) ;
#14061=CARTESIAN_POINT ( 'NONE',  ( 14.01931971080170847, -19.72843696819627013, -20.19157926468732356 ) ) ;
#14066=CARTESIAN_POINT ( 'NONE',  ( 15.05470115789045593, 26.29235278780934593, -8.760806541134785519 ) ) ;
#14068=CARTESIAN_POINT ( 'NONE',  ( -15.51364032778053925, 26.43312886238355119, -5.000000000000002665 ) ) ;
#14071=CARTESIAN_POINT ( 'NONE',  ( 15.45734228612143646, 26.63525802094401840, -5.474165804386270651 ) ) ;
#14073=CARTESIAN_POINT ( 'NONE',  ( 17.67655037483637415, -11.18511709101394302, -26.96765970948913349 ) ) ;
#14075=CARTESIAN_POINT ( 'NONE',  ( -13.21556436932873702, 23.35821163730123828, -15.38919888636536015 ) ) ;
#14078=CARTESIAN_POINT ( 'NONE',  ( -12.04589167603010758, -20.30227844483841437, -20.42902932149552342 ) ) ;
#14084=CARTESIAN_POINT ( 'NONE',  ( -34.84681707271400342, -13.17048057206591061, -7.565634217669577666 ) ) ;
#14085=CARTESIAN_POINT ( 'NONE',  ( -14.68723827886567435, -26.16908770772800708, -8.301334212331063611 ) ) ;
#14087=CARTESIAN_POINT ( 'NONE',  ( 17.18319281906964235, 20.94686736314969266, -7.387940685848898070 ) ) ;
#14089=CARTESIAN_POINT ( 'NONE',  ( 20.15589419559134754, 3.806103299124593775, -30.00000000000000711 ) ) ;
#14094=CARTESIAN_POINT ( 'NONE',  ( -30.88772949577154137, -0.1296325399160530301, -6.414922386148385058 ) ) ;
#14095=CARTESIAN_POINT ( 'NONE',  ( 30.67843010612066834, -0.5310868340548599020, -8.737336165245711328 ) ) ;
#14099=CARTESIAN_POINT ( 'NONE',  ( -26.02750893215630512, 1.859127183977640652, -14.58313542125660689 ) ) ;
#14100=CARTESIAN_POINT ( 'NONE',  ( -9.163310636333559245, 20.63632441393290762, -29.99999999999998579 ) ) ;
#14107=DIRECTION ( 'NONE',  ( -0.000000000000000000, -0.000000000000000000, 1.000000000000000000 ) ) ;
#14111=CARTESIAN_POINT ( 'NONE',  ( -20.93756045555672429, 5.794231368335179155, -22.09979801953191014 ) ) ;
#14114=CARTESIAN_POINT ( 'NONE',  ( 15.88542612224667927, -12.95767258840383285, -30.00000000000000711 ) ) ;
#14118=CARTESIAN_POINT ( 'NONE',  ( 13.85193959438362121, 24.35802306960261632, -13.47368439763754289 ) ) ;
#14122=CARTESIAN_POINT ( 'NONE',  ( -15.65588464930769597, 19.60408957237921612, -14.69554073304035668 ) ) ;
#14124=CARTESIAN_POINT ( 'NONE',  ( 14.29363999704249366, -25.05931576210448952, -11.60082902445461706 ) ) ;
#14126=CARTESIAN_POINT ( 'NONE',  ( 13.21981074911866649, 22.21720586980774925, -16.44568224045854166 ) ) ;
#14128=CARTESIAN_POINT ( 'NONE',  ( 11.30648189521336633, 18.04080162384153496, -25.01410076809229110 ) ) ;
#14130=CARTESIAN_POINT ( 'NONE',  ( -14.80676639301200126, 25.71291667989606466, -10.17396840098144750 ) ) ;
#14133=CARTESIAN_POINT ( 'NONE',  ( -13.45451633981421757, -23.63114001665184816, -14.46875807778122081 ) ) ;
#14136=CARTESIAN_POINT ( 'NONE',  ( -32.28394191823594639, -20.85172211888466620, -5.435695248426204884 ) ) ;
#14137=CARTESIAN_POINT ( 'NONE',  ( -6.849675264061505509, -24.72308982460099003, -9.348409214434667547 ) ) ;
#14138=CARTESIAN_POINT ( 'NONE',  ( 13.01345650832474199, 19.67229149937466204, -19.60135455124983395 ) ) ;
#14140=CARTESIAN_POINT ( 'NONE',  ( 19.09486710253168695, 8.055642014369341908, -26.60153427135273674 ) ) ;
#14146=CARTESIAN_POINT ( 'NONE',  ( -20.60443745909306301, -1.795035389764878309, -27.94510193186766145 ) ) ;
#14154=CARTESIAN_POINT ( 'NONE',  ( 30.15216583608805934, -14.28728122224699071, -12.89820425123808256 ) ) ;
#14160=VERTEX_POINT ( 'NONE', #22252 ) ;
#14161=CARTESIAN_POINT ( 'NONE',  ( 0.3248095335732383848, 30.21040829111500869, -15.67845704928061323 ) ) ;
#14168=CARTESIAN_POINT ( 'NONE',  ( 14.00903526708603053, 27.25070609806927280, -10.53950710942262425 ) ) ;
#14172=CARTESIAN_POINT ( 'NONE',  ( -16.80464701721349385, 11.74058409121013469, -30.00000000000000000 ) ) ;
#14174=CARTESIAN_POINT ( 'NONE',  ( -2.485571585149885632, -11.24999999999987566, 6.000000000000000000 ) ) ;
#14175=CARTESIAN_POINT ( 'NONE',  ( 11.21665055246841725, -20.46292137171589332, -20.53731539713322007 ) ) ;
#14176=CYLINDRICAL_SURFACE ( 'NONE', #9413, 15.99999999999999645 ) ;
#14177=CARTESIAN_POINT ( 'NONE',  ( 12.37323903880625764, 20.51431812958072953, -19.49257168437462440 ) ) ;
#14179=CARTESIAN_POINT ( 'NONE',  ( -17.34253826592568970, 27.32041144456614390, -5.000000000000000000 ) ) ;
#14182=CARTESIAN_POINT ( 'NONE',  ( -26.75556982913416704, -25.10111586528267935, -7.156957325213197940 ) ) ;
#14183=CARTESIAN_POINT ( 'NONE',  ( 1.794506358125838696, -24.59416170551979519, -7.919342959519173775 ) ) ;
#14184=CARTESIAN_POINT ( 'NONE',  ( 12.32508505241873031, 19.69439391497782665, -20.57495747500194483 ) ) ;
#14185=CARTESIAN_POINT ( 'NONE',  ( 20.27016213421537572, 13.74473133855453533, -9.391409443377602528 ) ) ;
#14189=CARTESIAN_POINT ( 'NONE',  ( -4.067729689095753720, 20.10162097886301780, -29.23193154362917667 ) ) ;
#14196=CARTESIAN_POINT ( 'NONE',  ( -28.71628164481152368, 0.3103093194282594558, -11.60661526385460718 ) ) ;
#14198=CARTESIAN_POINT ( 'NONE',  ( 20.15225922584352958, -5.429322806097534482, -27.08385357569856922 ) ) ;
#14216=CARTESIAN_POINT ( 'NONE',  ( 18.36481394660784616, 17.66788468870112183, -8.868296049281793714 ) ) ;
#14217=CARTESIAN_POINT ( 'NONE',  ( 11.61237692786606779, 33.10454720036470633, -7.206114420758453321 ) ) ;
#14220=CARTESIAN_POINT ( 'NONE',  ( 10.86866341958027249, -19.47793087445224103, -22.69139715315293770 ) ) ;
#14224=CARTESIAN_POINT ( 'NONE',  ( -11.07085948108040974, 17.50394663469646517, -27.44763187279587413 ) ) ;
#14227=CARTESIAN_POINT ( 'NONE',  ( 13.27451975403652540, -24.88833393671288619, -11.62983193108599700 ) ) ;
#14233=CARTESIAN_POINT ( 'NONE',  ( -7.924297901226319496, 19.68525824574059158, -25.90363148246721181 ) ) ;
#14237=CARTESIAN_POINT ( 'NONE',  ( -34.47791643563932951, -6.499699467164269606, -7.206147143098082353 ) ) ;
#14240=CARTESIAN_POINT ( 'NONE',  ( 23.90523083592902864, 0.5703977246735572049, -19.50614640947865652 ) ) ;
#14247=CARTESIAN_POINT ( 'NONE',  ( -21.27552871334581397, 0.7820719158082399813, -25.01525379879122113 ) ) ;
#14249=ORIENTED_EDGE ( 'NONE', *, *, #12493, .T. ) ;
#14250=CARTESIAN_POINT ( 'NONE',  ( 34.31080765618935402, -5.232520982112594865, -5.452539590646297896 ) ) ;
#14262=DIRECTION ( 'NONE',  ( 0.000000000000000000, 0.000000000000000000, 1.000000000000000000 ) ) ;
#14265=CARTESIAN_POINT ( 'NONE',  ( 5.921814423382286918, 36.05187545745704369, -8.870160957477187580 ) ) ;
#14266=CARTESIAN_POINT ( 'NONE',  ( 18.69487370500359091, 22.45507383323641193, -4.999999999999999112 ) ) ;
#14268=CARTESIAN_POINT ( 'NONE',  ( 18.69514969737914001, -27.26850006250750624, -5.461146079405737375 ) ) ;
#14273=CARTESIAN_POINT ( 'NONE',  ( 10.91553583107620007, 17.35227997941746025, -29.34686799396787649 ) ) ;
#14275=CARTESIAN_POINT ( 'NONE',  ( -12.91493168522746693, 20.67346994317426478, -18.49686148064046876 ) ) ;
#14278=CARTESIAN_POINT ( 'NONE',  ( 11.52208528209529348, 18.40475063778455933, -23.85969712606921078 ) ) ;
#14280=CARTESIAN_POINT ( 'NONE',  ( 32.82868241010613275, -19.42490378352035307, -7.116715984878871915 ) ) ;
#14281=VERTEX_POINT ( 'NONE', #4931 ) ;
#14282=CARTESIAN_POINT ( 'NONE',  ( -10.74681136125822256, 17.71780809595123429, -27.42243502390378396 ) ) ;
#14284=CARTESIAN_POINT ( 'NONE',  ( -14.06110963209943421, -22.53835070925789807, -16.29745831186998117 ) ) ;
#14288=CARTESIAN_POINT ( 'NONE',  ( -19.60397279729912157, -6.775456283739323737, -27.75461981094199260 ) ) ;
#14289=CARTESIAN_POINT ( 'NONE',  ( -14.88818106304697508, -26.46991234739331844, -6.888965760716232012 ) ) ;
#14291=CARTESIAN_POINT ( 'NONE',  ( 17.26836613049929881, 21.08639604684729463, -5.952994375637418401 ) ) ;
#14293=CARTESIAN_POINT ( 'NONE',  ( 23.85642135670279629, 2.961483799603526368, -17.67184769396539323 ) ) ;
#14299=CARTESIAN_POINT ( 'NONE',  ( -29.76338656478942113, -0.1358195184987218418, -10.16612580020036916 ) ) ;
#14300=CARTESIAN_POINT ( 'NONE',  ( 22.40604002092578995, -0.1555999769332679916, -22.63024419021551381 ) ) ;
#14303=CARTESIAN_POINT ( 'NONE',  ( -28.62628535912805461, 0.9249821381284000221, -10.67733050510392268 ) ) ;
#14304=CARTESIAN_POINT ( 'NONE',  ( 11.31392148919590923, 36.91540483778863546, -5.000000000000002665 ) ) ;
#14309=ADVANCED_FACE ( 'NONE', ( #24212, #9178, #23815, #8574 ), #17739, .F. ) ;
#14311=DIRECTION ( 'NONE',  ( 1.000000000000000000, 0.000000000000000000, 0.000000000000000000 ) ) ;
#14314=CARTESIAN_POINT ( 'NONE',  ( -25.53096875586516390, 6.216240356532259703, -5.478322317225678084 ) ) ;
#14317=CARTESIAN_POINT ( 'NONE',  ( 25.19512240098035250, -24.69066459180183415, -9.356458335724495257 ) ) ;
#14321=CARTESIAN_POINT ( 'NONE',  ( 11.36962475154139796, 19.21036919021693024, -22.68052711305023905 ) ) ;
#14324=CARTESIAN_POINT ( 'NONE',  ( -15.64269498361865729, 21.26784539589563394, -12.67544165040647464 ) ) ;
#14326=CARTESIAN_POINT ( 'NONE',  ( 9.564543489041190227, -18.36833051452632048, -27.45183364396559256 ) ) ;
#14327=LINE ( 'NONE', #24073, #15909 ) ;
#14328=CARTESIAN_POINT ( 'NONE',  ( 11.13033197888396764, 17.60926338241307576, -26.83090848175526588 ) ) ;
#14332=CARTESIAN_POINT ( 'NONE',  ( -15.17099104544988641, 26.61370929599295820, -7.820916635083668744 ) ) ;
#14334=CARTESIAN_POINT ( 'NONE',  ( -14.89274031364858786, -25.83765763563116025, -9.708005537497479409 ) ) ;
#14338=CARTESIAN_POINT ( 'NONE',  ( -30.63528468994626053, -19.80586681999809784, -9.728514707820110630 ) ) ;
#14339=CARTESIAN_POINT ( 'NONE',  ( -4.774817478240758639, -20.11729465013693385, -27.10572799927598808 ) ) ;
#14340=CARTESIAN_POINT ( 'NONE',  ( 11.74040845465362892, 16.94500352943240173, -28.11737847864129591 ) ) ;
#14343=CARTESIAN_POINT ( 'NONE',  ( 23.26889270032514645, 6.256968188779593376, -14.81455085170663821 ) ) ;
#14349=CARTESIAN_POINT ( 'NONE',  ( -30.62465793492241062, -2.263991001138987436, -11.41340153498721222 ) ) ;
#14350=CARTESIAN_POINT ( 'NONE',  ( 30.20212831021078870, -0.007183286174248709743, -8.767436680044319530 ) ) ;
#14366=CARTESIAN_POINT ( 'NONE',  ( 0.2333680323409619561, 22.01890222510690975, -24.21865200866544399 ) ) ;
#14373=CARTESIAN_POINT ( 'NONE',  ( 10.48996851602322344, 18.64616631778530120, -24.90364434592935083 ) ) ;
#14376=CARTESIAN_POINT ( 'NONE',  ( -16.98576275542438196, 14.17128621410275180, -20.06049913518808125 ) ) ;
#14380=CARTESIAN_POINT ( 'NONE',  ( 10.56515747574125541, -19.56746311216371481, -22.73119885331434276 ) ) ;
#14382=CARTESIAN_POINT ( 'NONE',  ( 10.98291459920649338, 17.36300444913146634, -28.70599113223154930 ) ) ;
#14383=CARTESIAN_POINT ( 'NONE',  ( 17.34253826539385201, 27.32041144647958575, -13.70816084473008800 ) ) ;
#14386=CARTESIAN_POINT ( 'NONE',  ( -15.65942272168468996, -13.82713998445992054, -27.03602420171817045 ) ) ;
#14387=CARTESIAN_POINT ( 'NONE',  ( 3.914585310762173087, -24.47571531563621861, -9.381846448608621714 ) ) ;
#14388=CARTESIAN_POINT ( 'NONE',  ( 15.50434170514593468, 26.37861656039416047, -5.946155412696958464 ) ) ;
#14390=CARTESIAN_POINT ( 'NONE',  ( 19.21831362878624816, 14.20819548674236543, -12.87518209901260846 ) ) ;
#14394=CARTESIAN_POINT ( 'NONE',  ( -6.368201183702909773, 37.02352246815677717, -6.288982803245489528 ) ) ;
#14402=CARTESIAN_POINT ( 'NONE',  ( -20.51831096985980807, 1.024188904302109737, -28.71274422071960331 ) ) ;
#14404=CARTESIAN_POINT ( 'NONE',  ( 34.80199681878606555, -10.49577831786894677, -8.021756253636395328 ) ) ;
#14416=CARTESIAN_POINT ( 'NONE',  ( 16.36340388119751310, 15.09553078370668366, -20.01599901236055956 ) ) ;
#14417=CARTESIAN_POINT ( 'NONE',  ( 13.11118861972762240, 31.67446990147458052, -5.902404578990857686 ) ) ;
#14422=CARTESIAN_POINT ( 'NONE',  ( 15.47930552936342963, -26.10041863403043649, -9.214347334491035824 ) ) ;
#14425=CARTESIAN_POINT ( 'NONE',  ( -15.41023552481722447, 26.80405844223972522, -5.474109759163972910 ) ) ;
#14427=CARTESIAN_POINT ( 'NONE',  ( 10.09725523659168722, -20.16347431786755706, -21.70548052805963835 ) ) ;
#14431=CARTESIAN_POINT ( 'NONE',  ( -10.34192303438924299, 26.07364305517009839, -16.01722023157933705 ) ) ;
#14437=CARTESIAN_POINT ( 'NONE',  ( 20.96446129645448408, 0.8575792327581100993, -26.22921226360291769 ) ) ;
#14443=CARTESIAN_POINT ( 'NONE',  ( -28.32157472073443216, 0.1617651296188915844, -12.55129266915809261 ) ) ;
#14446=CARTESIAN_POINT ( 'NONE',  ( 30.24971233770529011, -4.493041484851756806, -13.15307322356999897 ) ) ;
#14461=CARTESIAN_POINT ( 'NONE',  ( 7.119170425228222854, 36.77535074466948117, -5.866140454657438497 ) ) ;
#14464=EDGE_CURVE ( 'NONE', #15130, #25273, #36284, .T. ) ;
#14467=CARTESIAN_POINT ( 'NONE',  ( 17.86116285895126410, -24.79026673224041843, -12.29608082019653459 ) ) ;
#14473=CARTESIAN_POINT ( 'NONE',  ( 14.23710703006283396, 24.61411403652301644, -12.53843163329819532 ) ) ;
#14475=CARTESIAN_POINT ( 'NONE',  ( -15.51364032778053925, 26.43312886238355119, -5.474109364757008045 ) ) ;
#14478=CARTESIAN_POINT ( 'NONE',  ( 14.88668315484156146, 25.46919082029659620, -10.18295691443133499 ) ) ;
#14480=CARTESIAN_POINT ( 'NONE',  ( 21.74907656359282626, -13.77287494480177976, -19.63093583157703748 ) ) ;
#14482=CARTESIAN_POINT ( 'NONE',  ( -10.79408003525095694, 18.03183192774827859, -26.18276724716969639 ) ) ;
#14484=CARTESIAN_POINT ( 'NONE',  ( -10.48684353440000194, -17.61503585894356050, -29.32750364307806734 ) ) ;
#14486=CIRCLE ( 'NONE', #19040, 16.00000000000000355 ) ;
#14488=CARTESIAN_POINT ( 'NONE',  ( -35.13470064561631290, -12.09547139906384672, -7.143865450880896972 ) ) ;
#14489=CARTESIAN_POINT ( 'NONE',  ( -14.35490488552378174, -25.85456304999896560, -9.246097774239588674 ) ) ;
#14492=CARTESIAN_POINT ( 'NONE',  ( 28.61305316926027587, 1.166352659189931140, -10.20691745326966604 ) ) ;
#14497=ORIENTED_EDGE ( 'NONE', *, *, #27152, .F. ) ;
#14498=CARTESIAN_POINT ( 'NONE',  ( -27.21489488970257753, 0.1324291793181980870, -14.46509639632424360 ) ) ;
#14499=CARTESIAN_POINT ( 'NONE',  ( 22.96275717310609110, -0.2160451777520107086, -21.50653127259290898 ) ) ;
#14503=CARTESIAN_POINT ( 'NONE',  ( -23.97679352225928184, 2.727602047639537730, -17.65530553011062054 ) ) ;
#14507=CIRCLE ( 'NONE', #17778, 17.00000000000000355 ) ;
#14513=LINE ( 'NONE', #12063, #6821 ) ;
#14515=CARTESIAN_POINT ( 'NONE',  ( -20.09296739951089350, 5.008361712747955607, -27.07435144307553898 ) ) ;
#14518=CARTESIAN_POINT ( 'NONE',  ( 15.05365685536567355, -14.74619886204681585, -26.38815432015796958 ) ) ;
#14519=LINE ( 'NONE', #7818, #6678 ) ;
#14521=CARTESIAN_POINT ( 'NONE',  ( 15.01939689310542825, 26.78336088948045557, -8.278624996432389693 ) ) ;
#14526=CARTESIAN_POINT ( 'NONE',  ( -16.10992647123930510, 22.10140223917236213, -10.24986995600674078 ) ) ;
#14529=CARTESIAN_POINT ( 'NONE',  ( 15.43121851897235786, 26.72868093004962020, -5.474190317923420146 ) ) ;
#14533=CARTESIAN_POINT ( 'NONE',  ( -10.99222416622049359, 17.55659943774363185, -27.44150676154917790 ) ) ;
#14535=CARTESIAN_POINT ( 'NONE',  ( -14.83405348788300415, -25.67306116219898726, -10.17574755994341373 ) ) ;
#14537=CARTESIAN_POINT ( 'NONE',  ( -33.53737908833902992, -18.88502799929946008, -5.855487158225816557 ) ) ;
#14539=CARTESIAN_POINT ( 'NONE',  ( -11.57545763705510744, -25.81734924782649543, -5.474310789163009616 ) ) ;
#14541=CARTESIAN_POINT ( 'NONE',  ( 15.84467149865224833, 25.30824157118464868, -5.000000000000000888 ) ) ;
#14543=CARTESIAN_POINT ( 'NONE',  ( 23.06768432047073247, 7.142456518765742501, -13.83685962162048710 ) ) ;
#14548=ORIENTED_EDGE ( 'NONE', *, *, #21732, .T. ) ;
#14549=CARTESIAN_POINT ( 'NONE',  ( -30.56639149896655638, -1.107291129257161444, -10.09863760926522325 ) ) ;
#14551=CARTESIAN_POINT ( 'NONE',  ( 30.94782199696930647, -0.1917222966042023691, -6.413581524601221773 ) ) ;
#14552=FACE_OUTER_BOUND ( 'NONE', #7692, .T. ) ;
#14567=CARTESIAN_POINT ( 'NONE',  ( -0.3972110264143906000, 20.50537081352338475, -30.00000000000000355 ) ) ;
#14576=CARTESIAN_POINT ( 'NONE',  ( 14.21588428194489673, 27.70830296778597557, -9.610143119930103950 ) ) ;
#14580=CARTESIAN_POINT ( 'NONE',  ( -17.46026703879977049, 13.44560834044810704, -20.08683738022571319 ) ) ;
#14581=DIRECTION ( 'NONE',  ( -0.000000000000000000, -0.000000000000000000, 1.000000000000000000 ) ) ;
#14583=CARTESIAN_POINT ( 'NONE',  ( 14.08258714517840637, -24.61786426002636929, -12.54774028598870395 ) ) ;
#14585=CARTESIAN_POINT ( 'NONE',  ( 12.91504324178902152, 21.67529910927544634, -17.43456327316026844 ) ) ;
#14586=CIRCLE ( 'NONE', #4860, 18.00000000000000000 ) ;
#14590=CARTESIAN_POINT ( 'NONE',  ( -16.24747610076109439, -13.49626370421807309, -26.31547060377475944 ) ) ;
#14591=CARTESIAN_POINT ( 'NONE',  ( 4.290221133370377693, -20.29569990938377089, -26.55723615674921945 ) ) ;
#14592=CARTESIAN_POINT ( 'NONE',  ( 15.52046154931812261, 26.41174381453696540, -5.474116501232952459 ) ) ;
#14593=CARTESIAN_POINT ( 'NONE',  ( 20.29313191480849099, 11.31791106737759556, -14.92333789774876607 ) ) ;
#14596=CARTESIAN_POINT ( 'NONE',  ( -4.675295383163502017, 19.96902330696676131, -29.23835142064850956 ) ) ;
#14605=CARTESIAN_POINT ( 'NONE',  ( -27.59216913682209338, 0.3852774775313504430, -13.52450996651226411 ) ) ;
#14607=CARTESIAN_POINT ( 'NONE',  ( 35.47189031372824530, -10.73249152999393097, -5.870541421840872687 ) ) ;
#14615=AXIS2_PLACEMENT_3D ( 'NONE', #24954, #12956, #4008 ) ;
#14623=CARTESIAN_POINT ( 'NONE',  ( 18.57748288431603712, 16.38268946942090309, -10.84922581770859296 ) ) ;
#14624=CARTESIAN_POINT ( 'NONE',  ( 10.11190604682229299, 28.56348632143605926, -14.02879073800986909 ) ) ;
#14627=CARTESIAN_POINT ( 'NONE',  ( -19.38332915818774893, 8.712623186017649957, -23.31311828547350018 ) ) ;
#14630=CARTESIAN_POINT ( 'NONE',  ( 12.09766887496989085, -21.47150019090766548, -18.42868602394403155 ) ) ;
#14633=CARTESIAN_POINT ( 'NONE',  ( -11.29646106035690245, 18.04863004157237327, -25.01271745524739387 ) ) ;
#14634=CARTESIAN_POINT ( 'NONE',  ( 10.63490610281069770, -21.58777382264839062, -18.57263060209788108 ) ) ;
#14638=CARTESIAN_POINT ( 'NONE',  ( -11.86532622451750107, 33.05761182678129728, -6.331822098149086919 ) ) ;
#14646=EDGE_LOOP ( 'NONE', ( #11814, #243, #34942, #27549 ) ) ;
#14647=CARTESIAN_POINT ( 'NONE',  ( 29.51458379201200088, 0.1415349160452132049, -10.18257699856247278 ) ) ;
#14652=CARTESIAN_POINT ( 'NONE',  ( -20.81523479917187203, 0.8345188516400835477, -26.83090836434666215 ) ) ;
#14655=CARTESIAN_POINT ( 'NONE',  ( 29.45872667429271630, -4.364009981319033393, -14.09197514256877426 ) ) ;
#14660=CARTESIAN_POINT ( 'NONE',  ( -37.49625565938783467, -14.69322820095469240, -5.000000000000008882 ) ) ;
#14665=CARTESIAN_POINT ( 'NONE',  ( -13.29616015536805662, -18.15165799370312882, -30.00000000000000711 ) ) ;
#14667=AXIS2_PLACEMENT_3D ( 'NONE', #4532, #33183, #4939 ) ;
#14669=CARTESIAN_POINT ( 'NONE',  ( 3.426279686912360400, 21.12864742734303292, -25.63660972253196846 ) ) ;
#14674=CARTESIAN_POINT ( 'NONE',  ( 15.97914833959363357, -22.30600193650763785, -16.12660968148156471 ) ) ;
#14677=DIRECTION ( 'NONE',  ( -0.000000000000000000, 0.000000000000000000, -1.000000000000000000 ) ) ;
#14678=ORIENTED_EDGE ( 'NONE', *, *, #35669, .T. ) ;
#14679=CARTESIAN_POINT ( 'NONE',  ( 12.59997131692024297, 21.13310654933077259, -18.44044215902303563 ) ) ;
#14681=CARTESIAN_POINT ( 'NONE',  ( -13.30230047454564968, 21.05347397263300380, -17.49821043808168852 ) ) ;
#14684=CARTESIAN_POINT ( 'NONE',  ( 12.45581562386595031, 20.40522463409936904, -19.50774782679574670 ) ) ;
#14686=CARTESIAN_POINT ( 'NONE',  ( 32.01702270572438636, -20.29116740411223319, -7.545109314425605618 ) ) ;
#14688=CARTESIAN_POINT ( 'NONE',  ( -12.63529647066861905, 22.12582800369916924, -17.37362551299798596 ) ) ;
#14690=CARTESIAN_POINT ( 'NONE',  ( -17.87207185564084355, -26.59298717711743976, -8.659308747257311367 ) ) ;
#14693=CARTESIAN_POINT ( 'NONE',  ( -19.74937082396974120, -7.498879515469185186, -26.30929424058608035 ) ) ;
#14694=CARTESIAN_POINT ( 'NONE',  ( -14.68167628062920826, -25.79242183381518316, -9.711880916258452956 ) ) ;
#14697=CARTESIAN_POINT ( 'NONE',  ( 25.33785701000014612, 2.122015632169762078, -15.59009891290605943 ) ) ;
#14703=CARTESIAN_POINT ( 'NONE',  ( -27.81571540047708879, 0.08885976736978917767, -13.50292438661861638 ) ) ;
#14705=CARTESIAN_POINT ( 'NONE',  ( 25.65762806520498529, -0.4781389605788837205, -17.32945229485775229 ) ) ;
#14706=CIRCLE ( 'NONE', #19892, 17.00000000000000000 ) ;
#14710=CARTESIAN_POINT ( 'NONE',  ( -26.91927498037264499, 4.412534205184938330, -5.476192048854705341 ) ) ;
#14719=CARTESIAN_POINT ( 'NONE',  ( -25.95420856792063447, 5.296653683992947670, -7.877654426414621547 ) ) ;
#14723=CARTESIAN_POINT ( 'NONE',  ( 22.30282066329013446, -21.88865312665271290, -13.92261583855099438 ) ) ;
#14726=CARTESIAN_POINT ( 'NONE',  ( 10.65067361986881700, 17.57180219728759241, -28.69216590317797611 ) ) ;
#14729=CARTESIAN_POINT ( 'NONE',  ( -13.37529537539570867, 15.55228444284129097, -29.39288029773726052 ) ) ;
#14733=CARTESIAN_POINT ( 'NONE',  ( 12.15072974113908089, 19.90049516934647045, -20.54455445324533258 ) ) ;
#14736=EDGE_LOOP ( 'NONE', ( #17909, #1763, #36937, #16322 ) ) ;
#14737=CARTESIAN_POINT ( 'NONE',  ( -14.48563613516329873, 25.10382544214007083, -11.58903774489672500 ) ) ;
#14739=CARTESIAN_POINT ( 'NONE',  ( -11.60472954253665456, -20.96974312390484130, -19.48931687713154304 ) ) ;
#14742=CARTESIAN_POINT ( 'NONE',  ( -28.30349747650313930, -15.93428203292501522, -13.80390666543416955 ) ) ;
#14743=CARTESIAN_POINT ( 'NONE',  ( -9.169147237707843345, -25.20086482100098024, -7.872094350184594802 ) ) ;
#14745=CARTESIAN_POINT ( 'NONE',  ( 12.74585289761866136, 17.86932441180232090, -22.89739794729497646 ) ) ;
#14747=CARTESIAN_POINT ( 'NONE',  ( 23.92111322297680687, 6.328116427676794054, -12.80316392715411133 ) ) ;
#14753=CARTESIAN_POINT ( 'NONE',  ( -20.88471566866979146, -0.5118096901872604132, -26.72609791841199822 ) ) ;
#14754=CARTESIAN_POINT ( 'NONE',  ( 31.05798941631825727, -0.2002603227334578129, -5.473151826744909521 ) ) ;
#14759=CARTESIAN_POINT ( 'NONE',  ( 22.45323650136968396, -2.382502413133517738, -29.99999999999998934 ) ) ;
#14769=CARTESIAN_POINT ( 'NONE',  ( 0.3500065460287011265, 32.44603839567150061, -13.80550477351713390 ) ) ;
#14778=CARTESIAN_POINT ( 'NONE',  ( 14.70740557672079518, 28.82247346305062408, -5.465036479938481406 ) ) ;
#14781=CARTESIAN_POINT ( 'NONE',  ( -16.44708297367234451, 13.55940066003513955, -23.27598954255405417 ) ) ;
#14784=CARTESIAN_POINT ( 'NONE',  ( 9.495448100151719473, -18.16828483302926145, -30.00000000000000000 ) ) ;
#14785=CARTESIAN_POINT ( 'NONE',  ( 14.28858787313285994, 24.47746469342009235, -12.55008231428945997 ) ) ;
#14786=CARTESIAN_POINT ( 'NONE',  ( 11.67120187369582851, 18.92585590138232732, -22.73257522065779668 ) ) ;
#14791=CARTESIAN_POINT ( 'NONE',  ( -17.48025379037459714, -14.52550820055553160, -23.07137230154036800 ) ) ;
#14792=CARTESIAN_POINT ( 'NONE',  ( 4.646166367048098600, -21.13261100285546945, -22.14179161734661605 ) ) ;
#14793=CARTESIAN_POINT ( 'NONE',  ( 15.07117766819621885, 24.92558405637350560, -10.19323716522371726 ) ) ;
#14794=CARTESIAN_POINT ( 'NONE',  ( 19.35936484833087690, 11.87520330856569650, -16.98394864372990654 ) ) ;
#14796=CARTESIAN_POINT ( 'NONE',  ( -4.200723223758354052, 37.83089482203977383, -6.281056964556750444 ) ) ;
#14798=ORIENTED_EDGE ( 'NONE', *, *, #11042, .F. ) ;
#14805=CARTESIAN_POINT ( 'NONE',  ( -30.65045886600562852, 0.1824153768363431516, -5.946136105496247382 ) ) ;
#14806=CARTESIAN_POINT ( 'NONE',  ( 22.47955544282887530, -6.794619135805436194, -22.00045867376432795 ) ) ;
#14817=CYLINDRICAL_SURFACE ( 'NONE', #23044, 17.00000000000000000 ) ;
#14821=CARTESIAN_POINT ( 'NONE',  ( 18.98065206215026990, -15.49966443493606327, -20.77364446795738218 ) ) ;
#14823=CARTESIAN_POINT ( 'NONE',  ( 19.37072484188776400, 15.75976958111966297, -8.396351507073255505 ) ) ;
#14825=CARTESIAN_POINT ( 'NONE',  ( 7.999721452599430016, 22.53002257771371220, -21.05289303791193234 ) ) ;
#14827=CARTESIAN_POINT ( 'NONE',  ( -22.33890996451869171, 10.80501728358744984, -6.452941623317727249 ) ) ;
#14830=CARTESIAN_POINT ( 'NONE',  ( 15.58441477488922366, -26.56835683918586710, -7.350884426725713183 ) ) ;
#14833=CARTESIAN_POINT ( 'NONE',  ( -11.09393661379458074, 17.63453714546405848, -26.82748596485767933 ) ) ;
#14834=CARTESIAN_POINT ( 'NONE',  ( -23.72113249276927505, -26.46856040302326463, -6.759642254155505903 ) ) ;
#14835=CARTESIAN_POINT ( 'NONE',  ( 12.99674836092793839, -24.46215500157558864, -12.58877913748062127 ) ) ;
#14839=CARTESIAN_POINT ( 'NONE',  ( -9.393194761908011614, 23.60535835710769703, -19.02674971333937037 ) ) ;
#14841=EDGE_CURVE ( 'NONE', #29462, #3976, #36719, .T. ) ;
#14846=CARTESIAN_POINT ( 'NONE',  ( 29.93839244934208921, 0.08748910287391382934, -9.239377091290068122 ) ) ;
#14852=CARTESIAN_POINT ( 'NONE',  ( -30.76822878952619433, -0.006411674588949102180, -6.417027793339856068 ) ) ;
#14855=CARTESIAN_POINT ( 'NONE',  ( 20.30048362414427743, -2.857582090605152558, -29.99999999999998579 ) ) ;
#14870=CARTESIAN_POINT ( 'NONE',  ( 3.279674764711695722, 20.24540435116753301, -29.22490024661859920 ) ) ;
#14874=CARTESIAN_POINT ( 'NONE',  ( 13.35105216789999716, -17.76889701558443591, -23.46262091258972049 ) ) ;
#14880=CARTESIAN_POINT ( 'NONE',  ( 12.35228433879287380, 20.54234309038960049, -19.48813501896534817 ) ) ;
#14882=CARTESIAN_POINT ( 'NONE',  ( -11.45248459189543588, 17.05290680873532239, -28.72504823342588409 ) ) ;
#14885=CARTESIAN_POINT ( 'NONE',  ( 13.00369382996352563, 21.53152199447597326, -17.45016979600528018 ) ) ;
#14886=ORIENTED_EDGE ( 'NONE', *, *, #3441, .T. ) ;
#14887=CARTESIAN_POINT ( 'NONE',  ( 18.96300721855776317, -11.21761247941028650, -24.21598040740967406 ) ) ;
#14889=CARTESIAN_POINT ( 'NONE',  ( -10.67640217097355482, 17.76288147141041662, -27.41698759738607194 ) ) ;
#14891=CARTESIAN_POINT ( 'NONE',  ( -17.17635872890215509, -26.93998231148862743, -6.852558094669841893 ) ) ;
#14895=CARTESIAN_POINT ( 'NONE',  ( -35.43763548776691863, -11.07137260576668147, -5.869669228994635723 ) ) ;
#14896=CARTESIAN_POINT ( 'NONE',  ( -9.345945910616261898, -18.29489296895642880, -28.71376903915567880 ) ) ;
#14899=CARTESIAN_POINT ( 'NONE',  ( 29.75447456610766750, 1.108193808558314508, -5.946487029707098415 ) ) ;
#14903=ORIENTED_EDGE ( 'NONE', *, *, #38076, .T. ) ;
#14904=CARTESIAN_POINT ( 'NONE',  ( -21.72248880293610185, 0.6579594075278962784, -23.84550374915839654 ) ) ;
#14906=CARTESIAN_POINT ( 'NONE',  ( 31.51816681948337617, -1.356210769490176160, -8.235438873524525860 ) ) ;
#14910=CARTESIAN_POINT ( 'NONE',  ( -26.55795656307421027, 3.516599515638362927, -10.75008132255575433 ) ) ;
#14912=DIRECTION ( 'NONE',  ( -0.000000000000000000, -0.000000000000000000, -1.000000000000000000 ) ) ;
#14919=CARTESIAN_POINT ( 'NONE',  ( -23.41974574084031246, 6.012251731081178718, -14.80241686762865605 ) ) ;
#14922=CARTESIAN_POINT ( 'NONE',  ( 25.29206606878849328, -26.20377346906149185, -5.444282035157826272 ) ) ;
#14925=CARTESIAN_POINT ( 'NONE',  ( 15.05907480041244639, 26.65905605469517781, -8.283340056487517700 ) ) ;
#14929=CARTESIAN_POINT ( 'NONE',  ( -15.20187259911379662, 18.82279879278276269, -16.71752878418681476 ) ) ;
#14932=CARTESIAN_POINT ( 'NONE',  ( 11.70759707017889362, 18.89087562079335569, -22.73869321768459173 ) ) ;
#14937=CARTESIAN_POINT ( 'NONE',  ( -15.33869540756803751, 26.96259011824205487, -5.943855708106864810 ) ) ;
#14939=CARTESIAN_POINT ( 'NONE',  ( -9.506566060136700358, -18.16246691004805314, -29.34816978379683050 ) ) ;
#14941=CARTESIAN_POINT ( 'NONE',  ( -33.15301329781156170, -17.35959640044362473, -8.406341442035538236 ) ) ;
#14942=CARTESIAN_POINT ( 'NONE',  ( -10.12595346383139017, -23.38316831488110026, -14.65118248118756306 ) ) ;
#14944=CARTESIAN_POINT ( 'NONE',  ( 12.67361812497431295, 18.54269888232404995, -21.74640883014503245 ) ) ;
#14946=CARTESIAN_POINT ( 'NONE',  ( 20.30257773999915116, 5.964623025713435389, -24.29955355791028992 ) ) ;
#14949=CARTESIAN_POINT ( 'NONE',  ( 0.000000000000000000, 22.50000000000000355, 6.000000000000000000 ) ) ;
#14951=CARTESIAN_POINT ( 'NONE',  ( -30.48098785803534483, -0.7257077854517125504, -9.657254528547552397 ) ) ;
#14952=CARTESIAN_POINT ( 'NONE',  ( 30.87575086445591666, -0.1861898454035852968, -6.883314186587743855 ) ) ;
#14956=CARTESIAN_POINT ( 'NONE',  ( 37.62663912510992503, -8.659558992827971480, -14.26382729546509687 ) ) ;
#14963=CARTESIAN_POINT ( 'NONE',  ( 2.741814962476898376, 38.30556977738701363, -5.435872072964093249 ) ) ;
#14971=CARTESIAN_POINT ( 'NONE',  ( 14.85673200164996643, 28.20965467857394771, -6.393760900654135604 ) ) ;
#14975=CARTESIAN_POINT ( 'NONE',  ( -15.91172688669051283, 12.94523012445180399, -30.00000000000000711 ) ) ;
#14980=CARTESIAN_POINT ( 'NONE',  ( 9.531353544348123208, -18.20021061595370782, -28.70654323991336909 ) ) ;
#14983=CARTESIAN_POINT ( 'NONE',  ( 12.63673072935002573, 21.07828628784659131, -18.44856727879870206 ) ) ;
#14987=CARTESIAN_POINT ( 'NONE',  ( -22.68080910437082309, -17.76831930014195393, -16.67414630805707887 ) ) ;
#14988=CARTESIAN_POINT ( 'NONE',  ( 1.539264792407522231, -22.70516402096868092, -16.98615508874380353 ) ) ;
#14989=CARTESIAN_POINT ( 'NONE',  ( 11.39136839498931408, 17.60508876921546317, -26.24673842913259136 ) ) ;
#14990=CARTESIAN_POINT ( 'NONE',  ( 17.89753197511066674, 10.02670602479014228, -29.42980511128735444 ) ) ;
#14992=CARTESIAN_POINT ( 'NONE',  ( -2.883099083560371589, 20.54810638744049811, -27.73126374019785345 ) ) ;
#14994=CARTESIAN_POINT ( 'NONE',  ( -33.67692147928062241, -6.312519796522384041, -8.978852421033355569 ) ) ;
#15001=CARTESIAN_POINT ( 'NONE',  ( -22.17658030202064978, 0.8441110128694983006, -22.75671850330635237 ) ) ;
#15002=CARTESIAN_POINT ( 'NONE',  ( 19.45830134839955505, -7.192962728667438022, -27.74412373246262220 ) ) ;
#15003=AXIS2_PLACEMENT_3D ( 'NONE', #5121, #14262, #4518 ) ;
#15008=FACE_OUTER_BOUND ( 'NONE', #3741, .T. ) ;
#15016=CARTESIAN_POINT ( 'NONE',  ( 30.18422347142476880, -23.20414393450525736, -5.437200421920011628 ) ) ;
#15017=CARTESIAN_POINT ( 'NONE',  ( 18.14119866732840336, 14.50330093467433556, -15.90978874977256829 ) ) ;
#15018=CARTESIAN_POINT ( 'NONE',  ( 7.898168204405470405, 20.17838150051020207, -24.60177268676963536 ) ) ;
#15020=CARTESIAN_POINT ( 'NONE',  ( -21.87593696763935824, 10.61463320033040247, -10.38310781559205687 ) ) ;
#15023=CARTESIAN_POINT ( 'NONE',  ( 14.74460831617895806, -25.48601742449350738, -10.64559727961380631 ) ) ;
#15025=CARTESIAN_POINT ( 'NONE',  ( 30.41237130417911771, 3.314011747244134387, -4.999999999999999112 ) ) ;
#15026=CARTESIAN_POINT ( 'NONE',  ( -11.27968654789714797, 18.06170250143723877, -25.01040361136536561 ) ) ;
#15028=CARTESIAN_POINT ( 'NONE',  ( -22.66017947715816661, -25.37253451465284115, -9.858107741291926018 ) ) ;
#15029=CARTESIAN_POINT ( 'NONE',  ( 10.61360125799510179, -25.41145544430514747, -7.858495472244451996 ) ) ;
#15034=CARTESIAN_POINT ( 'NONE',  ( -11.15150138062039709, 34.02824952835918992, -5.000000000000002665 ) ) ;
#15038=ORIENTED_EDGE ( 'NONE', *, *, #31617, .T. ) ;
#15039=CARTESIAN_POINT ( 'NONE',  ( 28.88427010664839045, 0.1085951546874318191, -11.59929086114978247 ) ) ;
#15045=CARTESIAN_POINT ( 'NONE',  ( -29.98580443888884162, 0.03576373324625783945, -9.238541745588479515 ) ) ;
#15048=CARTESIAN_POINT ( 'NONE',  ( 33.79624156833973103, -5.123317329496374306, -7.674098321924684107 ) ) ;
#15053=CARTESIAN_POINT ( 'NONE',  ( -20.71630303010418572, -29.20803740758281464, -4.999999999999997335 ) ) ;
#15061=ADVANCED_FACE ( 'NONE', ( #8938 ), #28493, .T. ) ;
#15062=CARTESIAN_POINT ( 'NONE',  ( 3.904167649330699152, 20.20748209445285681, -28.48006849494148796 ) ) ;
#15067=CARTESIAN_POINT ( 'NONE',  ( 10.80806213842329200, -17.72408045989398673, -27.36067723112840255 ) ) ;
#15073=CARTESIAN_POINT ( 'NONE',  ( -11.01126394183691737, 17.29167595606526575, -29.99999999999999645 ) ) ;
#15077=CARTESIAN_POINT ( 'NONE',  ( 10.18847001889738557, -19.17713045604790167, -23.85841820396901269 ) ) ;
#15081=CARTESIAN_POINT ( 'NONE',  ( -14.09379978727693050, 28.77806074224476163, -8.659515015975241425 ) ) ;
#15083=CARTESIAN_POINT ( 'NONE',  ( -16.21692691291975663, -23.02287499300812357, -15.16141334603994473 ) ) ;
#15084=CARTESIAN_POINT ( 'NONE',  ( -17.34253826592568970, 27.32041144456614390, -5.000000000000000000 ) ) ;
#15086=CARTESIAN_POINT ( 'NONE',  ( -33.27136418661606854, -12.54424548814919937, -10.20349738210835078 ) ) ;
#15087=CARTESIAN_POINT ( 'NONE',  ( -14.43538540834600603, -25.42431206739405525, -10.65726991915511768 ) ) ;
#15091=CARTESIAN_POINT ( 'NONE',  ( 21.37456834929076166, 2.344506045348980994, -24.03039016388560256 ) ) ;
#15097=CARTESIAN_POINT ( 'NONE',  ( -25.90181000411780943, 0.2561891300705002594, -16.43557158720686573 ) ) ;
#15100=CARTESIAN_POINT ( 'NONE',  ( 26.25999556400573098, -0.3564369614627482807, -16.35972333294595060 ) ) ;
#15105=CARTESIAN_POINT ( 'NONE',  ( -27.56582635568890183, 2.642126925834923146, -9.763091250748670902 ) ) ;
#15113=EDGE_CURVE ( 'NONE', #29585, #34227, #26471, .T. ) ;
#15116=CARTESIAN_POINT ( 'NONE',  ( -20.87835934725191933, 7.397986125119080825, -20.05141113204322423 ) ) ;
#15119=CARTESIAN_POINT ( 'NONE',  ( 25.18615822904968837, -26.10665374189652255, -6.311177740306681549 ) ) ;
#15121=CARTESIAN_POINT ( 'NONE',  ( 12.80245792270091343, 21.86072822920704439, -17.40930403903157853 ) ) ;
#15123=ORIENTED_EDGE ( 'NONE', *, *, #24599, .T. ) ;
#15124=CARTESIAN_POINT ( 'NONE',  ( -13.52125812691403084, 19.79767817946104813, -18.59499618884840189 ) ) ;
#15128=CARTESIAN_POINT ( 'NONE',  ( 13.22685551685943750, 22.20468417799810368, -16.44677199118808630 ) ) ;
#15130=VERTEX_POINT ( 'NONE', #36325 ) ;
#15131=DIRECTION ( 'NONE',  ( -1.000000000000000000, 0.000000000000000000, 0.000000000000000000 ) ) ;
#15133=CARTESIAN_POINT ( 'NONE',  ( -14.22044113856730085, 24.65775004622394562, -12.53473158459295433 ) ) ;
#15134=DIRECTION ( 'NONE',  ( 1.000000000000000000, 0.000000000000000000, 0.000000000000000000 ) ) ;
#15135=CARTESIAN_POINT ( 'NONE',  ( -13.90384679662962064, -24.14306550353441239, -13.49653236846003601 ) ) ;
#15138=CARTESIAN_POINT ( 'NONE',  ( -18.43138823906292245, -10.38250042718520838, -26.25437023946332360 ) ) ;
#15139=CARTESIAN_POINT ( 'NONE',  ( -11.13925371099489858, -22.06373630501061811, -17.53492604603244231 ) ) ;
#15141=CARTESIAN_POINT ( 'NONE',  ( 13.15222192828749748, 18.70752044091742761, -20.71114827470474040 ) ) ;
#15143=CARTESIAN_POINT ( 'NONE',  ( 24.64205719296993280, 7.386444343913908028, -5.960736307629980857 ) ) ;
#15145=DIRECTION ( 'NONE',  ( -0.000000000000000000, -0.000000000000000000, -1.000000000000000000 ) ) ;
#15148=CARTESIAN_POINT ( 'NONE',  ( -31.78846064705475527, -1.224209755121473675, -6.856355146768160047 ) ) ;
#15150=CARTESIAN_POINT ( 'NONE',  ( 22.77334587319110071, 0.4700357585246903724, -21.59816853818721327 ) ) ;
#15157=ORIENTED_EDGE ( 'NONE', *, *, #8197, .T. ) ;
#15163=CARTESIAN_POINT ( 'NONE',  ( 3.179194328277191506, 30.99994159145660078, -14.75100848146118970 ) ) ;
#15170=CARTESIAN_POINT ( 'NONE',  ( 10.81914528518449892, 18.98893231873664078, -23.75032747527389887 ) ) ;
#15173=CARTESIAN_POINT ( 'NONE',  ( -17.26255069659608310, 13.24883950376971598, -21.14449336137800373 ) ) ;
#15177=CARTESIAN_POINT ( 'NONE',  ( 14.73715625254732231, -25.65210853834342686, -10.18073480337578829 ) ) ;
#15178=CARTESIAN_POINT ( 'NONE',  ( -21.42170977900226703, -25.44073649801487491, -10.34015057612328370 ) ) ;
#15180=CARTESIAN_POINT ( 'NONE',  ( 11.66727136869983283, 18.92964083422280552, -22.73188705715889313 ) ) ;
#15186=CARTESIAN_POINT ( 'NONE',  ( -27.78070527026259740, -23.17491891568929674, -9.313639814683513762 ) ) ;
#15187=CARTESIAN_POINT ( 'NONE',  ( 1.264170519848298424, -20.71387444820763335, -26.62396510143870287 ) ) ;
#15188=CARTESIAN_POINT ( 'NONE',  ( 15.62693799746092971, 26.04132429419060557, -4.999999999999999112 ) ) ;
#15189=CARTESIAN_POINT ( 'NONE',  ( 20.92218733704004663, 11.65753682693518911, -11.88398976070928015 ) ) ;
#15190=PRODUCT_DEFINITION_FORMATION_WITH_SPECIFIED_SOURCE ( 'ANY', '', #7087, .NOT_KNOWN. ) ;
#15192=CARTESIAN_POINT ( 'NONE',  ( -5.321426344574297751, 37.58193452263969903, -5.861036830693866051 ) ) ;
#15194=CARTESIAN_POINT ( 'NONE',  ( -31.89401778038308777, -5.009461060679962330, -11.27517601632434996 ) ) ;
#15198=DIRECTION ( 'NONE',  ( 0.000000000000000000, 0.000000000000000000, 1.000000000000000000 ) ) ;
#15201=CARTESIAN_POINT ( 'NONE',  ( -29.03964460488705868, 0.9025844493971224569, -9.726429368847238521 ) ) ;
#15202=CARTESIAN_POINT ( 'NONE',  ( 35.25372542428971201, -14.20602460021386193, -4.999999999999997335 ) ) ;
#15214=ORIENTED_EDGE ( 'NONE', *, *, #28400, .F. ) ;
#15215=CARTESIAN_POINT ( 'NONE',  ( -2.236895112781585482, 20.38702974553298830, -29.99999999999999289 ) ) ;
#15219=CARTESIAN_POINT ( 'NONE',  ( 16.34286479496965327, -12.53075802742931266, -28.46040907605739534 ) ) ;
#15220=CARTESIAN_POINT ( 'NONE',  ( 16.27893284296826337, 12.57309314609360129, -28.28617463803444210 ) ) ;
#15221=CARTESIAN_POINT ( 'NONE',  ( 10.45177150771196040, 27.06930753712435589, -15.02913264056041243 ) ) ;
#15222=CIRCLE ( 'NONE', #20416, 21.00000000000002842 ) ;
#15224=CARTESIAN_POINT ( 'NONE',  ( -21.61538879608044894, 11.66913484622351938, -8.407920237374057137 ) ) ;
#15226=CARTESIAN_POINT ( 'NONE',  ( 14.80517497283435979, -25.49818430814198322, -10.64180685166133600 ) ) ;
#15228=CARTESIAN_POINT ( 'NONE',  ( 21.88444403592371756, 6.126538576424477966, -30.00000000000001066 ) ) ;
#15229=CARTESIAN_POINT ( 'NONE',  ( -12.37885040140798765, 20.50679986589284098, -19.49376219608895866 ) ) ;
#15230=CARTESIAN_POINT ( 'NONE',  ( -17.04124340972882834, -20.30949825123198949, -17.92891331059860249 ) ) ;
#15231=CARTESIAN_POINT ( 'NONE',  ( 10.05098765505323222, -24.42915519467451091, -11.72241341964282491 ) ) ;
#15235=CARTESIAN_POINT ( 'NONE',  ( -6.485893174894165725, 19.45725460019876252, -29.26213642569760864 ) ) ;
#15241=CARTESIAN_POINT ( 'NONE',  ( 20.96888093453203794, 0.8149526723977724707, -26.22550878230689619 ) ) ;
#15246=CARTESIAN_POINT ( 'NONE',  ( -25.83226977945856362, 0.3709960288796101402, -16.44840538093085414 ) ) ;
#15250=CARTESIAN_POINT ( 'NONE',  ( 30.76698505935834405, -6.362076114912868618, -13.06728835035745462 ) ) ;
#15265=CARTESIAN_POINT ( 'NONE',  ( 8.135523341600167768, 36.16613191329250299, -6.297504617459584786 ) ) ;
#15269=CARTESIAN_POINT ( 'NONE',  ( 11.21453531681511784, -17.17359087135386631, -29.99999999999999645 ) ) ;
#15275=CARTESIAN_POINT ( 'NONE',  ( -13.89045959741800296, 23.13722222314543941, -14.49167495132802763 ) ) ;
#15278=CARTESIAN_POINT ( 'NONE',  ( 11.44353187076013434, -20.98966551814972803, -19.50774576217023792 ) ) ;
#15282=CARTESIAN_POINT ( 'NONE',  ( -9.499396656360119096, 18.35689620915350417, -27.98656568115667653 ) ) ;
#15283=CARTESIAN_POINT ( 'NONE',  ( -11.59581746604265184, -16.91849113041673647, -30.00000000000000355 ) ) ;
#15286=CARTESIAN_POINT ( 'NONE',  ( -21.60667917395808502, -6.743361281366732740, -23.13545725626142513 ) ) ;
#15287=CARTESIAN_POINT ( 'NONE',  ( -13.54564564923477477, -24.09781583726222465, -13.52072601590651679 ) ) ;
#15290=CARTESIAN_POINT ( 'NONE',  ( 25.09144846651838634, 0.6029723664216483092, -17.46064374251114160 ) ) ;
#15294=CARTESIAN_POINT ( 'NONE',  ( -28.95213599401768434, 0.02960606682219414990, -11.59245046285586156 ) ) ;
#15296=ORIENTED_EDGE ( 'NONE', *, *, #31497, .F. ) ;
#15297=CARTESIAN_POINT ( 'NONE',  ( 20.50115022911059270, -0.2752137519716084113, -30.00000000000000000 ) ) ;
#15298=CARTESIAN_POINT ( 'NONE',  ( 9.908215252718470367, -17.95959716121500449, -30.00000000000000711 ) ) ;
#15301=CARTESIAN_POINT ( 'NONE',  ( -21.05269208634015854, 3.574702288414596474, -24.13667089053400971 ) ) ;
#15312=CARTESIAN_POINT ( 'NONE',  ( -24.20609638677606412, 8.035638068618503382, -5.000000000000000888 ) ) ;
#15315=CARTESIAN_POINT ( 'NONE',  ( 16.13585048104015840, -17.81699276545519339, -20.99261974159198729 ) ) ;
#15318=CARTESIAN_POINT ( 'NONE',  ( 15.26288695882580093, 26.87683090409402098, -6.882367006327409165 ) ) ;
#15320=CARTESIAN_POINT ( 'NONE',  ( -12.94450195943344717, 16.22636800668987078, -26.98281085777279742 ) ) ;
#15323=CARTESIAN_POINT ( 'NONE',  ( 13.78307072732043537, 23.36720680302070363, -14.47774454319189452 ) ) ;
#15324=ORIENTED_EDGE ( 'NONE', *, *, #35287, .F. ) ;
#15325=FACE_OUTER_BOUND ( 'NONE', #21581, .T. ) ;
#15328=CARTESIAN_POINT ( 'NONE',  ( -15.31676148297655615, 27.12555199532522110, -5.000000000000000888 ) ) ;
#15330=CARTESIAN_POINT ( 'NONE',  ( -14.55700941178259633, -25.10763777908611871, -11.58478221798611507 ) ) ;
#15333=CARTESIAN_POINT ( 'NONE',  ( -33.06715563149963089, -18.61836429930299985, -7.543782265277601873 ) ) ;
#15334=CARTESIAN_POINT ( 'NONE',  ( -11.36118072446144645, -25.45899015601136028, -8.329040007300676507 ) ) ;
#15336=CARTESIAN_POINT ( 'NONE',  ( 16.22988331200706469, 23.74208035757151691, -6.896498610208569247 ) ) ;
#15338=CARTESIAN_POINT ( 'NONE',  ( 25.99279172464974508, 5.576676355531687612, -5.956011220400047712 ) ) ;
#15343=ORIENTED_EDGE ( 'NONE', *, *, #3206, .T. ) ;
#15344=CARTESIAN_POINT ( 'NONE',  ( -31.52181932710565349, -0.8163613484490098715, -6.400955463894867137 ) ) ;
#15346=CARTESIAN_POINT ( 'NONE',  ( 30.49808096523472756, -0.1579847061273154385, -8.289727916065702473 ) ) ;
#15351=CARTESIAN_POINT ( 'NONE',  ( 22.40982762235196901, 2.618079236896951656, -21.24786896499729139 ) ) ;
#15360=CARTESIAN_POINT ( 'NONE',  ( 2.942419129403968547, 28.79255951157002613, -16.65093014769575674 ) ) ;
#15369=CARTESIAN_POINT ( 'NONE',  ( 10.36933582218109429, 17.95643907423222885, -27.39330729671292630 ) ) ;
#15372=CARTESIAN_POINT ( 'NONE',  ( -16.69924863411024418, 15.13135123064752996, -18.96634367901145524 ) ) ;
#15375=CARTESIAN_POINT ( 'NONE',  ( 10.83685788847059506, -19.99059525684932481, -21.61737879950500840 ) ) ;
#15376=CARTESIAN_POINT ( 'NONE',  ( -16.85113020441335507, -21.30447706854098300, -16.99219159709304705 ) ) ;
#15377=CARTESIAN_POINT ( 'NONE',  ( -19.48557158514998022, -11.24999999999982414, 0.000000000000000000 ) ) ;
#15379=CARTESIAN_POINT ( 'NONE',  ( 13.48181092597923936, 22.83514489210295650, -15.44851730194768535 ) ) ;
#15383=CARTESIAN_POINT ( 'NONE',  ( -15.43577743098633981, -26.72909887300547283, -5.474191126876100988 ) ) ;
#15385=CARTESIAN_POINT ( 'NONE',  ( -28.90526601420243935, -24.05987742975590749, -6.288601596644300962 ) ) ;
#15386=CARTESIAN_POINT ( 'NONE',  ( -2.597410653098545463, -24.79173595445318767, -5.000000000000000000 ) ) ;
#15387=CARTESIAN_POINT ( 'NONE',  ( 11.26908400546618871, 17.12495040990986794, -29.35441016993270580 ) ) ;
#15388=CARTESIAN_POINT ( 'NONE',  ( 21.64434010710703404, 12.04703973602239842, -4.999999999999996447 ) ) ;
#15390=CARTESIAN_POINT ( 'NONE',  ( -4.537929203215356644, 31.78147521891694893, -13.83853917308986148 ) ) ;
#15392=CARTESIAN_POINT ( 'NONE',  ( -31.16281537880387731, -4.882152567110715324, -12.19897026441750931 ) ) ;
#15396=ORIENTED_EDGE ( 'NONE', *, *, #17261, .F. ) ;
#15401=CARTESIAN_POINT ( 'NONE',  ( -27.28629896358888374, 0.7998108622630019093, -13.54774279276146665 ) ) ;
#15402=CARTESIAN_POINT ( 'NONE',  ( 23.93184905822953468, -8.822957309754631439, -19.71412903833790509 ) ) ;
#15411=CARTESIAN_POINT ( 'NONE',  ( -1.923949180127531244, 38.42603324025853340, -5.000000000000000000 ) ) ;
#15415=CARTESIAN_POINT ( 'NONE',  ( 16.46668505474601929, -12.62653714806953609, -27.72794644683495591 ) ) ;
#15416=CARTESIAN_POINT ( 'NONE',  ( 19.31863883839061558, 15.70629445910060440, -8.886768639220122168 ) ) ;
#15417=AXIS2_PLACEMENT_3D ( 'NONE', #33751, #412, #27835 ) ;
#15418=CARTESIAN_POINT ( 'NONE',  ( 13.68675864763349281, 30.66322818530211691, -6.360680230841967209 ) ) ;
#15421=CARTESIAN_POINT ( 'NONE',  ( -21.10979132117194368, 12.63226555665139728, -7.918966435008256255 ) ) ;
#15423=CARTESIAN_POINT ( 'NONE',  ( 15.44356999697831334, -26.44085754146421507, -7.821532254917190841 ) ) ;
#15426=CIRCLE ( 'NONE', #31001, 16.00000000000000355 ) ;
#15427=CARTESIAN_POINT ( 'NONE',  ( -5.636483973512888213, -22.01575377102104270, -21.50719306941231679 ) ) ;
#15430=CARTESIAN_POINT ( 'NONE',  ( -10.98560485883561455, 17.36128174412877456, -28.70610319738578298 ) ) ;
#15431=CARTESIAN_POINT ( 'NONE',  ( -23.21950482537012661, -25.96020083042891713, -8.516380179814060369 ) ) ;
#15432=CARTESIAN_POINT ( 'NONE',  ( 9.916190783591865454, -21.18337445448872813, -19.66014789460458090 ) ) ;
#15435=CARTESIAN_POINT ( 'NONE',  ( -9.608178598149136107, 29.00351644723056665, -13.99953411183117069 ) ) ;
#15440=CARTESIAN_POINT ( 'NONE',  ( 20.69356520073354133, 0.8462078722227619476, -27.44831186004264367 ) ) ;
#15445=CARTESIAN_POINT ( 'NONE',  ( -23.30142641249946678, 0.5956563822689483478, -20.54734181390668724 ) ) ;
#15448=CARTESIAN_POINT ( 'NONE',  ( 20.27907779278287492, -3.502347089416769865, -28.55884872021393051 ) ) ;
#15449=CIRCLE ( 'NONE', #22569, 17.00000000000000000 ) ;
#15461=DIRECTION ( 'NONE',  ( 1.000000000000000000, 0.000000000000000000, 0.000000000000000000 ) ) ;
#15464=CARTESIAN_POINT ( 'NONE',  ( 9.105319387809036158, 35.54444977581241005, -6.303818603030153511 ) ) ;
#15467=CARTESIAN_POINT ( 'NONE',  ( 13.02764125108839366, -20.75515974360676452, -19.31289340529147580 ) ) ;
#15473=ORIENTED_EDGE ( 'NONE', *, *, #31640, .F. ) ;
#15474=CARTESIAN_POINT ( 'NONE',  ( -15.11124835272140388, 26.10590699377372559, -8.767955561639961815 ) ) ;
#15477=CARTESIAN_POINT ( 'NONE',  ( 15.18788860438108124, -26.66571922823320051, -5.000000000000000888 ) ) ;
#15485=CARTESIAN_POINT ( 'NONE',  ( -11.89628958333163311, 22.12938455673445404, -18.29461116250375596 ) ) ;
#15486=CARTESIAN_POINT ( 'NONE',  ( -12.57245947831582811, -18.18636306848776130, -23.55555282489862279 ) ) ;
#15490=CARTESIAN_POINT ( 'NONE',  ( -33.38568604116227334, -10.36665845154829491, -10.23472671421048652 ) ) ;
#15491=CARTESIAN_POINT ( 'NONE',  ( -14.78550315123711556, -25.94740016304241337, -9.240703662871906587 ) ) ;
#15494=CARTESIAN_POINT ( 'NONE',  ( 29.14303797557771958, 0.3180640978246742079, -10.66026172746647482 ) ) ;
#15498=CARTESIAN_POINT ( 'NONE',  ( -30.53010055481989937, -0.05901878607395646265, -7.825680868720071182 ) ) ;
#15500=CARTESIAN_POINT ( 'NONE',  ( 31.22701752701838274, -1.717445521449697976, -9.600932008253289851 ) ) ;
#15501=CARTESIAN_POINT ( 'NONE',  ( 2.113389199311633604, -20.40176566834144012, -30.00000000000001776 ) ) ;
#15504=EDGE_CURVE ( 'NONE', #7759, #11613, #7221, .T. ) ;
#15505=ORIENTED_EDGE ( 'NONE', *, *, #17867, .T. ) ;
#15506=CARTESIAN_POINT ( 'NONE',  ( -20.57159149025624245, 4.298814444492946585, -25.31853320033998855 ) ) ;
#15509=DIRECTION ( 'NONE',  ( 1.000000000000000000, 0.000000000000000000, 0.000000000000000000 ) ) ;
#15515=B_SPLINE_SURFACE_WITH_KNOTS ( 'NONE', 3, 3, ( 
 ( #6686, #25189, #32085, #22729, #804, #37589, #28236, #13185, #415, #4045, #19094, #16448, #10154, #34937, #31485, #3652, #16045, #37312, #18432, #24518, #34466, #6230, #21864, #9689, #33876, #31413, #30823, #27964, #36918, #37116, #6423, #39756, #36722, #40155 ),
 ( #18235, #12328, #9487, #31021, #9086, #18828, #21668, #8886, #27368, #22066, #21274, #6614, #2990, #12723, #21471, #6028, #11934, #33685, #3380, #15376, #27568, #31216, #27766, #19021, #24716, #24324, #9283, #3187, #15773, #3579, #34069, #39955, #12131, #18632 ),
 ( #15577, #137, #5835, #12527, #37512, #24918, #30629, #34269, #2786, #28163, #339, #25115, #15178, #34122, #27223, #31074, #9340, #24575, #11981, #24171, #15230, #18483, #30277, #24373, #21522, #2840, #8738, #30875, #33738, #8535, #39407, #6279, #20928, #18683 ),
 ( #30480, #21720, #12182, #3239, #14834, #36566, #33337, #2641, #15431, #2449, #30677, #15028, #3038, #33925, #15631, #23975, #27418, #24770, #27821, #5882, #8940, #39807, #18092, #36769, #11587, #33537, #36370, #27616, #5480, #21329, #17894, #36970, #40004, #39609 ),
 ( #9137, #18286, #11784, #12379, #6080, #21127, #4809, #37165, #5681, #25170, #28214, #19268, #37763, #31863, #13374, #31667, #9934, #28615, #10133, #16232, #19075, #22316, #31269, #16428, #34715, #18878, #6868, #22510, #9540, #32065, #28414, #3631, #993, #34518 ),
 ( #21918, #38161, #3832, #4026, #589, #12579, #785, #3432, #25763, #13168, #28818, #25361, #15830, #192, #6668, #25563, #31467, #7268, #12775, #37962, #10331, #4234, #16028, #7071, #34920, #22712, #19469, #35116, #19671, #28017, #24971, #37364, #34320, #6474 ),
 ( #394, #37566, #9736, #22119, #12972, #14182, #39163, #20285, #38563, #26773, #38361, #13574, #16840, #11346, #29621, #22916, #13980, #23332, #4839, #29222, #17248, #32886, #32483, #20492, #33089, #4639, #23728, #7475, #26577, #1598, #35728, #7686, #35925, #23121 ),
 ( #19882, #5040, #38766, #32274, #26371, #11142, #10532, #20695, #17041, #29422, #29822, #35522, #13776, #36127, #26169, #17451, #32684, #20087, #35317, #8290, #10947, #4438, #25960, #16637, #8083, #10736, #1391, #2007, #7879, #14386, #1799, #38968, #23527, #29020 ),
 ( #1194, #24529, #30636, #15385, #36927, #27777, #33884, #27577, #2794, #11941, #15186, #11544, #23931, #33292, #37123, #40164, #39962, #18046, #30232, #21283, #9093, #36327, #30439, #12139, #8893, #14791, #21478, #39762, #14590, #5242, #12335, #26979, #24723, #8695 ),
 ( #9292, #18243, #21677, #20890, #2401, #39365, #36523, #6036, #8491, #36729, #21087, #18441, #30831, #17654, #30027, #33495, #2997, #2204, #24332, #14987, #5634, #33692, #2601, #5445, #17853, #27181, #39566, #27374, #11742, #24127, #5841, #3589, #25122, #12730 ),
 ( #3197, #16186, #28570, #31614, #16385, #37719, #15781, #3983, #15586, #31030, #34278, #28770, #6823, #146, #31422, #545, #22265, #6432, #34670, #10087, #9698, #37915, #10284, #22074, #946, #24927, #3784, #19029, #12929, #37521, #13122, #349, #15984, #34078 ),
 ( #37322, #28365, #744, #27971, #38112, #34474, #6622, #7023, #25320, #31224, #13326, #3388, #22467, #9885, #19224, #12535, #25718, #25513, #9495, #21871, #6237, #34872, #28172, #18836, #19425, #31818, #18639, #32435, #20242, #4594, #16589, #10486, #16994, #11098 ),
 ( #32842, #14136, #4995, #23481, #4793, #7834, #29373, #32640, #28971, #1146, #22868, #14338, #17406, #17200, #35477, #7428, #38723, #1755, #13529, #7633, #29577, #26329, #32225, #26534, #1549, #32020, #22666, #29782, #4186, #1962, #26120, #8036, #4388, #16793 ),
 ( #38314, #19837, #25917, #13728, #38922, #35271, #10899, #29179, #26730, #1345, #19625, #38515, #39116, #35680, #10691, #20040, #13933, #23285, #23078, #35878, #20444, #35070, #7224, #27722, #27131, #18391, #2155, #8847, #36477, #18000, #2358, #30588, #17807, #21038 ),
 ( #39910, #33447, #14537, #5589, #5793, #33047, #15333, #11696, #39519, #24477, #30183, #8448, #30782, #20846, #12088, #27329, #14742, #29975, #2946, #24083, #26932, #8240, #5983, #2745, #33245, #20646, #36873, #8645, #15138, #30387, #21233, #2554, #5197, #39319 ),
 ( #27528, #36677, #21429, #9046, #33835, #11301, #33644, #18195, #14941, #23682, #17606, #11496, #23881, #36080, #36286, #5394, #39717, #11893, #24281, #19172, #30976, #12680, #22214, #3536, #9444, #31566, #34424, #9239, #40110, #34817, #21626, #19373, #3339, #25461 ),
 ( #12878, #31772, #15538, #37269, #34030, #31174, #16134, #3142, #31371, #15731, #3732, #34618, #16335, #24676, #28120, #37861, #28518, #6574, #9647, #298, #18786, #37471, #6969, #34228, #10034, #28317, #12287, #18980, #25274, #6187, #18592, #27922, #3934, #22413 ),
 ( #99, #25075, #6771, #21823, #37070, #12481, #15934, #693, #22025, #498, #37667, #13070, #9836, #24875, #6379, #11051, #22822, #19782, #23435, #1498, #20397, #4133, #25866, #22619, #32177, #4746, #19576, #19990, #4339, #20191, #23237, #4949, #13273, #16744 ),
 ( #28920, #26068, #13889, #7788, #35026, #7178, #38063, #10845, #35630, #26277, #35827, #32386, #10437, #38875, #10233, #25665, #1098, #7984, #38672, #31968, #38469, #35425, #16944, #13478, #29328, #17153, #29125, #32587, #28717, #1297, #32791, #16538, #29529, #13680 ),
 ( #1704, #35218, #10642, #896, #38269, #23025, #14084, #26481, #7379, #7585, #4543, #39269, #15086, #18150, #27477, #33398, #32997, #11247, #39863, #11652, #21187, #30134, #1910, #5540, #5148, #30540, #27084, #33592, #14693, #17554, #29731, #23834, #24033, #8400 ),
 ( #39473, #23636, #29928, #36429, #5744, #14488, #27284, #20797, #26881, #24430, #8592, #11843, #12040, #24232, #39068, #21383, #17759, #33194, #2699, #36240, #11448, #36823, #5345, #8996, #17951, #2307, #36033, #33790, #20991, #20599, #14288, #17355, #8800, #30336 ),
 ( #2508, #26680, #14895, #39669, #36630, #8192, #2108, #250, #34571, #3095, #15888, #37224, #15490, #13026, #25026, #451, #28470, #12433, #9987, #9395, #6528, #27875, #15683, #25226, #18339, #15286, #18739, #12833, #47, #5938, #18540, #9595, #37624, #28071 ),
 ( #27674, #30733, #645, #40061, #25417, #21773, #31524, #24825, #34178, #2896, #12238, #22172, #6330, #6135, #9792, #31128, #37815, #3291, #24628, #12637, #21977, #6722, #22367, #37419, #30930, #34378, #18933, #31321, #19131, #37022, #9192, #21578, #28274, #3687 ),
 ( #3491, #33980, #16085, #35378, #22570, #7327, #11001, #32333, #1252, #10189, #7738, #13428, #31723, #35580, #32126, #3886, #31918, #34979, #26020, #4291, #38620, #20142, #38420, #16691, #7535, #16898, #22975, #25822, #29075, #38016, #23179, #13633, #25617, #10592 ),
 ( #7129, #19938, #38222, #26225, #29279, #34773, #19328, #22770, #32541, #10795, #4495, #1448, #10391, #35172, #13833, #29477, #28874, #4696, #17100, #6922, #1653, #16284, #14035, #26426, #19527, #19734, #28670, #38822, #845, #4085, #13225, #16489, #1049, #24731 ),
 ( #39770, #27786, #152, #11949, #31039, #14237, #21486, #8900, #30643, #14994, #3004, #29874, #33699, #23386, #32739, #27382, #33892, #24538, #37130, #18646, #5097, #17505, #21685, #9302, #34086, #39969, #39018, #17304, #6244, #18252, #40171, #36737, #7935, #12147 ),
 ( #5848, #12342, #21292, #11196, #35781, #2608, #2801, #24339, #3205, #8138, #27585, #15593, #20345, #15194, #15392, #9100, #27979, #4896, #29678, #1860, #6044, #18449, #36934, #30838, #26628, #23587, #35983, #20546, #32939, #37923, #25328, #37529, #28578, #31826 ),
 ( #25129, #16194, #3992, #22274, #13130, #25522, #34880, #752, #10095, #22475, #35080, #6630, #3597, #7234, #7034, #4196, #28178, #9705, #6438, #19634, #19038, #16599, #15994, #19433, #22083, #34678, #16393, #24935, #21877, #37727, #28779, #34483, #12542, #31430 ),
 ( #28373, #955, #6831, #34285, #37328, #32030, #18843, #28980, #554, #38120, #12937, #9894, #9502, #31231, #13334, #19232, #12736, #25727, #31625, #3394, #3793, #15788, #10294, #22677, #357, #17617, #4604, #13740, #1355, #38732, #14146, #20456, #35281, #7439 ),
 ( #11311, #29586, #13539, #10908, #1156, #26544, #1764, #29188, #13943, #25926, #38932, #7845, #16804, #14349, #20050, #38326, #1971, #23295, #10497, #38525, #26129, #32649, #35689, #5004, #26740, #4805, #20252, #11108, #23492, #35887, #32445, #17210, #4397, #29792 ),
 ( #8045, #39126, #36093, #23087, #35486, #23692, #8250, #20657, #32852, #10701, #19846, #33058, #17415, #5207, #26338, #22877, #32235, #7644, #17004, #29384, #1559, #27340, #17818, #2165, #36488, #24292, #21049, #9252, #14753, #33654, #2957, #6197, #33458, #9057 ),
 ( #21440, #40120, #18401, #12101, #15148, #39530, #30195, #33848, #5602, #21636, #18010, #14549, #27143, #5805, #5994, #29988, #30398, #2369, #11706, #39728, #2756, #30793, #23891, #36296, #39331, #24487, #36885, #27539, #12300, #18207, #24094, #24686, #11508, #26943 ),
 ( #39921, #36690, #5405, #15344, #8655, #8458, #27734, #11903, #20857, #2567, #14951, #21245, #8858, #37082, #34041, #30599, #33256, #19185, #703, #6781, #9658, #28328, #21834, #6979, #508, #9455, #12889, #13081, #109, #22628, #18992, #34435, #31782, #25086 ),
 ( #28131, #19383, #34630, #37482, #37280, #10243, #22036, #34238, #15548, #13282, #10046, #15742, #27934, #3944, #6586, #22423, #25285, #16144, #37677, #12492, #6389, #9848, #16344, #309, #28530, #31381, #12691, #25677, #22225, #25472, #906, #3547, #35036, #15946 ),
 ( #18603, #28725, #3742, #31576, #3351, #37871, #34829, #18799, #38072, #30986, #3154, #24886, #31184, #1508, #16548, #7187, #1919, #28929, #26689, #10652, #32801, #16755, #29134, #19586, #1110, #23445, #31978, #35435, #4959, #38884, #13898, #16954, #38479, #26078 ),
 ( #13487, #29538, #1716, #4756, #29740, #10854, #1308, #17366, #25876, #4142, #7388, #14299, #20200, #38279, #4553, #26287, #35639, #19791, #7800, #35836, #23034, #11061, #23644, #7594, #39079, #10447, #17163, #32397, #38682, #19999, #26490, #13689, #29337, #22831 ),
 ( #23246, #35229, #32597, #14094, #32187, #11256, #7995, #20406, #4348, #2315, #33202, #2904, #5354, #24438, #11852, #14703, #14498, #27682, #27093, #39279, #33007, #30743, #27486, #17767, #5156, #21392, #11660, #39871, #5550, #33601, #17959, #29936, #23844, #30347 ),
 ( #21197, #5947, #12048, #18349, #36833, #18158, #5753, #2516, #30550, #2117, #26889, #36248, #40070, #15294, #2707, #8603, #20805, #24241, #15097, #11457, #21000, #9004, #39679, #30144, #33799, #14904, #17563, #36041, #12247, #8410, #8202, #39482, #20608, #24045 ),
 ( #36437, #33407, #27293, #36639, #8808, #653, #15498, #15896, #28080, #16094, #19140, #853, #57, #21782, #18548, #15691, #13035, #27884, #28283, #258, #28479, #31532, #24636, #9202, #12646, #9995, #25425, #18942, #34386, #25034, #3301, #21985, #19337, #18748 ),
 ( #22180, #6929, #459, #6338, #34781, #6146, #21586, #24835, #31730, #37632, #30938, #6537, #31329, #12843, #37233, #25234, #37822, #37428, #22374, #37033, #9604, #3893, #12442, #34581, #3500, #9801, #6732, #3696, #31136, #16292, #33988, #3104, #28677, #9403 ),
 ( #34186, #35179, #7335, #11009, #14043, #23394, #29287, #28881, #7136, #35789, #7545, #17109, #26029, #38023, #1457, #1057, #26434, #22982, #29486, #10600, #13435, #25625, #16906, #35590, #35386, #10804, #19945, #19535, #25830, #32343, #1662, #10399, #23189, #4298 ),
 ( #4503, #7746, #7944, #19741, #17312, #16699, #13842, #22778, #26233, #32549, #10196, #22578, #38428, #20150, #32136, #13233, #38229, #38629, #4705, #38833, #20353, #32748, #4905, #29686, #34987, #31925, #4093, #29083, #1259, #16498, #13641, #33753, #5106, #39027 ),
 ( #39424, #29885, #24390, #17513, #36783, #8955, #21348, #26837, #5496, #15045, #18303, #33150, #21144, #27238, #12000, #33551, #5899, #30497, #24187, #39626, #8551, #11802, #8148, #20554, #2067, #1869, #14247, #36584, #14652, #39228, #17910, #5698, #32948, #27041 ),
 ( #18109, #11608, #2464, #14852, #8755, #30294, #2658, #27436, #26638, #36189, #5304, #11204, #39822, #23595, #14443, #11407, #35991, #17714, #23790, #8358, #33353, #30089, #20758, #2263, #23991, #36388, #20947, #16044, #22136, #24988, #208, #21734, #9355, #28035 ),
 ( #12794, #25188, #28235, #12989, #34342, #12395, #610, #12197, #27637, #30890, #25380, #3452, #36986, #12597, #37383, #18895, #3054, #31287, #6685, #6292, #34535, #6885, #18699, #37778, #21538, #414, #15648, #9557, #34142, #9755, #37183, #21934, #30693, #40018 ),
 ( #33938, #6490, #37587, #24593, #34734, #31092, #3256, #3651, #15848, #27839, #9949, #12, #19093, #31484, #28431, #9152, #22330, #2858, #15246, #24784, #6097, #18501, #15445, #29435, #35336, #34936, #13184, #1613, #13592, #23141, #32084, #3852, #7494, #7089 ),
 ( #13996, #10753, #16447, #19486, #32500, #22936, #1410, #29036, #16861, #1212, #25579, #31882, #25979, #7700, #28833, #29238, #10352, #1010, #26385, #38379, #13793, #38783, #25783, #23348, #22728, #19899, #13391, #10553, #38580, #31681, #28633, #4251, #26186, #38177 ),
 ( #32293, #35538, #4454, #20102, #4656, #17058, #10960, #35742, #19286, #16249, #35135, #7286, #803, #37978, #10153, #4043, #19688, #22525, #16654, #24140, #38983, #39381, #11359, #39582, #2414, #24345, #32700, #36142, #33507, #11755, #2218, #17669, #39180, #26788 ),
 ( #17264, #30246, #14805, #5457, #30451, #11559, #29838, #18059, #29637, #4852, #8097, #2613, #20902, #14196, #5256, #14605, #36342, #20506, #8505, #36537, #23743, #8708, #7897, #8311, #15001, #11155, #17864, #33105, #26994, #20709, #27192, #14402, #30044, #20301 ),
 ( #23946, #23546, #33306, #21099, #1816, #26592, #27388, #35940, #39778, #5649, #11955, #17465, #2022, #32904, #5056, #12743, #6053, #36940, #15795, #27792, #28383, #40177, #21299, #33897, #158, #25137, #12943, #12349, #9106, #21492, #34091, #9507, #28185, #30650 ),
 ( #30844, #6637, #24940, #8909, #6251, #36743, #21887, #37335, #24545, #9308, #33704, #34291, #3211, #12154, #9711, #15401, #5855, #37537, #18654, #18257, #18454, #3010, #27985, #31047, #362, #22091, #12549, #15600, #6445, #18849, #31237, #24736, #3401, #39977 ),
 ( #27590, #34489, #19045, #2808, #560, #37136, #21693, #31436, #3603, #15999, #15201, #35444, #14303, #1723, #4558, #3801, #17570, #32403, #28585, #22282, #20613, #17372, #23039, #13695, #39084, #29543, #8001, #35646, #23451, #7804, #19238, #26083, #20207, #26696 ),
 ( #36046, #29744, #8209, #11262, #20411, #11066, #32603, #35841, #31633, #16199, #38483, #29942, #33012, #32806, #38689, #10658, #14099, #4965, #757, #10862, #1926, #26496, #7599, #23650, #5161, #20004, #2122, #25334, #37734, #16961, #38890, #9902, #34684, #29342 ),
 ( #6836, #1513, #13903, #26293, #4761, #23250, #17168, #21006, #18554, #17966, #15105, #11666, #24249, #33805, #26895, #23849, #27298, #9010, #36444, #14503, #27098, #18164, #5954, #36644, #27492, #39877, #36839, #30555, #12053, #24445, #37039, #8611, #5555, #9210 ),
 ( #30149, #24051, #8416, #30353, #30751, #5360, #5758, #2521, #18356, #21399, #30946, #39283, #14910, #40078, #2910, #8814, #21202, #39687, #33413, #11858, #21594, #33608, #24644, #2714, #11463, #15301, #36252, #27689, #12253, #2321, #33996, #20810, #6153, #33212 ),
 ( #17774, #14710, #39487, #266, #34392, #6347, #21992, #15903, #18754, #31338, #12451, #25040, #31145, #15698, #34194, #9611, #21789, #3307, #3111, #27891, #28087, #6544, #37437, #18948, #3507, #12652, #15506, #64, #24843, #37240, #9409, #2334, #20421, #39497 ),
 ( #23660, #35656, #39295, #26509, #24062, #20624, #14719, #8217, #38900, #11473, #11076, #36057, #27308, #8426, #17581, #23460, #36456, #29759, #7814, #11674, #33025, #20217, #8013, #35852, #2131, #5173, #27108, #8622, #14515, #29953, #23859, #33222, #36263, #1936 ),
 ( #32614, #14314, #20822, #5370, #21017, #5567, #32817, #4973, #33426, #17976, #26908, #30365, #10873, #17178, #2532, #17785, #14919, #30161, #4771, #23262, #17384, #29554, #1733, #14111, #26706, #39094, #11276, #2725, #34403, #22004, #18960, #24454, #3121, #12661 ),
 ( #28097, #36851, #9422, #30763, #9023, #6554, #18568, #34204, #31348, #5963, #3517, #2924, #76, #21408, #9219, #18765, #11870, #8824, #12267, #6357, #33815, #39697, #12065, #15518, #31154, #21604, #12460, #24853, #21802, #27900, #37249, #3318, #15914, #18368 ),
 ( #15312, #24259, #21211, #15709, #27698, #39888, #276, #40090, #36656, #24655, #33621, #37049, #25053, #37448, #5771, #34009, #6167, #30953, #9624, #18173, #30565, #15116, #27505, #37648, #10417, #22798, #25847, #10621, #31945, #10014, #38448, #32365, #874, #29104 ),
 ( #23002, #22597, #32157, #13253, #12859, #16518, #3711, #1277, #38043, #4317, #25645, #16112, #35405, #31547, #7564, #19965, #4524, #13050, #4111, #13660, #28299, #19354, #7356, #13454, #475, #19759, #25253, #16720, #35198, #38248, #35006, #26048, #34598, #6751 ),
 ( #9818, #22195, #19155, #10212, #28498, #22394, #671, #25440, #28901, #37839, #7156, #1078, #34797, #6947, #31751, #3913, #16312, #28695, #19554, #8525, #39995, #30472, #9127, #33123, #14627, #10823, #20920, #33728, #8332, #8729, #33326, #8932, #11975, #33917 ),
 ( #5473, #30064, #17688, #14827, #2632, #36762, #23212, #36162, #26255, #39798, #24365, #15020, #12174, #21120, #39398, #27610, #38651, #13866, #2239, #24568, #27410, #20732, #27213, #24161, #5672, #27015, #18082, #5875, #17886, #21323, #16924, #30269, #36963, #5276 ),
 ( #39602, #18278, #30670, #2832, #2437, #11776, #11579, #15224, #36558, #23967, #33528, #21514, #36362, #29307, #1479, #21907, #9331, #777, #28605, #25552, #31066, #9729, #19258, #22500, #37356, #25353, #31458, #16223, #37755, #13159, #34707, #28406, #3624, #12766 ),
 ( #9531, #6659, #3230, #15820, #9925, #18477, #15421, #18870, #582, #28008, #6072, #18674, #22110, #22306, #28207, #19068, #16019, #12963, #34510, #6858, #31658, #37953, #181, #34312, #10125, #3823, #30867, #21713, #15621, #40198, #6465, #3029, #37157, #37558 ),
 ( #12570, #27814, #12371, #24758, #31261, #24962, #6271, #3424, #34115, #386, #25161, #984, #4017, #17032, #29411, #32475, #17237, #38554, #16628, #4830, #16419, #31855, #35106, #29612, #7675, #13365, #32263, #1383, #23113, #7260, #35512, #10938, #10522, #38756 ),
 ( #4427, #23323, #20276, #10727, #16832, #20077, #1587, #4630, #25952, #29213, #38150, #35718, #13766, #25754, #26157, #13971, #28807, #38959, #35307, #22905, #11131, #7466, #7871, #26363, #4225, #32676, #1789, #13565, #10322, #26569, #1184, #22703, #19660, #14172 ),
 ( #32055, #34910, #7062, #29008, #19459, #38351, #19874, #23519, #18230, #5030, #2782, #26969, #8881, #33081, #5232, #35914, #32876, #39752, #17645, #23720, #2591, #14580, #15173, #39357, #8074, #20686, #27170, #11929, #39949, #11533, #36118, #8278, #20881, #36514 ),
 ( #33284, #30622, #30017, #33680, #11732, #20482, #5434, #17441, #8684, #24117, #11335, #36319, #29814, #21076, #30222, #39153, #36717, #2192, #1998, #24320, #17842, #14376, #23920, #8482, #14781, #2391, #27364, #21270, #39555, #33483, #5625, #18034, #30429, #14975 ),
 ( #5831, #27564, #26763, #21860, #6608, #33871, #16172, #12523, #27959, #28557, #24912, #12916, #3575, #21661, #532, #28158, #31017, #30819, #3769, #18628, #15372, #9081, #6806, #15971, #9279, #40150, #25309, #15768, #34461, #34265, #9685, #6419, #6022, #12324 ),
 ( #31406, #37508, #22251, #28352, #34655, #37706, #19017, #22062, #18824, #9870, #18427, #2984, #24711, #12127, #19211, #31600, #37306, #37111, #334, #24513, #27762, #9481, #36913, #31210, #21466, #34065, #6224, #3375, #12715, #3183, #15572, #25111, #131, #1332 ),
 ( #32006, #10472, #3969, #29358, #22854, #31804, #35259, #35464, #22451, #4780, #1134, #16575, #17188, #13513, #1536, #32422, #10270, #13921, #16779, #19612, #19408, #32626, #7211, #16369, #37898, #35667, #4579, #38097, #28756, #26315, #4373, #23061, #7413, #38503 ),
 ( #38708, #731, #4171, #20025, #26104, #10887, #16981, #23270, #7822, #7620, #10678, #19823, #20227, #7008, #930, #13308, #13109, #25499, #10072, #25903, #25703, #29163, #34860, #22651, #38301, #35056, #13714, #28954, #32210, #23870, #38909, #29563, #24270, #11086 ),
 ( #23670, #20634, #11878, #2343, #21220, #4983, #26718, #23469, #33034, #5575, #20430, #20832, #5183, #21026, #24071, #5780, #14122, #17594, #14929, #33435, #36272, #39305, #29963, #8228, #26917, #36664, #36066, #39705, #17796, #1742, #11483, #26521, #14729, #30170 ),
 ( #29767, #8834, #27119, #35862, #8436, #33234, #39506, #1949, #2142, #8024, #33631, #14526, #32827, #17394, #14324, #17985, #39103, #11287, #2540, #5380, #11683, #36464, #8633, #30376, #27316, #5971, #12468, #6561, #15320, #28106, #9226, #27706, #25258, #37257 ),
 ( #24861, #3327, #24464, #36862, #18377, #9823, #28304, #15716, #30962, #2931, #34212, #37456, #9031, #3129, #284, #21809, #40099, #9632, #9430, #27514, #18182, #12865, #39898, #37654, #21612, #3524, #12275, #24662, #30575, #12074, #34410, #37058, #30771, #22012 ),
 ( #34017, #2733, #6174, #6367, #18967, #34605, #18575, #15526, #27909, #84, #31162, #31355, #21417, #33823, #18772, #12668, #25061, #15920, #482, #22201, #15124, #16931, #28503, #3717, #6952, #1485, #19769, #13056, #4119, #13461, #35203, #19360, #7363, #23010 ),
 ( #31757, #38254, #16524, #10627, #32373, #10423, #28907, #32163, #29111, #4324, #38048, #1085, #10021, #35412, #25853, #37845, #22806, #1283, #676, #10831, #7163, #22605, #23221, #19561, #7570, #38454, #16318, #19974, #16728, #13665, #26055, #4529, #25445, #34802 ),
 ( #29315, #13874, #26264, #38658, #6757, #19160, #31552, #16120, #22399, #3919, #28703, #881, #13260, #25652, #10218, #35012, #31951, #20383, #11436, #14681, #26464, #8179, #17744, #39256, #4936, #27070, #29915, #4732, #35618, #30322, #17139, #14882, #39056, #20977 ),
 ( #8387, #27268, #11038, #32778, #29516, #26666, #11638, #38862, #26867, #11233, #39456, #30121, #11828, #20177, #23623, #33384, #24019, #2095, #5135, #36021, #14275, #32981, #2493, #29716, #5527, #23819, #7775, #17541, #32574, #20784, #36224, #23422, #20585, #1691 ),
 ( #14068, #14475, #33181, #5331, #7971, #2293, #36415, #8578, #17939, #35814, #39655, #17340, #1898, #21761, #9181, #30919, #15275, #3279, #30722, #33966, #24217, #33577, #27663, #34167, #24814, #37408, #18922, #5926, #18326, #21966, #25013, #27865, #238, #439 ),
 ( #18527, #28059, #37010, #8784, #12422, #39851, #9582, #6123, #12624, #21566, #12027, #6514, #27463, #31310, #3479, #3082, #37211, #9381, #6318, #35, #18726, #31116, #15876, #2884, #40047, #28262, #15672, #36615, #24417, #21372, #18137, #12226, #34367, #15073 ),
 ( #21174, #33777, #5728, #30526, #2686, #24618, #36811, #8982, #15474, #25813, #32114, #6711, #19120, #22160, #35161, #7316, #10380, #35367, #16477, #34762, #22963, #34561, #9780, #13017, #7522, #38211, #31514, #10180, #19516, #1038, #25406, #13419, #29064, #28660 ),
 ( #832, #19927, #3677, #22757, #38006, #31907, #3877, #4278, #19315, #22558, #12820, #16071, #16273, #19723, #16682, #26008, #32322, #6913, #31710, #10581, #13623, #28862, #1241, #29268, #28459, #4484, #7118, #38406, #25606, #37615, #16888, #635, #25214, #34966 ),
 ( #9976, #37803, #22355, #13212, #4074, #11184, #39209, #23575, #35566, #29463, #35972, #30072, #38811, #11389, #32728, #10988, #8533, #20533, #36171, #23973, #7925, #5479, #4882, #2047, #23376, #8126, #20738, #13820, #10784, #14224, #8338, #35770, #1437, #14023 ),
 ( #5085, #14425, #23770, #36369, #20334, #17294, #20927, #26819, #33335, #17088, #29667, #7728, #1849, #17696, #32530, #32930, #26616, #33132, #5282, #17893, #26214, #39008, #27024, #2246, #17494, #29863, #14633, #39406, #11586, #38607, #23168, #20132, #4685, #1642 ),
 ( #26417, #191, #11782, #27221, #30478, #24970, #3036, #36564, #27615, #36968, #18482, #2640, #30874, #6278, #5881, #34121, #7018, #18284, #37363, #21126, #27820, #15229, #9136, #21328, #9339, #36767, #40002, #30275, #39608, #33736, #8050, #15430, #3237, #9539 ),
 ( #30676, #2838, #34319, #12181, #31073, #21719, #39806, #18682, #6078, #8939, #8737, #21917, #24574, #33535, #24170, #2448, #15630, #27417, #18091, #28015, #33924, #12378, #21519, #24768, #37164, #5680, #15026, #12577, #14833, #11980, #24372, #10482, #16584, #26529 ),
 ( #4589, #26115, #16990, #25714, #38108, #7220, #11094, #29571, #29368, #32220, #4181, #35473, #38717, #10279, #4383, #1545, #23070, #28966, #10895, #13724, #28765, #19421, #4789, #1142, #13523, #31813, #941, #35676, #25913, #19620, #23278, #22863, #23477, #35267 ),
 ( #13929, #35873, #3979, #7422, #17196, #7830, #38511, #29175, #19831, #38310, #16787, #14130, #1340, #1751, #7628, #16379, #10686, #13319, #26323, #20034, #32014, #32431, #22662, #20238, #32635, #35065, #38917, #26927, #4991, #8842, #5388, #17402, #5191, #8236 ),
 ( #11886, #33640, #11692, #17803, #8640, #30383, #36471, #39313, #30177, #11297, #36671, #2353, #39111, #14737, #2548, #29775, #12082, #8444, #23877, #24472, #20839, #21228, #39712, #17601, #5787, #24078, #11492, #26725, #39905, #14533, #23677, #1958, #2741, #24277 ),
 ( #18191, #21033, #14937, #27127, #5583, #39513, #14332, #36075, #33442, #30583, #29970, #17995, #36280, #2150, #15133, #27324, #27522, #8032, #33241, #20439, #32836, #20642, #33041, #6374, #15929, #9040, #5979, #9438, #31365, #18584, #36869, #9235, #293, #28311 ),
 ( #31169, #18386, #21425, #31560, #30778, #16129, #93, #18975, #12675, #37465, #6568, #19167, #30970, #27917, #3726, #9640, #28512, #12282, #34025, #2939, #12476, #12873, #27715, #28114, #24870, #492, #3531, #13064, #33831, #37264, #22209, #25266, #3334, #18779 ),
 ( #15328, #40106, #24672, #37662, #9830, #34418, #686, #25069, #3136, #6766, #37065, #21620, #6181, #15533, #22019, #21817, #34221, #15726, #34613, #38057, #13675, #1492, #1093, #29323, #1699, #13472, #32581, #16327, #23018, #10432, #32171, #16532, #4537, #31960 ),
 ( #28711, #13883, #7371, #889, #35212, #19984, #6963, #29524, #25861, #38263, #25454, #22816, #26272, #16939, #35020, #38665, #1291, #4127, #3929, #17146, #28915, #13268, #22408, #20186, #10838, #22614, #25660, #23230, #29120, #7578, #19777, #35420, #4332, #19368 ),
 ( #16738, #35625, #10636, #7782, #4740, #37855, #10029, #32380, #34810, #26063, #31766, #10227, #7173, #19570, #38463, #24226, #39465, #26875, #39063, #30128, #33393, #4944, #39264, #36423, #17753, #23630, #5535, #8395, #36028, #14282, #17946, #5142, #5738, #17548 ),
 ( #8587, #30534, #38869, #2103, #39664, #30329, #20791, #23826, #29922, #32991, #11443, #8795, #8186, #36623, #2302, #26474, #36233, #14075, #11646, #14688, #1905, #33189, #11046, #24028, #5339, #29725, #27278, #14482, #23430, #14889, #27077, #35822, #11241, #26675 ),
 ( #2502, #11837, #20984, #21182, #33585, #18145, #7978, #20391, #32785, #17348, #20593, #24821, #33784, #12429, #37415, #24425, #6718, #3088, #18535, #19126, #15485, #3486, #34373, #12233, #31317, #18734, #21573, #21378, #34568, #9188, #5933, #39857, #37621, #6524 ),
 ( #25223, #18334, #9788, #22169, #2693, #27669, #6324, #15882, #15081, #33974, #21973, #28066, #12827, #18929, #27470, #28269, #25021, #245, #9388, #12630, #8990, #30729, #2890, #12034, #36817, #9589, #27871, #40055, #31124, #446, #15282, #43, #24624, #3287 ),
 ( #15679, #37017, #6130, #30925, #37218, #21769, #34174, #25612, #22565, #13828, #4288, #23175, #6919, #28667, #840, #31719, #22766, #1046, #35373, #16894, #35168, #13425, #32121, #13630, #19730, #34974, #25819, #34770, #19935, #38219, #22361, #10386, #26016, #13023 ),
 ( #29276, #32328, #7324, #7531, #7735, #37812, #1443, #16688, #4492, #4081, #16079, #29070, #19322, #26221, #1249, #38615, #28870, #3883, #10792, #16281, #35574, #31521, #3683, #13221, #38415, #28467, #642, #7125, #10588, #22971, #25413, #9983, #38013, #10186 ),
 ( #19524, #31915, #16484, #26423, #7931, #11792, #30283, #5291, #32936, #4890, #36178, #39412, #10998, #5093, #2251, #23778, #29675, #11595, #14431, #29472, #20138, #14839, #1648, #39614, #23582, #5486, #1855, #14233, #32538, #14032, #36377, #26624, #20341, #23981 ),
 ( #11395, #35979, #8541, #14638, #36572, #4692, #8132, #17899, #20935, #26826, #29870, #11192, #39015, #17502, #27229, #20542, #2454, #8344, #17095, #2056, #38818, #17703, #20748, #32734, #39216, #23382, #30078, #33138, #35778, #33343, #27031, #17301, #24177, #6085 ),
 ( #15034, #18097, #31079, #3247, #6283, #31277, #12383, #30683, #18886, #30486, #5686, #8945, #3440, #21724, #27426, #18490, #15435, #37170, #21334, #9344, #24977, #24580, #12585, #25179, #36975, #15837, #39812, #18688, #33929, #27826, #40009, #28023, #15235, #30879 ),
 ( #12187, #15637, #34129, #21924, #28221, #2847, #27622, #6481, #9548, #24774, #11987, #3043, #18292, #37370, #199, #9141, #24378, #401, #21526, #36774, #2647, #12782, #34327, #5887, #33744, #8744, #21132, #33542, #3, #35123, #19477, #31474, #25369, #31873 ),
 ( #22720, #7484, #29027, #19889, #25968, #19678, #7278, #4034, #32073, #3638, #16035, #37770, #29229, #32282, #4241, #10141, #22323, #13381, #16645, #28421, #22517, #1202, #1001, #6875, #13581, #16437, #6676, #37573, #4445, #19082, #16848, #793, #22926, #19275 ),
 ( #1398, #12980, #34723, #598, #28623, #38368, #9942, #28825, #13176, #10541, #35324, #13784, #22126, #25571, #9745, #34526, #25771, #7078, #37969, #16242, #31674, #3839, #34927, #38169, #10338, #2406, #17254, #5249, #11352, #36334, #17660, #8498, #14596, #8297 ),
 ( #32691, #30237, #29628, #26779, #23339, #35932, #30035, #38572, #35528, #38976, #20702, #7886, #26176, #38773, #29829, #2210, #8089, #39170, #23734, #33095, #2014, #36133, #26985, #20896, #20292, #1806, #33297, #39371, #17858, #1604, #35735, #20093, #14189, #11550 ),
 ( #26583, #10743, #4845, #14394, #23937, #23130, #11147, #10953, #26377, #23535, #5451, #7693, #32491, #4645, #17048, #29428, #13988, #20498, #32892, #5047, #17457, #34084, #24132, #39572, #30444, #18644, #21484, #8700, #2799, #27583, #9098, #2606, #33890, #12340 ),
 ( #18051, #12145, #15192, #40169, #9299, #24535, #39967, #6042, #30836, #18447, #36735, #36932, #5639, #24729, #3002, #21093, #15390, #27783, #36529, #15591, #33697, #21288, #37128, #5846, #33501, #21683, #27380, #6242, #31035, #8898, #14992, #3203, #11947, #39768 ),
 ( #27977, #30641, #24337, #14796, #18250, #27186, #11749, #39987, #30859, #6457, #24558, #18664, #12756, #34502, #12561, #31057, #9522, #31251, #37348, #40189, #3222, #12164, #37550, #15611, #36954, #27999, #3415, #30661, #12955, #9322, #24749, #28196, #37147, #15215 ),
 ( #173, #25149, #21704, #33720, #21898, #9119, #22101, #24953, #9721, #6263, #21503, #31449, #33909, #3615, #16011, #28394, #6063, #34303, #6650, #25344, #12361, #378, #18861, #19058, #572, #8921, #21313, #15811, #5865, #18270, #2822, #27603, #18467, #3021 ),
 ( #15411, #27804, #34106, #10311, #32254, #19449, #37745, #10114, #1173, #16820, #7250, #38341, #10511, #19864, #13555, #22894, #7455, #20067, #31844, #28797, #32463, #35297, #29401, #13150, #34897, #31645, #973, #13755, #28595, #28997, #13353, #29203, #4416, #13960 ),
 ( #25744, #22491, #37941, #35095, #1371, #26146, #3812, #16212, #6849, #38544, #10716, #23103, #4620, #25942, #4007, #7664, #19248, #34695, #7052, #17019, #35503, #767, #19650, #4213, #1575, #16409, #25542, #38138, #9916, #22295, #22694, #32046, #16618, #14567 ),
 ( #23707, #17224, #8062, #23906, #1780, #36108, #30208, #11720, #30005, #8266, #26957, #8471, #39344, #17430, #20673, #29601, #14769, #33070, #14161, #5221, #20871, #7861, #30415, #26752, #1987, #5424, #14366, #32664, #17633, #35904, #27158, #2181, #5020, #4821 ),
 ( #26560, #39543, #11523, #2380, #36308, #38949, #8672, #11121, #21065, #33471, #5613, #23506, #33271, #24106, #2580, #29804, #17830, #36503, #18024, #26353, #38747, #10927, #23313, #35707, #20265, #20471, #32864, #39142, #11325, #6598, #25099, #122, #27752, #39936 ),
 ( #36901, #14963, #27553, #18618, #34255, #24701, #15561, #27948, #37294, #31005, #12509, #24902, #37497, #9070, #6010, #9673, #9469, #19005, #30610, #12117, #8870, #18417, #31198, #5818, #6212, #30807, #6405, #21848, #31396, #39740, #2972, #323, #18813, #9267 ),
 ( #3364, #21260, #33668, #24307, #15756, #28146, #12702, #22049, #3172, #21454, #34450, #36706, #27352, #11918, #18220, #33862, #2770, #15163, #24502, #15360, #40138, #12313, #37099, #21650, #34054, #32563, #16158, #4721, #20372, #25299, #28543, #4923, #14058, #11222 ),
 ( #7763, #13862, #17128, #26451, #29504, #34844, #26251, #6795, #32766, #38647, #34644, #10820, #38850, #37693, #8167, #4521, #19396, #23409, #32359, #9861, #23209, #13094, #17329, #20166, #22438, #22239, #36009, #10059, #19199, #522, #39043, #35804, #718, #31588 ),
 ( #11027, #35606, #1679, #7959, #3756, #25485, #29704, #1885, #37885, #14265, #6995, #16920, #23612, #26653, #20573, #3562, #29304, #15960, #1475, #28340, #12903, #2482, #12017, #5123, #2083, #5513, #27452, #14669, #32968, #5320, #36603, #24405, #14870, #33567 ),
 ( #17530, #27654, #14461, #12217, #36404, #18318, #2280, #27060, #29903, #26855, #8974, #39445, #33168, #36800, #24008, #24609, #8566, #39245, #30107, #8770, #21363, #9171, #20965, #17731, #11625, #30312, #5717, #33770, #11425, #23809, #36211, #15062, #39838, #8374 ),
 ( #5917, #30711, #30516, #15265, #21160, #33370, #2876, #20774, #17927, #27256, #40038, #18126, #39642, #11817, #24204, #2675, #37003, #9775, #37795, #3075, #6312, #22348, #31505, #28651, #12413, #19113, #6508, #28257, #12618, #627, #28052, #31305, #21558, #30908 ),
 ( #24805, #3473, #16064, #15464, #25599, #21957, #37399, #13009, #9577, #27855, #15868, #31108, #9969, #37606, #231, #28, #13204, #25006, #37204, #18519, #16267, #25398, #18720, #9375, #34754, #25208, #3671, #431, #28452, #12814, #21752, #34160, #22152, #6904 ),
 ( #31702, #19309, #3869, #825, #37998, #6705, #34554, #33956, #3273, #15665, #34360, #6113, #18914, #35557, #22954, #35152, #26204, #29453, #1029, #35357, #32522, #13811, #19711, #1633, #4474, #19507, #10173, #4870, #31899, #29657, #13611, #35761, #32104, #4268 ),
 ( #25805, #7307, #4064, #1232, #26404, #13410, #1429, #26000, #14015, #4674, #26607, #34959, #38397, #7917, #38803, #16878, #19916, #10572, #7109, #10371, #17285, #23158, #16469, #7512, #29258, #38598, #22748, #10772, #10978, #28852, #16673, #23366, #20121, #1840 ),
 ( #7719, #32314, #17079, #20322, #32719, #14217, #22549, #38200, #29055, #20918, #29855, #8523, #33526, #20524, #2830, #39396, #14624, #18080, #27013, #5078, #33324, #8330, #27408, #14825, #17686, #17484, #30668, #5274, #2039, #35961, #33726, #30470, #36159, #26811 ),
 ( #21118, #5471, #36556, #17884, #32920, #39200, #30266, #39796, #20730, #8726, #30062, #33121, #5873, #2434, #5668, #21320, #2236, #15221, #11577, #39600, #23965, #27211, #2630, #11175, #8117, #36360, #15018, #11774, #39001, #11379, #24159, #11972, #24363, #36760 ),
 ( #23567, #18276, #14417, #23762, #8929, #12961, #37155, #9329, #39993, #36960, #3622, #21710, #27812, #6657, #18671, #19255, #31064, #12171, #24756, #31259, #16017, #3820, #3228, #40196, #12368, #24959, #384, #19065, #21512, #33915, #9125, #9727, #22108, #25158 ),
 ( #27608, #12764, #28204, #15418, #34113, #37752, #21904, #31455, #179, #24566, #15818, #3027, #580, #37354, #28403, #9529, #6269, #9922, #30865, #22303, #34702, #6855, #15619, #3421, #25351, #6070, #28005, #31654, #37556, #18474, #12568, #34310, #6463, #34508 ),
 ( #18868, #20272, #19657, #16828, #13361, #25949, #35509, #28602, #25549, #29004, #10723, #38146, #16220, #28804, #19871, #7671, #38348, #29209, #1380, #38551, #32260, #13762, #26154, #38753, #10319, #7257, #10934, #23110, #7867, #31852, #25750, #10121, #32052, #32470 ),
 ( #4221, #774, #22700, #4423, #4627, #32673, #16625, #980, #16416, #13562, #20074, #17028, #22497, #34906, #37949, #29408, #1584, #13968, #23320, #26360, #35103, #35714, #7059, #13156, #1179, #19456, #4014, #10518, #22902, #35304, #7462, #17437, #33280, #21073 ),
 ( #5622, #14778, #11926, #35911, #2388, #30013, #11530, #36115, #24114, #11332, #14576, #4827, #14168, #8275, #27166, #5431, #18031, #39748, #26760, #39149, #2588, #30425, #23716, #26965, #39552, #17839, #11728, #30217, #20682, #39354, #8071, #33479, #23916, #20478 ),
 ( #24317, #33078, #5228, #14971, #27361, #17642, #36316, #36510, #2189, #36714, #8478, #8681, #20878, #29609, #8878, #32873, #21267, #17233, #1786, #26566, #5027, #38955, #29811, #11128, #23514, #1994, #14373, #37303, #6605, #9867, #24708, #12711, #18821, #3572 ),
 ( #22059, #15764, #31206, #128, #3372, #39946, #12124, #21463, #25306, #15967, #28155, #6220, #18424, #9477, #25107, #24510, #18625, #331, #21857, #2980, #37505, #27955, #2778, #33676, #28348, #15170, #12912, #37108, #19013, #15369, #27759, #5828, #27561, #9681 ),
 ( #9275, #34457, #36909, #24909, #21658, #31403, #529, #18227, #30619, #34062, #37702, #9078, #12519, #3179, #31014, #12321, #15569, #33868, #40146, #6019, #34262, #30816, #6415, #38705, #7411, #22851, #10069, #35053, #22247, #19820, #28951, #37895, #35461, #927 ),
 ( #10468, #38499, #3766, #7005, #23058, #32208, #29355, #13106, #4370, #7207, #19405, #25899, #7616, #34652, #13305, #1329, #16776, #32418, #13710, #4576, #10675, #29159, #26101, #1130, #20022, #28554, #727, #22448, #13918, #16977, #1532, #19609, #31801, #38298 ),
 ( #6803, #34856, #35254, #26312, #32002, #19208, #31596, #16168, #25495, #3965, #16366, #28752, #25700, #38093, #10267, #22647, #4168, #16572, #13510, #4777, #1945, #27115, #1739, #2138, #14321, #2340, #5376, #27313, #35663, #39099, #36461, #14726, #5179, #20630 ),
 ( #17185, #29560, #20223, #33230, #17792, #8432, #33432, #14521, #32824, #21022, #32622, #7820, #11084, #5572, #23866, #14118, #8224, #17591, #39302, #23466, #11479, #39503, #26518, #35858, #11679, #20829, #17981, #38906, #30167, #36063, #29959, #26714, #24068, #17391 ),
 ( #8020, #8629, #33031, #20427, #26914, #30372, #4979, #14925, #11283, #23667, #2537, #36269, #29765, #10883, #23268, #28103, #15524, #18374, #18178, #31352, #5969, #2730, #36661, #34408, #31160, #36858, #27510, #12666, #3127, #21807, #9224, #37254, #39895, #34015 ),
 ( #24858, #9629, #3325, #22010, #281, #34209, #9428, #6172, #6364, #5777, #30572, #12071, #3521, #6559, #18770, #12273, #24460, #27907, #15714, #15121, #24660, #25059, #82, #9028, #37453, #18573, #8831, #39702, #18965, #21216, #15918, #2929, #11875, #21414 ),
 ( #33627, #24266, #33821, #30768, #15318, #27703, #40097, #37056, #21609, #30959, #12466, #4322, #4527, #31755, #674, #28501, #25650, #1083, #7360, #22199, #34602, #37652, #10421, #22804, #25851, #10624, #31949, #10018, #38452, #9821, #25256, #13054, #23007, #13458 ),
 ( #35010, #16521, #25443, #28905, #16725, #6754, #37843, #29109, #38252, #35410, #19158, #35201, #13258, #7161, #19358, #19766, #34800, #38046, #28302, #31550, #3917, #32161, #1281, #13663, #7568, #22397, #6949, #26053, #19971, #16316, #10215, #32371, #28701, #479 ),
 ( #878, #3714, #12863, #22602, #16117, #19559, #4116, #8385, #14066, #4730, #30118, #20582, #39253, #26664, #14473, #39054, #10829, #17742, #26864, #24017, #7773, #11434, #1896, #23621, #7969, #36220, #23420, #11231, #16929, #26261, #20381, #23817, #17539, #2290 ),
 ( #20975, #17338, #32775, #20782, #4934, #23218, #36018, #26461, #5329, #32978, #35812, #35616, #8576, #29713, #20175, #13871, #11636, #33179, #38860, #17136, #14679, #5133, #27068, #8177, #39453, #29913, #32572, #29514, #2093, #36413, #11036, #33381, #14273, #29313 ),
 ( #1483, #38656, #1689, #31462, #11826, #24215, #33575, #37959, #16228, #3628, #18875, #30524, #22116, #25358, #36612, #31266, #28410, #9733, #15627, #37760, #390, #14880, #5524, #782, #27266, #25558, #9535, #31663, #28012, #185, #17937, #39653, #22312, #12574 ),
 ( #34712, #8781, #37563, #21912, #9930, #586, #22505, #30320, #34316, #3829, #6863, #12770, #15824, #37360, #24966, #3428, #13165, #6470, #28612, #34514, #2490, #28211, #21172, #16023, #6664, #5725, #25165, #18135, #12968, #19072, #3234, #19263, #10130, #31860 ),
 ( #10942, #16424, #19667, #28814, #25957, #23328, #25759, #26165, #38357, #26368, #29417, #11138, #19465, #22911, #20281, #38761, #29218, #4433, #10529, #13570, #32268, #29617, #29014, #4835, #23118, #7067, #16837, #34915, #20083, #35517, #22708, #7472, #4023, #32480 ),
 ( #7876, #35313, #989, #35724, #1388, #38155, #16633, #4635, #10328, #13772, #32681, #17245, #38559, #10733, #7680, #17037, #1594, #19879, #13977, #35113, #1794, #14177, #7265, #26574, #38964, #13371, #32061, #4231, #1189, #2596, #39362, #29819, #5440, #33086 ),
 ( #27370, #36324, #8079, #11738, #39159, #36724, #33289, #39758, #20887, #11341, #5837, #26769, #18237, #30631, #2789, #8285, #27175, #8888, #39957, #14585, #14983, #8690, #33688, #11936, #15180, #24326, #5630, #21081, #30228, #33490, #2004, #14382, #23725, #27570 ),
 ( #35920, #32883, #8488, #18040, #5239, #23524, #36123, #39562, #21276, #17848, #24123, #36519, #30434, #20488, #5035, #17446, #20691, #17651, #26976, #30023, #2199, #11538, #23927, #2397, #14786, #140, #37714, #3581, #6425, #21866, #3189, #31023, #9489, #6815 ),
 ( #34468, #9691, #34663, #15775, #34071, #22259, #33878, #9088, #12330, #19219, #25117, #18434, #34271, #18830, #341, #24718, #12725, #28360, #6030, #37118, #12922, #22068, #31608, #2992, #6616, #37314, #31218, #15580, #31415, #18634, #3382, #12133, #21473, #27966 ),
 ( #25315, #3778, #6232, #12529, #9878, #16179, #24920, #28165, #19023, #37514, #28564, #15979, #538, #24520, #36920, #30825, #27768, #15379, #40157, #9285, #21670, #28763, #23276, #3977, #35674, #7828, #20236, #25712, #4381, #13927, #17194, #32012, #20032, #26112 ),
 ( #38106, #32633, #19829, #35471, #4787, #7218, #739, #4178, #1338, #10277, #10480, #32428, #13117, #10079, #13521, #7626, #22658, #25506, #13316, #16785, #4587, #22861, #13722, #38509, #23067, #29171, #10684, #16988, #37907, #35063, #16581, #22462, #29366, #34867 ),
 ( #19618, #938, #1543, #28964, #7016, #1140, #19417, #25909, #26321, #38308, #38715, #10893, #31811, #16377, #35265, #7419, #32218, #30381, #8234, #11490, #39511, #36072, #39710, #23875, #33440, #2148, #14128, #17801, #4989, #2546, #39310, #5580, #26925, #17400 ) ),
 .UNSPECIFIED., .F., .F., .F.,
 ( 4, 3, 3, 3, 3, 3, 3, 3, 3, 3, 3, 3, 3, 3, 3, 3, 3, 3, 3, 3, 3, 3, 3, 3, 3, 3, 3, 3, 3, 3, 3, 3, 3, 3, 3, 3, 3, 3, 3, 3, 3, 3, 3, 3, 3, 3, 3, 3, 3, 3, 3, 4 ),
 ( 4, 3, 3, 3, 3, 3, 3, 3, 3, 3, 3, 4 ),
 ( 0.5000000000000000000, 0.5156250000000000000, 0.5312500000000000000, 0.5468750000000000000, 0.5625000000000000000, 0.5781250000000000000, 0.5937500000000000000, 0.6093750000000000000, 0.6250000000000000000, 0.6406250000000000000, 0.6562500000000000000, 0.6640625000000000000, 0.6660156250000000000, 0.6665039062500000000, 0.6667480468750000000, 0.6669921875000000000, 0.6679687500000000000, 0.6718750000000000000, 0.6875000000000000000, 0.7031250000000000000, 0.7187500000000000000, 0.7343750000000000000, 0.7500000000000000000, 0.7656250000000000000, 0.7812500000000000000, 0.7968750000000000000, 0.8046875000000000000, 0.8085937500000000000, 0.8088378906250000000, 0.8090820312500000000, 0.8095703125000000000, 0.8105468750000000000, 0.8125000000000000000, 0.8281250000000000000, 0.8437500000000000000, 0.8593750000000000000, 0.8750000000000000000, 0.8906250000000000000, 0.9062500000000000000, 0.9218750000000000000, 0.9375000000000000000, 0.9531250000000000000, 0.9687500000000000000, 0.9843750000000000000, 0.9921875000000000000, 0.9960937500000000000, 0.9980468750000000000, 0.9990234375000000000, 0.9995117187500000000, 0.9997558593750000000, 0.9998779296875000000, 1.000000000000000000 ),
 ( 0.000000000000000000, 0.06250000000000011102, 0.1250000000000002220, 0.1875000000000003331, 0.2500000000000004441, 0.3750000000000006661, 0.5000000000000008882, 0.6250000000000011102, 0.7500000000000013323, 0.8750000000000015543, 0.9375000000000016653, 1.000000000000001776 ),
 .UNSPECIFIED. ) ;
#15518=CARTESIAN_POINT ( 'NONE',  ( -20.63291709985350053, 6.542238888207103642, -22.14536008743868933 ) ) ;
#15521=CARTESIAN_POINT ( 'NONE',  ( 13.74558791142738912, -15.22183123319548770, -29.25951782139146928 ) ) ;
#15522=DIRECTION ( 'NONE',  ( -1.000000000000000000, 0.000000000000000000, 0.000000000000000000 ) ) ;
#15524=CARTESIAN_POINT ( 'NONE',  ( 13.63088033700408452, 23.70229946530109899, -14.44436252122576114 ) ) ;
#15526=CARTESIAN_POINT ( 'NONE',  ( -15.81766387322535294, 24.25203275818095960, -8.314427518714673226 ) ) ;
#15529=CARTESIAN_POINT ( 'NONE',  ( 15.39433494388958046, 26.59358880772150258, -6.417088570401624281 ) ) ;
#15532=ORIENTED_EDGE ( 'NONE', *, *, #17867, .F. ) ;
#15533=CARTESIAN_POINT ( 'NONE',  ( -14.42407661054300583, 25.27392573504564410, -11.57633654154478720 ) ) ;
#15535=CARTESIAN_POINT ( 'NONE',  ( -9.875123302056525887, -18.52367353807504102, -26.21621392048563948 ) ) ;
#15538=CARTESIAN_POINT ( 'NONE',  ( -34.49769457167991504, -16.76017602247890892, -5.856898327356995893 ) ) ;
#15539=CARTESIAN_POINT ( 'NONE',  ( -8.962781483812664263, -18.91548421640152711, -26.29799973468894692 ) ) ;
#15541=CARTESIAN_POINT ( 'NONE',  ( 15.31670069829342573, 22.92704149593691554, -11.66084285614651250 ) ) ;
#15543=CARTESIAN_POINT ( 'NONE',  ( 19.75709278228214316, 5.918078465942131494, -27.67886744341916128 ) ) ;
#15546=CARTESIAN_POINT ( 'NONE',  ( -16.05099854214882171, -21.51520587156189279, -17.05908743440501851 ) ) ;
#15548=CARTESIAN_POINT ( 'NONE',  ( -30.53615654196750739, -0.3717794457668220920, -8.746079897285124360 ) ) ;
#15549=CARTESIAN_POINT ( 'NONE',  ( 30.58646958062722732, -0.2537825805908827115, -8.284971368571740769 ) ) ;
#15554=CARTESIAN_POINT ( 'NONE',  ( 19.69645987729881043, 11.37175641224107814, -21.56489709563629376 ) ) ;
#15561=CARTESIAN_POINT ( 'NONE',  ( 2.710501123038885130, 37.71647222079759132, -7.547886179347838009 ) ) ;
#15569=CARTESIAN_POINT ( 'NONE',  ( 13.39086794456952489, 24.19890610734487879, -14.39401347409533471 ) ) ;
#15572=CARTESIAN_POINT ( 'NONE',  ( -14.97876122052304027, 14.11420655003455593, -28.25524194599643835 ) ) ;
#15573=CARTESIAN_POINT ( 'NONE',  ( -14.98890122036483419, -28.67928442680469203, -4.999999999999999112 ) ) ;
#15576=CARTESIAN_POINT ( 'NONE',  ( 15.46723536449282044, -26.71148257425455697, -5.946079193718386335 ) ) ;
#15577=CARTESIAN_POINT ( 'NONE',  ( -22.79932625038946981, -26.94340799757786442, -4.999999999999999112 ) ) ;
#15580=CARTESIAN_POINT ( 'NONE',  ( 11.17038230804670107, 17.76644183184714265, -26.22336807236404610 ) ) ;
#15583=CARTESIAN_POINT ( 'NONE',  ( -14.50510232685715906, -25.43776907747248472, -10.65577769986489542 ) ) ;
#15586=CARTESIAN_POINT ( 'NONE',  ( -29.94129476457376882, -22.05385023193113980, -8.415718586356796038 ) ) ;
#15587=CARTESIAN_POINT ( 'NONE',  ( 1.397217954152080166, -21.66464354399617775, -21.18345308184954590 ) ) ;
#15588=CARTESIAN_POINT ( 'NONE',  ( 15.27813064198010196, 25.57022799658983558, -8.773304169343077774 ) ) ;
#15589=CARTESIAN_POINT ( 'NONE',  ( 20.28966096934918184, 10.25376961063980907, -16.97639449884776752 ) ) ;
#15591=CARTESIAN_POINT ( 'NONE',  ( -4.056756644314476468, 28.55033231052837550, -16.67183270246686178 ) ) ;
#15593=CARTESIAN_POINT ( 'NONE',  ( -32.81213598086766581, -5.178738028136198324, -9.908093442003993445 ) ) ;
#15600=CARTESIAN_POINT ( 'NONE',  ( -20.91237790324122159, 1.319957874075606385, -26.26824219631393476 ) ) ;
#15602=CARTESIAN_POINT ( 'NONE',  ( 27.77279998450218912, -11.16583192376935862, -15.71995317866785946 ) ) ;
#15605=CARTESIAN_POINT ( 'NONE',  ( 19.48557158514982746, -11.25000000000009415, -0.000000000000000000 ) ) ;
#15611=CARTESIAN_POINT ( 'NONE',  ( -2.700909190172711138, 24.47130327029587349, -20.72671218256706993 ) ) ;
#15617=EDGE_CURVE ( 'NONE', #12299, #23375, #39112, .T. ) ;
#15619=CARTESIAN_POINT ( 'NONE',  ( 10.08828624387746586, 22.01629898975007293, -20.18907799365789302 ) ) ;
#15621=CARTESIAN_POINT ( 'NONE',  ( -17.74591135789209773, 10.55662882352565646, -27.17856662802773116 ) ) ;
#15624=CARTESIAN_POINT ( 'NONE',  ( 9.670856713498491075, -18.12756278475329808, -28.70101805749319723 ) ) ;
#15627=CARTESIAN_POINT ( 'NONE',  ( 13.17275120719023107, 22.30352509093737012, -16.43557425179639964 ) ) ;
#15628=CARTESIAN_POINT ( 'NONE',  ( 2.168404344971008868E-14, -26.63027081345975589, -4.999999999999999112 ) ) ;
#15630=CARTESIAN_POINT ( 'NONE',  ( -13.74893865958837580, 23.44248173773514310, -14.47139730366743571 ) ) ;
#15631=CARTESIAN_POINT ( 'NONE',  ( -21.46071079579204977, -24.07222328743980455, -12.13688642999643896 ) ) ;
#15632=CARTESIAN_POINT ( 'NONE',  ( 8.971832194761836021, -22.56238950268238952, -16.70641590008881039 ) ) ;
#15633=CARTESIAN_POINT ( 'NONE',  ( 13.54214413866547240, 22.71670133636794731, -15.45773015834430097 ) ) ;
#15634=CARTESIAN_POINT ( 'NONE',  ( 31.02556648718628196, -22.39342206112319289, -5.000000000000000000 ) ) ;
#15637=CARTESIAN_POINT ( 'NONE',  ( -10.30584816049105257, 34.79301137796964127, -5.444905193120368025 ) ) ;
#15638=DIRECTION ( 'NONE',  ( -0.000000000000000000, -0.000000000000000000, -1.000000000000000000 ) ) ;
#15641=CARTESIAN_POINT ( 'NONE',  ( 18.00000000000000000, 22.50000000000001421, 3.000000000000000000 ) ) ;
#15643=CARTESIAN_POINT ( 'NONE',  ( 20.60885639961789906, 0.8764464790524432170, -28.07880677701691141 ) ) ;
#15648=CARTESIAN_POINT ( 'NONE',  ( -21.27250862215679206, 0.8036217730998547193, -25.01755668826255175 ) ) ;
#15651=CARTESIAN_POINT ( 'NONE',  ( 29.00584441142848746, -5.994069036618491886, -14.94548092090875535 ) ) ;
#15665=CARTESIAN_POINT ( 'NONE',  ( 9.732527571296289537, 33.77328167068598219, -8.933206717022359911 ) ) ;
#15668=CARTESIAN_POINT ( 'NONE',  ( 14.30237662736994508, -22.54417004151479631, -16.27104889190381698 ) ) ;
#15672=CARTESIAN_POINT ( 'NONE',  ( -11.33053354013682856, 18.02203028756851211, -25.01733111074807070 ) ) ;
#15674=CARTESIAN_POINT ( 'NONE',  ( 15.03078399508466134, -26.24871699600646124, -8.298773291112503614 ) ) ;
#15679=CARTESIAN_POINT ( 'NONE',  ( -13.86191765000857856, 30.49075772208747992, -4.999999999999998224 ) ) ;
#15680=CARTESIAN_POINT ( 'NONE',  ( -19.35675346592083557, -25.73740943145480742, -10.41501234748526983 ) ) ;
#15683=CARTESIAN_POINT ( 'NONE',  ( -24.16886640984839119, -7.534202883240132209, -19.77792120075160653 ) ) ;
#15684=CARTESIAN_POINT ( 'NONE',  ( -9.413550212251061922, -18.21086026825004112, -29.35007373650224238 ) ) ;
#15687=CARTESIAN_POINT ( 'NONE',  ( 20.43785338154470921, 1.730618592969307867, -30.00000000000000355 ) ) ;
#15691=CARTESIAN_POINT ( 'NONE',  ( -27.78115282291058818, 0.1336662928856390542, -13.50786979312386471 ) ) ;
#15693=CARTESIAN_POINT ( 'NONE',  ( 24.52549093940175950, -1.059282194882694927, -19.29662230946326673 ) ) ;
#15694=CARTESIAN_POINT ( 'NONE',  ( 17.30788606036681543, -10.99133882972088472, -30.00000000000004263 ) ) ;
#15698=CARTESIAN_POINT ( 'NONE',  ( -25.59020507252603949, 4.375312855643961107, -11.74991072239141765 ) ) ;
#15700=DIRECTION ( 'NONE',  ( -0.000000000000000000, -0.000000000000000000, 1.000000000000000000 ) ) ;
#15705=EDGE_CURVE ( 'NONE', #31788, #21571, #33536, .T. ) ;
#15707=LINE ( 'NONE', #36653, #38516 ) ;
#15709=CARTESIAN_POINT ( 'NONE',  ( -24.15419107429150003, 8.025926297992866054, -6.445781696981516262 ) ) ;
#15712=CARTESIAN_POINT ( 'NONE',  ( 17.38440248539185262, -18.07777754567372952, -19.86656258602833702 ) ) ;
#15714=CARTESIAN_POINT ( 'NONE',  ( 13.08626868863102288, 22.46072230355650845, -16.41598118283816277 ) ) ;
#15716=CARTESIAN_POINT ( 'NONE',  ( -16.00871871683318659, 23.70244287861901356, -8.319657716573615858 ) ) ;
#15722=CARTESIAN_POINT ( 'NONE',  ( 13.78636421790129063, 23.36015420247935737, -14.47817171644321910 ) ) ;
#15724=DIRECTION ( 'NONE',  ( 0.000000000000000000, 0.000000000000000000, 1.000000000000000000 ) ) ;
#15726=CARTESIAN_POINT ( 'NONE',  ( -13.36282164858120147, 23.07485381450693751, -15.42106084104891828 ) ) ;
#15728=CARTESIAN_POINT ( 'NONE',  ( -10.67195756934210316, -19.53628626400035984, -22.71718723575088461 ) ) ;
#15731=CARTESIAN_POINT ( 'NONE',  ( -33.36273675432661179, -16.18931552824140496, -8.847619819632241089 ) ) ;
#15732=CARTESIAN_POINT ( 'NONE',  ( -8.865215912320328684, -18.48469441140770542, -29.36070228624526024 ) ) ;
#15734=CARTESIAN_POINT ( 'NONE',  ( 12.94160102779525445, 16.66888978004905653, -25.21160078660660631 ) ) ;
#15736=CARTESIAN_POINT ( 'NONE',  ( 23.87359454083856747, 4.573863347061236873, -15.74749371091426653 ) ) ;
#15737=CYLINDRICAL_SURFACE ( 'NONE', #16729, 59.99999999999997868 ) ;
#15742=CARTESIAN_POINT ( 'NONE',  ( -29.92778146367382774, -0.3254292208867340386, -10.15219817829411397 ) ) ;
#15743=CARTESIAN_POINT ( 'NONE',  ( 20.53661583307810901, 0.6341784373652767925, -28.69910307870409483 ) ) ;
#15749=CARTESIAN_POINT ( 'NONE',  ( 16.77267017469755217, -29.13948811618736912, -13.79123840944735413 ) ) ;
#15752=CARTESIAN_POINT ( 'NONE',  ( 5.049784273262975631, -26.77689918168219307, -5.000000000000000000 ) ) ;
#15756=CARTESIAN_POINT ( 'NONE',  ( 3.853265673577690009, 37.77810895946699077, -6.702677861497350342 ) ) ;
#15764=CARTESIAN_POINT ( 'NONE',  ( 15.00330998323748055, 28.06465100738194351, -5.468235726354898851 ) ) ;
#15768=CARTESIAN_POINT ( 'NONE',  ( -15.57484573673720796, 13.69435820708697982, -26.56392333108821191 ) ) ;
#15771=CARTESIAN_POINT ( 'NONE',  ( 10.81386370403635944, -19.99604346397223864, -21.62019203441402837 ) ) ;
#15773=CARTESIAN_POINT ( 'NONE',  ( -12.94346141028061759, -16.53452242939091121, -26.54686612419656555 ) ) ;
#15774=CARTESIAN_POINT ( 'NONE',  ( 11.68691289177312420, 18.91070414389390564, -22.73532874761463773 ) ) ;
#15775=CARTESIAN_POINT ( 'NONE',  ( 15.36131648685467610, 26.71043341655636638, -6.416599091998089754 ) ) ;
#15778=CARTESIAN_POINT ( 'NONE',  ( -10.75859123654805316, -20.00912467510691783, -21.62693100897464404 ) ) ;
#15781=CARTESIAN_POINT ( 'NONE',  ( -30.29849476799594044, -22.30624241272796482, -7.553674803089624135 ) ) ;
#15783=CARTESIAN_POINT ( 'NONE',  ( 1.239157320478834423, -20.53705677395570461, -28.86354223400775254 ) ) ;
#15784=CARTESIAN_POINT ( 'NONE',  ( 11.47031954842671730, 17.36846946539129988, -26.86199371866775820 ) ) ;
#15785=CARTESIAN_POINT ( 'NONE',  ( 22.17218238145936837, 9.941665176672954018, -10.87683032894513246 ) ) ;
#15787=VERTEX_POINT ( 'NONE', #20239 ) ;
#15788=CARTESIAN_POINT ( 'NONE',  ( -24.90016405581419434, -2.372344258043737497, -19.14849256580092884 ) ) ;
#15789=CIRCLE ( 'NONE', #35896, 16.00000000000000000 ) ;
#15791=EDGE_LOOP ( 'NONE', ( #19191, #33972, #25257, #37985 ) ) ;
#15795=CARTESIAN_POINT ( 'NONE',  ( -25.62784820657104135, 0.7174978263156285285, -16.47873148568791635 ) ) ;
#15797=CARTESIAN_POINT ( 'NONE',  ( 22.15328883633298318, -8.178027178684930121, -21.92584078457036867 ) ) ;
#15804=B_SPLINE_CURVE_WITH_KNOTS ( 'NONE', 3,
 ( #22903, #7463, #19872, #4424, #4628, #26761 ),
 .UNSPECIFIED., .F., .F.,
 ( 4, 2, 4 ),
 ( 0.000000000000000000, 0.1492836598722001307, 0.2985673197444002613 ),
 .UNSPECIFIED. ) ;
#15811=CARTESIAN_POINT ( 'NONE',  ( -1.699711140334807302, 21.35824065759481627, -25.59207206193138973 ) ) ;
#15816=DIRECTION ( 'NONE',  ( 1.000000000000000000, 0.000000000000000000, 0.000000000000000000 ) ) ;
#15818=CARTESIAN_POINT ( 'NONE',  ( 13.25468081180020263, 29.55206051663221345, -9.525608598956070594 ) ) ;
#15820=CARTESIAN_POINT ( 'NONE',  ( -21.21721043375235283, 12.69857392348516711, -6.454068583460846220 ) ) ;
#15822=CARTESIAN_POINT ( 'NONE',  ( 15.30366455603881803, -26.31361304454697603, -8.292863508495639024 ) ) ;
#15824=CARTESIAN_POINT ( 'NONE',  ( 14.71377148196451934, 25.46827901036206399, -10.64846216776593657 ) ) ;
#15826=CARTESIAN_POINT ( 'NONE',  ( 11.41987377193677489, -19.41918266173338026, -20.90349153980996988 ) ) ;
#15830=CARTESIAN_POINT ( 'NONE',  ( -24.44490540209602614, -24.40828659446678373, -10.25875033300979311 ) ) ;
#15831=CARTESIAN_POINT ( 'NONE',  ( 11.94839969841157590, -24.33362986171098186, -12.62691988318393221 ) ) ;
#15832=CARTESIAN_POINT ( 'NONE',  ( 15.15622143329154525, 25.96001174859074467, -8.769384549947115914 ) ) ;
#15833=CARTESIAN_POINT ( 'NONE',  ( 24.38153214571670446, -17.61758732495730939, -15.69893765422416010 ) ) ;
#15837=CARTESIAN_POINT ( 'NONE',  ( -7.072584127764374173, 21.29840595540943937, -23.29275699177380332 ) ) ;
#15843=CARTESIAN_POINT ( 'NONE',  ( 29.96329728503961221, 0.06029566601255719610, -9.238937171761827827 ) ) ;
#15848=CARTESIAN_POINT ( 'NONE',  ( -30.13613696638300610, 0.06374650685281088580, -8.768336777620580946 ) ) ;
#15852=CARTESIAN_POINT ( 'NONE',  ( 20.29344634343774700, -4.154788219150724160, -27.84155812886654502 ) ) ;
#15864=CARTESIAN_POINT ( 'NONE',  ( -19.71057812522863628, 5.645469553838248444, -29.99999999999999645 ) ) ;
#15867=CARTESIAN_POINT ( 'NONE',  ( 16.01654674860193595, 17.47364687737974975, -16.80141053676624452 ) ) ;
#15868=CARTESIAN_POINT ( 'NONE',  ( 8.811643058094634995, 34.19349861355132703, -9.354887791571313116 ) ) ;
#15869=CARTESIAN_POINT ( 'NONE',  ( 11.31110988152877894, -17.30322875125625615, -27.97697571136258787 ) ) ;
#15870=CYLINDRICAL_SURFACE ( 'NONE', #28803, 57.00000000000003553 ) ;
#15876=CARTESIAN_POINT ( 'NONE',  ( -12.15709906223975700, 19.89297644826506328, -20.54567599615587881 ) ) ;
#15878=CARTESIAN_POINT ( 'NONE',  ( 13.46238087013228579, -24.08803019759326247, -13.52451462657619352 ) ) ;
#15882=CARTESIAN_POINT ( 'NONE',  ( -14.16754981693137339, 28.95138659793071056, -8.202177504148025378 ) ) ;
#15884=CARTESIAN_POINT ( 'NONE',  ( -19.33876548823874231, -27.12358307434724125, -6.816496654975429337 ) ) ;
#15888=CARTESIAN_POINT ( 'NONE',  ( -34.02488686188301159, -10.57580012044028805, -9.338804097880540667 ) ) ;
#15889=CARTESIAN_POINT ( 'NONE',  ( -10.11677155123750005, -19.20203320946534475, -23.86710499911539785 ) ) ;
#15892=CARTESIAN_POINT ( 'NONE',  ( 30.70345270623383627, 0.1631843812369964120, -5.474135951704134584 ) ) ;
#15896=CARTESIAN_POINT ( 'NONE',  ( -30.39538365534349040, -0.04934266608166847090, -8.295282253696063535 ) ) ;
#15898=CARTESIAN_POINT ( 'NONE',  ( 31.65024234132572545, -1.763089522669275322, -8.678469945394718721 ) ) ;
#15899=CARTESIAN_POINT ( 'NONE',  ( -9.819550942989188513, -18.04686579641860078, -30.00000000000000000 ) ) ;
#15903=CARTESIAN_POINT ( 'NONE',  ( -26.55359138347274239, 4.403205473926642632, -8.349092865648199080 ) ) ;
#15904=CARTESIAN_POINT ( 'NONE',  ( -20.66733686379708956, -29.21156249568803531, -4.999999999999997335 ) ) ;
#15909=VECTOR ( 'NONE', #26720, 1000.000000000000000 ) ;
#15910=AXIS2_PLACEMENT_3D ( 'NONE', #4417, #20472, #35905 ) ;
#15914=CARTESIAN_POINT ( 'NONE',  ( -19.48816862725384169, 6.402609444000542993, -29.41693484488668631 ) ) ;
#15916=CARTESIAN_POINT ( 'NONE',  ( 23.69164916738933258, -26.06248331711220345, -8.067269366965431843 ) ) ;
#15918=CARTESIAN_POINT ( 'NONE',  ( 10.86287567075531157, 17.54031720676627515, -28.06684646824993123 ) ) ;
#15920=CARTESIAN_POINT ( 'NONE',  ( -14.28253842008971297, 21.30371530270891256, -15.55968883884288445 ) ) ;
#15924=CARTESIAN_POINT ( 'NONE',  ( 14.76097837988864825, 25.32778234306308462, -10.65473370507753437 ) ) ;
#15929=CARTESIAN_POINT ( 'NONE',  ( -11.58297502488001385, 19.01036633197951176, -22.71718434665674380 ) ) ;
#15931=CARTESIAN_POINT ( 'NONE',  ( -9.708379805665277473, -18.29787746346482891, -27.44150705248273425 ) ) ;
#15934=CARTESIAN_POINT ( 'NONE',  ( -34.37712449666406656, -15.41263033719045339, -7.552124065748168746 ) ) ;
#15935=CARTESIAN_POINT ( 'NONE',  ( -11.23442614370865833, -21.53855194063014267, -18.51691792380379198 ) ) ;
#15937=CARTESIAN_POINT ( 'NONE',  ( 15.29729418701016996, 21.14454537556351355, -13.64836929760071094 ) ) ;
#15939=CARTESIAN_POINT ( 'NONE',  ( 25.09639509413040059, 5.514876398772647903, -10.80109637251452881 ) ) ;
#15941=LINE ( 'NONE', #37674, #36821 ) ;
#15946=CARTESIAN_POINT ( 'NONE',  ( -20.49328727640310888, 0.5260942599782594264, -29.99999999999999645 ) ) ;
#15947=CARTESIAN_POINT ( 'NONE',  ( 21.29626117702810362, 0.6323340879910104295, -24.99883547235564407 ) ) ;
#15952=CARTESIAN_POINT ( 'NONE',  ( -3.859759734048395785E-14, -22.74351282448223799, -21.56489709563626533 ) ) ;
#15960=CARTESIAN_POINT ( 'NONE',  ( 5.015607813569435969, 30.50653394152838516, -14.78114538601825600 ) ) ;
#15967=CARTESIAN_POINT ( 'NONE',  ( 14.59836673145885122, 27.18161558271501832, -9.180379322459677027 ) ) ;
#15971=CARTESIAN_POINT ( 'NONE',  ( -16.12111101626893372, 14.39761757377728912, -22.15277786026702245 ) ) ;
#15976=CARTESIAN_POINT ( 'NONE',  ( 15.10398894348100995, -26.26589654887872527, -8.298239031644310870 ) ) ;
#15978=CARTESIAN_POINT ( 'NONE',  ( 15.42079449665415680, 26.76609254708107244, -5.474200704454040611 ) ) ;
#15979=CARTESIAN_POINT ( 'NONE',  ( 14.83638920640944292, 25.62079248104728535, -10.17951853491134351 ) ) ;
#15982=CARTESIAN_POINT ( 'NONE',  ( -14.63471340173679280, -25.63113514326269993, -10.18257656473890371 ) ) ;
#15984=CARTESIAN_POINT ( 'NONE',  ( -16.53721940376430055, -12.13086247549455443, -29.21783723221567186 ) ) ;
#15985=CARTESIAN_POINT ( 'NONE',  ( -4.434780010005740181, -23.77905508842546922, -12.85394067315957578 ) ) ;
#15986=CARTESIAN_POINT ( 'NONE',  ( 12.01796449282804424, 18.59096114822754231, -22.78820876937768247 ) ) ;
#15989=CARTESIAN_POINT ( 'NONE',  ( 18.25678040558227622, 9.365065964941067023, -28.86123873035057130 ) ) ;
#15994=CARTESIAN_POINT ( 'NONE',  ( -24.21134473998290559, -3.011152994252887627, -20.11598446922123884 ) ) ;
#15999=CARTESIAN_POINT ( 'NONE',  ( -29.21372990917784662, 0.8930521456687262605, -9.252833956221683920 ) ) ;
#16000=CARTESIAN_POINT ( 'NONE',  ( 25.45230351418204151, -11.15605511405185091, -17.62830037521853299 ) ) ;
#16004=EDGE_CURVE ( 'NONE', #19822, #33574, #14706, .T. ) ;
#16011=CARTESIAN_POINT ( 'NONE',  ( -2.776705887744885803, 34.22514237022959804, -11.98289488661590951 ) ) ;
#16017=CARTESIAN_POINT ( 'NONE',  ( 10.12684856687054236, 24.03473075183826069, -18.03693486850220040 ) ) ;
#16019=CARTESIAN_POINT ( 'NONE',  ( -19.94802261067724203, 11.91594554592121114, -14.92335899463314242 ) ) ;
#16021=CARTESIAN_POINT ( 'NONE',  ( 14.40609022250728444, -25.07970014599643349, -11.59567163901805387 ) ) ;
#16023=CARTESIAN_POINT ( 'NONE',  ( 11.85601099147671178, 19.42086764860403036, -21.61009544485835931 ) ) ;
#16024=CARTESIAN_POINT ( 'NONE',  ( 16.77267017469755217, -29.13948811618736912, -13.79123840944735413 ) ) ;
#16028=CARTESIAN_POINT ( 'NONE',  ( -17.82960224414886596, -17.77519942552612520, -19.83192060708631743 ) ) ;
#16029=CARTESIAN_POINT ( 'NONE',  ( 6.772447531124758058, -21.91223081777216564, -18.87814742099377341 ) ) ;
#16030=CARTESIAN_POINT ( 'NONE',  ( 11.44368038160577683, 17.93323933076874255, -25.03240686958881156 ) ) ;
#16031=CARTESIAN_POINT ( 'NONE',  ( 26.97183419387431158, -19.50619947319538383, -12.90440121806097729 ) ) ;
#16035=CARTESIAN_POINT ( 'NONE',  ( -9.049625497917114458, 33.98022236337723712, -9.362205654903002383 ) ) ;
#16039=ORIENTED_EDGE ( 'NONE', *, *, #17261, .T. ) ;
#16040=CARTESIAN_POINT ( 'NONE',  ( 30.52100727590019957, -0.04949924042143036274, -7.826100079217978234 ) ) ;
#16044=CARTESIAN_POINT ( 'NONE',  ( -20.96756735925385229, 0.8276901569395326286, -26.22661741445136840 ) ) ;
#16045=CARTESIAN_POINT ( 'NONE',  ( -17.60052849991877721, -23.51059660139243590, -14.14515744553814258 ) ) ;
#16047=CARTESIAN_POINT ( 'NONE',  ( 34.37689022701968611, -6.182391807707502629, -7.210918363890624683 ) ) ;
#16059=CARTESIAN_POINT ( 'NONE',  ( 9.866575328975670800, 17.98194059978866122, -29.99999999999999645 ) ) ;
#16062=CARTESIAN_POINT ( 'NONE',  ( 17.67500771205885712, 19.99486213594162010, -6.434741731482024996 ) ) ;
#16064=CARTESIAN_POINT ( 'NONE',  ( 9.123773087559795769, 35.63818776545269174, -5.873441756282732129 ) ) ;
#16066=CARTESIAN_POINT ( 'NONE',  ( 16.36351675325202137, -26.72998542747626871, -7.330931130651400451 ) ) ;
#16071=CARTESIAN_POINT ( 'NONE',  ( -14.84491883786760980, 25.59395107166792727, -10.18114221944758135 ) ) ;
#16073=CARTESIAN_POINT ( 'NONE',  ( 11.34245683043676500, -21.00257692745146443, -19.51844232644348764 ) ) ;
#16079=CARTESIAN_POINT ( 'NONE',  ( -12.84571259627460016, 30.17467865810253613, -9.499430740182077670 ) ) ;
#16085=CARTESIAN_POINT ( 'NONE',  ( -35.29093393616297902, -8.784390315875461042, -5.878240462516181708 ) ) ;
#16086=CARTESIAN_POINT ( 'NONE',  ( -11.43337157596636544, -20.99096340568458530, -19.50882303433272469 ) ) ;
#16089=CARTESIAN_POINT ( 'NONE',  ( 23.53087566707228007, 1.464397449701676068, -19.60697909502530223 ) ) ;
#16094=CARTESIAN_POINT ( 'NONE',  ( -30.04181568689138260, -0.02446475513555576228, -9.235284800656327064 ) ) ;
#16096=CARTESIAN_POINT ( 'NONE',  ( 24.40599740997825862, -0.7005350811509940545, -19.34016958161941346 ) ) ;
#16112=CARTESIAN_POINT ( 'NONE',  ( -23.00670302975767001, 8.813160239992733125, -10.36552060695138522 ) ) ;
#16113=CARTESIAN_POINT ( 'NONE',  ( 22.73890499347229266, -26.44294304952364527, -7.647982415843417314 ) ) ;
#16114=VECTOR ( 'NONE', #10455, 1000.000000000000000 ) ;
#16117=CARTESIAN_POINT ( 'NONE',  ( 15.29112707284399697, 26.78136894998224804, -6.884427309518560634 ) ) ;
#16120=CARTESIAN_POINT ( 'NONE',  ( -15.45299194632486817, 25.37713463119194657, -8.304757890177965507 ) ) ;
#16124=CARTESIAN_POINT ( 'NONE',  ( 15.04050438790828359, 25.89781307577547409, -9.239200427050345610 ) ) ;
#16126=CARTESIAN_POINT ( 'NONE',  ( 18.46594824408953883, -9.479048207884551047, -27.70750746852463919 ) ) ;
#16129=CARTESIAN_POINT ( 'NONE',  ( -15.21106512963387480, 26.79959205483123341, -7.350366708388557768 ) ) ;
#16131=CARTESIAN_POINT ( 'NONE',  ( -10.12380078748041967, -18.23434954340907410, -26.79320281504661949 ) ) ;
#16134=CARTESIAN_POINT ( 'NONE',  ( -34.01707189250791430, -16.51593366370477867, -7.547920849479440086 ) ) ;
#16135=CARTESIAN_POINT ( 'NONE',  ( -13.58096217418507834, -25.42507875219865809, -10.20197574081395686 ) ) ;
#16137=CARTESIAN_POINT ( 'NONE',  ( 12.82616162776056257, 17.22787463660536034, -24.04226039045894936 ) ) ;
#16139=CARTESIAN_POINT ( 'NONE',  ( 20.54619531059088189, 5.238262143020175898, -24.25515232715240188 ) ) ;
#16144=CARTESIAN_POINT ( 'NONE',  ( -26.74272548658042936, -0.08550078280221545812, -15.40661396295627661 ) ) ;
#16146=CARTESIAN_POINT ( 'NONE',  ( 31.05663563045704478, -0.3811732190980007817, -6.877908887127494708 ) ) ;
#16150=CIRCLE ( 'NONE', #20048, 17.00000000000000000 ) ;
#16151=CARTESIAN_POINT ( 'NONE',  ( -37.62663912510979003, -8.659558992827880886, -14.26382729546507555 ) ) ;
#16158=CARTESIAN_POINT ( 'NONE',  ( 2.210526487218244185, 21.88195040076548992, -24.24797893842004370 ) ) ;
#16163=CARTESIAN_POINT ( 'NONE',  ( 22.22908212014391793, -18.19034539544399465, -16.69010318239997304 ) ) ;
#16167=AXIS2_PLACEMENT_3D ( 'NONE', #5327, #14677, #33573 ) ;
#16168=CARTESIAN_POINT ( 'NONE',  ( 14.97811516567272250, 26.90743356226946759, -8.273984026653725010 ) ) ;
#16172=CARTESIAN_POINT ( 'NONE',  ( -18.60376045229827824, 17.50160579387829429, -7.896274594234498068 ) ) ;
#16175=CARTESIAN_POINT ( 'NONE',  ( 15.04920134050132319, -26.13886538990421826, -8.767989598681507957 ) ) ;
#16177=CARTESIAN_POINT ( 'NONE',  ( 12.65668697161344980, 21.04834371600279397, -18.45301148604537644 ) ) ;
#16179=CARTESIAN_POINT ( 'NONE',  ( 15.28655252905469730, 26.54335169034005659, -7.357393274253329452 ) ) ;
#16184=CARTESIAN_POINT ( 'NONE',  ( -9.507670998357182768, -18.30485029568063382, -28.08089151536464456 ) ) ;
#16186=CARTESIAN_POINT ( 'NONE',  ( -30.78128484184130187, -22.64136542128004592, -5.436615360335371072 ) ) ;
#16187=CARTESIAN_POINT ( 'NONE',  ( -1.766708854211077595, -20.47917438257665879, -29.42887188877706706 ) ) ;
#16188=CARTESIAN_POINT ( 'NONE',  ( 15.74108267814583506, 25.56877728144000272, -5.946523357311115809 ) ) ;
#16190=CARTESIAN_POINT ( 'NONE',  ( 18.63330078627290831, 8.706250619080577735, -28.29465965160086682 ) ) ;
#16194=CARTESIAN_POINT ( 'NONE',  ( -33.99706561663532511, -4.510256399178081743, -5.454631704968152306 ) ) ;
#16199=CARTESIAN_POINT ( 'NONE',  ( -28.44303449390735494, 1.764778243225489041, -9.267788830656531474 ) ) ;
#16200=CARTESIAN_POINT ( 'NONE',  ( 34.60165783442131726, -15.16164455357073493, -7.126201915243990825 ) ) ;
#16212=CARTESIAN_POINT ( 'NONE',  ( -0.7423364057732033672, 37.73799070049938109, -7.971040485890229732 ) ) ;
#16220=CARTESIAN_POINT ( 'NONE',  ( 13.54008180094028369, 28.15075258002628900, -10.49033432201353477 ) ) ;
#16223=CARTESIAN_POINT ( 'NONE',  ( -18.16760906032456191, 9.915766630534925241, -26.62071025163185212 ) ) ;
#16226=CARTESIAN_POINT ( 'NONE',  ( 9.697117038158115321, -18.30344589899865682, -27.44232109050611612 ) ) ;
#16228=CARTESIAN_POINT ( 'NONE',  ( 15.07355143598519653, 26.23066616942490725, -8.763531730697579292 ) ) ;
#16229=CARTESIAN_POINT ( 'NONE',  ( -7.289639608743034849, -27.06962010326280321, -13.42901749168595060 ) ) ;
#16232=CARTESIAN_POINT ( 'NONE',  ( -19.19123774765981594, -20.32519271048812470, -16.83485235770917043 ) ) ;
#16233=CARTESIAN_POINT ( 'NONE',  ( 5.635282026549600864, -19.76630616200782242, -30.00000000000002132 ) ) ;
#16234=CARTESIAN_POINT ( 'NONE',  ( 12.77347909899223666, 20.87875728061086633, -18.47285699837302886 ) ) ;
#16235=CARTESIAN_POINT ( 'NONE',  ( 26.78380537101320158, -18.14658901527507595, -13.81421069608905050 ) ) ;
#16239=EDGE_CURVE ( 'NONE', #34227, #31250, #23431, .T. ) ;
#16242=CARTESIAN_POINT ( 'NONE',  ( -6.503115034744880063, 27.62047085464899965, -16.75544015141223753 ) ) ;
#16245=CARTESIAN_POINT ( 'NONE',  ( 30.36599317559471345, -0.01867231823262901699, -8.297552807227344118 ) ) ;
#16247=CARTESIAN_POINT ( 'NONE',  ( 0.000000000000000000, 22.50000000000000355, 3.000000000000000000 ) ) ;
#16249=CARTESIAN_POINT ( 'NONE',  ( -29.84897892274408804, 0.1853354081241826434, -9.240966997248238002 ) ) ;
#16251=ORIENTED_EDGE ( 'NONE', *, *, #3166, .F. ) ;
#16252=CARTESIAN_POINT ( 'NONE',  ( 20.15412120921589079, -4.773411862323607480, -27.81894205312340063 ) ) ;
#16262=CARTESIAN_POINT ( 'NONE',  ( -15.94745313500304462, 12.88431841366640640, -30.00000000000001421 ) ) ;
#16266=CARTESIAN_POINT ( 'NONE',  ( 17.27189083593461305, 19.38243549486986694, -10.30461736581324672 ) ) ;
#16267=CARTESIAN_POINT ( 'NONE',  ( 6.781401459173456381, 26.34037369773561821, -17.76491729653662333 ) ) ;
#16269=CARTESIAN_POINT ( 'NONE',  ( 15.73177369934751546, -26.14870740989517728, -9.202792353689568827 ) ) ;
#16273=CARTESIAN_POINT ( 'NONE',  ( -14.74173057345504745, 25.38325330337421448, -10.65401870494813430 ) ) ;
#16276=CARTESIAN_POINT ( 'NONE',  ( 9.892406512096915350, -19.27897539523535286, -23.89377238802892123 ) ) ;
#16281=CARTESIAN_POINT ( 'NONE',  ( -10.62610282291096908, 24.67057416925172575, -17.05606316619996221 ) ) ;
#16282=CARTESIAN_POINT ( 'NONE',  ( -12.53503683000786317, -17.06533638865724711, -25.95590165904247115 ) ) ;
#16284=CARTESIAN_POINT ( 'NONE',  ( -25.26715884121037448, -5.457600878228082486, -18.89157672615069572 ) ) ;
#16287=CARTESIAN_POINT ( 'NONE',  ( 29.23574345009283704, 0.2107415669908022926, -10.65726852293757254 ) ) ;
#16288=CARTESIAN_POINT ( 'NONE',  ( 12.93090914525160429, 21.64873284465707926, -17.43820100234846393 ) ) ;
#16292=CARTESIAN_POINT ( 'NONE',  ( -20.69558676386508722, 0.8167323363481363563, -27.44640420991715146 ) ) ;
#16293=DIRECTION ( 'NONE',  ( 1.000000000000000000, 0.000000000000000000, 0.000000000000000000 ) ) ;
#16295=CARTESIAN_POINT ( 'NONE',  ( 24.07014152680269703, -2.057471556945281943, -20.21244778586666158 ) ) ;
#16312=CARTESIAN_POINT ( 'NONE',  ( -21.42042906878900865, 9.376721029140135499, -14.90424463124249677 ) ) ;
#16313=CARTESIAN_POINT ( 'NONE',  ( 13.93925166872112875, -17.41998327387213763, -23.39582284468144024 ) ) ;
#16316=CARTESIAN_POINT ( 'NONE',  ( 10.96769517727479304, 17.57291733725187299, -27.43959740574487327 ) ) ;
#16318=CARTESIAN_POINT ( 'NONE',  ( -12.01564447343423048, 17.47318069141996233, -25.10589379291032230 ) ) ;
#16321=CARTESIAN_POINT ( 'NONE',  ( 14.30703310639081849, 24.43075738655355522, -12.55189784990152724 ) ) ;
#16322=ORIENTED_EDGE ( 'NONE', *, *, #32198, .T. ) ;
#16323=CARTESIAN_POINT ( 'NONE',  ( 26.88093566382320887, -13.77087523494271792, -15.68169874583660217 ) ) ;
#16324=CARTESIAN_POINT ( 'NONE',  ( 14.98890121934614506, -28.67928442654198307, -0.000000000000000000 ) ) ;
#16327=CARTESIAN_POINT ( 'NONE',  ( -11.00125217484130147, 17.88729467479140567, -26.20505879420463913 ) ) ;
#16330=CARTESIAN_POINT ( 'NONE',  ( -9.820084318045166683, -18.37969044849650757, -26.81932440670792062 ) ) ;
#16335=CARTESIAN_POINT ( 'NONE',  ( -32.45949353565496409, -15.74491919779192806, -10.17783366908536813 ) ) ;
#16336=CARTESIAN_POINT ( 'NONE',  ( -14.22070947177296851, -26.40434344209961637, -5.946558550297234902 ) ) ;
#16337=CARTESIAN_POINT ( 'NONE',  ( 3.863783140547853712E-14, -86.77689918168233874, 0.000000000000000000 ) ) ;
#16338=CARTESIAN_POINT ( 'NONE',  ( 16.49060731112116684, 23.31193391774742807, -5.474701027004573284 ) ) ;
#16340=CARTESIAN_POINT ( 'NONE',  ( 27.23700843456267151, 3.778717822207238175, -7.382781898693922429 ) ) ;
#16344=CARTESIAN_POINT ( 'NONE',  ( -23.44040957046583173, 0.2069204251881845147, -20.49466620512498238 ) ) ;
#16345=CARTESIAN_POINT ( 'NONE',  ( 27.32033147505850224, -0.01464922774640640794, -14.44792093758196749 ) ) ;
#16349=CARTESIAN_POINT ( 'NONE',  ( 11.41987377193677489, -19.41918266173338026, -20.90349153980996988 ) ) ;
#16363=CARTESIAN_POINT ( 'NONE',  ( 23.96003644509144337, -20.87731938338408000, -13.86997135298250505 ) ) ;
#16366=CARTESIAN_POINT ( 'NONE',  ( 14.73628306789068887, 26.39990037738499851, -9.676459069332137730 ) ) ;
#16369=CARTESIAN_POINT ( 'NONE',  ( -15.13822083024485465, 15.68883449183921108, -22.06930914276376399 ) ) ;
#16373=CARTESIAN_POINT ( 'NONE',  ( 14.83864103363871934, -25.82583482475954995, -9.709532566869290449 ) ) ;
#16375=CARTESIAN_POINT ( 'NONE',  ( 15.40441473722033372, 26.73208805529019827, -5.946081656235632451 ) ) ;
#16377=CARTESIAN_POINT ( 'NONE',  ( 14.53140152873310775, 24.97328356840171182, -11.59890379914568115 ) ) ;
#16379=CARTESIAN_POINT ( 'NONE',  ( -13.98917752177664475, 24.03416810030780937, -13.50391462411186438 ) ) ;
#16381=CARTESIAN_POINT ( 'NONE',  ( -10.52525848093844196, -19.57894633451951805, -22.73643589974196999 ) ) ;
#16383=ADVANCED_FACE ( 'NONE', ( #24029 ), #36424, .F. ) ;
#16385=CARTESIAN_POINT ( 'NONE',  ( -30.57778148685732944, -22.50129585022499867, -6.703186603742934402 ) ) ;
#16386=CARTESIAN_POINT ( 'NONE',  ( -4.617270946191116998, -24.33986194121566271, -10.36143787604604682 ) ) ;
#16387=CARTESIAN_POINT ( 'NONE',  ( 15.52679059097398273, 25.14300703315133134, -8.306665296563053857 ) ) ;
#16389=CARTESIAN_POINT ( 'NONE',  ( 21.94669886647698220, 10.98376864938533082, -8.898427312023766689 ) ) ;
#16393=CARTESIAN_POINT ( 'NONE',  ( -21.45859226520986951, -2.583396648404852503, -24.66285604314880686 ) ) ;
#16396=DIRECTION ( 'NONE',  ( -1.000000000000000000, 0.000000000000000000, 0.000000000000000000 ) ) ;
#16397=DIRECTION ( 'NONE',  ( 1.000000000000000000, 0.000000000000000000, -0.000000000000000000 ) ) ;
#16398=CARTESIAN_POINT ( 'NONE',  ( 19.09187170439694725, -7.719518535268413473, -28.46272815273926682 ) ) ;
#16405=CARTESIAN_POINT ( 'NONE',  ( -19.07667540522614047, 16.81475038866948069, -5.000000000000000000 ) ) ;
#16409=CARTESIAN_POINT ( 'NONE',  ( -0.4436405235953277959, 22.83777681550889582, -22.98300611285952755 ) ) ;
#16416=CARTESIAN_POINT ( 'NONE',  ( 14.16561412993485014, 28.57187406534849927, -8.667803205440176129 ) ) ;
#16419=CARTESIAN_POINT ( 'NONE',  ( -18.58854498669193944, 12.12440799916769940, -19.06110518814004706 ) ) ;
#16422=CARTESIAN_POINT ( 'NONE',  ( 15.37591282558991601, -26.51818385147999635, -7.356517339422841140 ) ) ;
#16424=CARTESIAN_POINT ( 'NONE',  ( 15.39755691330850951, 26.84919286949167017, -5.473884989333777540 ) ) ;
#16425=CARTESIAN_POINT ( 'NONE',  ( 6.023418944065110914, 39.81932404830325112, -14.45070082761206365 ) ) ;
#16428=CARTESIAN_POINT ( 'NONE',  ( -16.56729576810697324, -17.53405923247618858, -20.95322699904796693 ) ) ;
#16429=CARTESIAN_POINT ( 'NONE',  ( 8.251618643569010203, -24.83515768495495379, -9.332969128487192734 ) ) ;
#16430=CARTESIAN_POINT ( 'NONE',  ( 15.00280477620397512, 25.59022088404001138, -9.712201262136385793 ) ) ;
#16431=CARTESIAN_POINT ( 'NONE',  ( 29.94381607632180220, -21.64440053025225552, -8.853049120304181230 ) ) ;
#16437=CARTESIAN_POINT ( 'NONE',  ( -5.802259185096063199, 21.80286457058984340, -23.19183301011633347 ) ) ;
#16441=CARTESIAN_POINT ( 'NONE',  ( 21.28174780547579914, 0.7376432744340452041, -25.01040352120890020 ) ) ;
#16447=CARTESIAN_POINT ( 'NONE',  ( -30.75812384186223625, 0.07155913731190695348, -5.946101298864587825 ) ) ;
#16448=CARTESIAN_POINT ( 'NONE',  ( -19.54254079969926750, -25.96847085201792282, -9.956545144438887718 ) ) ;
#16450=ORIENTED_EDGE ( 'NONE', *, *, #34335, .T. ) ;
#16451=CARTESIAN_POINT ( 'NONE',  ( 34.72648361517081383, -9.366762812312714459, -8.036555274816278072 ) ) ;
#16463=CARTESIAN_POINT ( 'NONE',  ( -11.90291963069949155, 16.69351461089588540, -29.99999999999999289 ) ) ;
#16468=CARTESIAN_POINT ( 'NONE',  ( 16.70512624272670976, 16.98008137324713118, -15.81966299108973573 ) ) ;
#16469=CARTESIAN_POINT ( 'NONE',  ( 7.632467833249850564, 23.73579192844700714, -19.92015518565826326 ) ) ;
#16473=CARTESIAN_POINT ( 'NONE',  ( 12.28607510256881241, -20.87432611439488639, -19.40397933997828872 ) ) ;
#16477=CARTESIAN_POINT ( 'NONE',  ( -13.22195404768716642, 22.21339375608201294, -16.44601427550475847 ) ) ;
#16480=CARTESIAN_POINT ( 'NONE',  ( 13.33431249370194926, -24.07337194581927164, -13.53033386366181468 ) ) ;
#16484=CARTESIAN_POINT ( 'NONE',  ( -12.64192529757091954, 32.30851842349025560, -5.897544463971819084 ) ) ;
#16489=CARTESIAN_POINT ( 'NONE',  ( -20.11683937074663930, -4.305318936261572915, -28.53642093606467967 ) ) ;
#16493=CARTESIAN_POINT ( 'NONE',  ( 29.67767680329217939, 0.1815030806635676563, -9.711878978317606936 ) ) ;
#16494=CARTESIAN_POINT ( 'NONE',  ( 15.41558956984165363, 26.78481017248027740, -5.000000000000000000 ) ) ;
#16498=CARTESIAN_POINT ( 'NONE',  ( -20.69415337481283501, 0.8377244533787358005, -27.44776534124708434 ) ) ;
#16501=CARTESIAN_POINT ( 'NONE',  ( 25.36917227601168889, -1.505153948585238322, -18.21253142723226759 ) ) ;
#16518=CARTESIAN_POINT ( 'NONE',  ( -23.46155114344813342, 8.928999627652238757, -7.419147749525820679 ) ) ;
#16519=CARTESIAN_POINT ( 'NONE',  ( 17.65433335263828596, -21.92020081565964418, -16.00066446180797186 ) ) ;
#16521=CARTESIAN_POINT ( 'NONE',  ( 15.36061443993781062, 26.97785078317152596, -5.473250886727928588 ) ) ;
#16524=CARTESIAN_POINT ( 'NONE',  ( -15.84332410282777559, 25.22439668510312316, -5.946718473460527399 ) ) ;
#16527=CARTESIAN_POINT ( 'NONE',  ( 15.44688523099049959, 26.67261462138580441, -5.474175438101869240 ) ) ;
#16529=CARTESIAN_POINT ( 'NONE',  ( 30.67527980673472143, -15.70519271476555190, -11.97612696850552716 ) ) ;
#16532=CARTESIAN_POINT ( 'NONE',  ( -10.81748158546086280, 17.46796835832452288, -28.69910257507550000 ) ) ;
#16534=CARTESIAN_POINT ( 'NONE',  ( -16.41154929109325877, -26.54183177608878808, -8.252701314873407412 ) ) ;
#16535=EDGE_CURVE ( 'NONE', #20904, #1089, #39375, .T. ) ;
#16538=CARTESIAN_POINT ( 'NONE',  ( -19.01480660951762403, -7.883819887955906935, -28.46126324442468558 ) ) ;
#16539=CARTESIAN_POINT ( 'NONE',  ( -13.86090271882461522, -25.47782269314085823, -10.19673432174426786 ) ) ;
#16541=CARTESIAN_POINT ( 'NONE',  ( 12.66487866387964978, 16.11973886863585648, -29.38096022884959879 ) ) ;
#16543=CARTESIAN_POINT ( 'NONE',  ( 21.35709708808257901, 3.778198925977738210, -23.05548261300866741 ) ) ;
#16548=CARTESIAN_POINT ( 'NONE',  ( -28.56343558534357996, -0.1369546348107109623, -12.52232705135813262 ) ) ;
#16550=CARTESIAN_POINT ( 'NONE',  ( 31.48691846961225593, -0.7858779617076784296, -6.401761492272640908 ) ) ;
#16554=CARTESIAN_POINT ( 'NONE',  ( -20.90924525106831666, -8.502318254486386451, -19.80438750953543803 ) ) ;
#16562=DIRECTION ( 'NONE',  ( 0.000000000000000000, 0.000000000000000000, -1.000000000000000000 ) ) ;
#16567=CARTESIAN_POINT ( 'NONE',  ( 27.13643189954879631, -23.62865347416715522, -9.322685417528527196 ) ) ;
#16572=CARTESIAN_POINT ( 'NONE',  ( 13.24833755792088397, 23.29711900540358016, -15.39597941112752899 ) ) ;
#16575=CARTESIAN_POINT ( 'NONE',  ( -17.39674132288666897, 19.08569459991767658, -10.31070539419228993 ) ) ;
#16577=CARTESIAN_POINT ( 'NONE',  ( 12.26911082574471479, -22.02329771041612716, -17.43940135948574621 ) ) ;
#16579=CARTESIAN_POINT ( 'NONE',  ( 11.18323034263226035, 17.75715498309750728, -26.22476241273409059 ) ) ;
#16581=CARTESIAN_POINT ( 'NONE',  ( 11.03438618020454065, 17.42870394567875181, -28.07707603705586052 ) ) ;
#16584=CARTESIAN_POINT ( 'NONE',  ( -10.95814459664155294, 17.32538844660855659, -29.34778725072792938 ) ) ;
#16586=CARTESIAN_POINT ( 'NONE',  ( -13.37288965632171056, -23.62230190449336931, -14.47666671991737708 ) ) ;
#16589=CARTESIAN_POINT ( 'NONE',  ( -17.09558480960348703, -11.76928779124230928, -27.71295030018220018 ) ) ;
#16590=CARTESIAN_POINT ( 'NONE',  ( -7.011761754585625006, -25.08926108585034243, -6.920918333007429091 ) ) ;
#16591=CARTESIAN_POINT ( 'NONE',  ( 15.45857095869342146, 25.00809084266443350, -8.779209621340882563 ) ) ;
#16594=CARTESIAN_POINT ( 'NONE',  ( 19.41139689652032274, 8.139058158844877156, -24.38516366816878289 ) ) ;
#16595=DIRECTION ( 'NONE',  ( 0.000000000000000000, 0.000000000000000000, 1.000000000000000000 ) ) ;
#16596=DIRECTION ( 'NONE',  ( -0.000000000000000000, -0.000000000000000000, -1.000000000000000000 ) ) ;
#16599=CARTESIAN_POINT ( 'NONE',  ( -25.03457601920170106, -3.132625777938056633, -19.07791454636011252 ) ) ;
#16605=CARTESIAN_POINT ( 'NONE',  ( 33.21478130368457471, -15.74274012923293498, -9.287806114988983452 ) ) ;
#16610=AXIS2_PLACEMENT_3D ( 'NONE', #33437, #17990, #30378 ) ;
#16618=CARTESIAN_POINT ( 'NONE',  ( -0.3972110264143895453, 20.50537081352338475, -29.21185317353639022 ) ) ;
#16625=CARTESIAN_POINT ( 'NONE',  ( 14.29899370898130506, 28.88346223184144890, -7.751924271491758667 ) ) ;
#16628=CARTESIAN_POINT ( 'NONE',  ( -19.02631976647747436, 12.44553799571251851, -16.97951980596597821 ) ) ;
#16631=CARTESIAN_POINT ( 'NONE',  ( 10.04937125551628618, -18.78011654068590630, -25.00484559559975395 ) ) ;
#16633=CARTESIAN_POINT ( 'NONE',  ( 15.21849957777671314, 26.45364063945018174, -7.826203491635935094 ) ) ;
#16634=CARTESIAN_POINT ( 'NONE',  ( -37.49625565938783467, -14.69322820095472792, -14.45070082761207964 ) ) ;
#16637=CARTESIAN_POINT ( 'NONE',  ( -18.30114940672576296, -16.17431463582818552, -20.81536956475945743 ) ) ;
#16638=CARTESIAN_POINT ( 'NONE',  ( 5.525540643850987088, -23.27048628860477208, -14.83466894819389559 ) ) ;
#16639=CARTESIAN_POINT ( 'NONE',  ( 14.36253475959486536, 24.29084598106111059, -12.55734418687435472 ) ) ;
#16641=CARTESIAN_POINT ( 'NONE',  ( 19.39710119862932558, 14.36785624656014271, -11.87024744276765809 ) ) ;
#16645=CARTESIAN_POINT ( 'NONE',  ( -7.519639825678971157, 28.17713263649764244, -15.83309228201346741 ) ) ;
#16650=CARTESIAN_POINT ( 'NONE',  ( 30.63487244704973733, -0.03777629022359453581, -7.357755587464951397 ) ) ;
#16654=CARTESIAN_POINT ( 'NONE',  ( -25.77377119570790143, 0.4699378652983322580, -16.45710013214238288 ) ) ;
#16656=CARTESIAN_POINT ( 'NONE',  ( 29.08655274285753833, -6.911406729420680684, -14.90707277284040977 ) ) ;
#16663=DIRECTION ( 'NONE',  ( 1.000000000000000000, 0.000000000000000000, 0.000000000000000000 ) ) ;
#16671=CARTESIAN_POINT ( 'NONE',  ( 17.61609821162914713, 19.90481306378846682, -7.394926759373131375 ) ) ;
#16673=CARTESIAN_POINT ( 'NONE',  ( 6.371632084311922739, 19.71237340112613268, -27.83441168883466688 ) ) ;
#16678=CARTESIAN_POINT ( 'NONE',  ( 10.87541234147110636, -18.92597107710026449, -23.77079982040127248 ) ) ;
#16680=DIRECTION ( 'NONE',  ( 1.000000000000000000, 0.000000000000000000, 0.000000000000000000 ) ) ;
#16682=CARTESIAN_POINT ( 'NONE',  ( -14.29267867992720298, 24.46646551869955388, -12.55102490079049282 ) ) ;
#16684=CARTESIAN_POINT ( 'NONE',  ( 14.59266630479183036, -26.14775508231291923, -8.302069403805344194 ) ) ;
#16687=VERTEX_POINT ( 'NONE', #23532 ) ;
#16688=CARTESIAN_POINT ( 'NONE',  ( -13.08275260916906113, 30.80677173799382018, -8.144048944713123461 ) ) ;
#16691=CARTESIAN_POINT ( 'NONE',  ( -23.45153049914467047, -5.794994276869281258, -20.93761132930348268 ) ) ;
#16693=EDGE_LOOP ( 'NONE', ( #18533, #37783, #3422, #36973 ) ) ;
#16694=CARTESIAN_POINT ( 'NONE',  ( 20.47484565207173546, 1.015995796922180006, -29.35120656865814937 ) ) ;
#16699=CARTESIAN_POINT ( 'NONE',  ( -30.61903234434311827, -0.02130004668534590459, -7.357831981613901284 ) ) ;
#16702=CARTESIAN_POINT ( 'NONE',  ( 20.61746273054656342, -1.604345479211515491, -27.95458587662992400 ) ) ;
#16718=ADVANCED_FACE ( 'NONE', ( #4442 ), #19473, .T. ) ;
#16720=CARTESIAN_POINT ( 'NONE',  ( -19.17173663826903862, 7.846818401146893329, -26.59525583229557810 ) ) ;
#16722=CARTESIAN_POINT ( 'NONE',  ( 20.67276675977905498, -26.96143717380833849, -7.241510599420801775 ) ) ;
#16725=CARTESIAN_POINT ( 'NONE',  ( 15.28171370150459829, 26.81318960135283902, -6.883740541788177403 ) ) ;
#16728=CARTESIAN_POINT ( 'NONE',  ( -11.84261757144468596, 17.09703652377666927, -26.89487436953058008 ) ) ;
#16729=AXIS2_PLACEMENT_3D ( 'NONE', #9052, #40116, #12293 ) ;
#16732=CARTESIAN_POINT ( 'NONE',  ( 11.23528749269386395, 17.71942187280074421, -26.23031324771008244 ) ) ;
#16734=CARTESIAN_POINT ( 'NONE',  ( 27.44116408010769703, -15.12913582886689134, -14.73136720375602415 ) ) ;
#16738=CARTESIAN_POINT ( 'NONE',  ( -15.23746052738172096, 27.38211562678985445, -5.000000000000001776 ) ) ;
#16740=CARTESIAN_POINT ( 'NONE',  ( -16.15831973348936401, -26.82997807573334725, -6.405446087739315786 ) ) ;
#16744=CARTESIAN_POINT ( 'NONE',  ( -18.70070976566389831, -8.421454915599365876, -30.00000000000000711 ) ) ;
#16745=CARTESIAN_POINT ( 'NONE',  ( -12.96835034737378045, -23.58818813561633831, -14.49844098154287053 ) ) ;
#16747=CARTESIAN_POINT ( 'NONE',  ( 17.09040934979314841, 20.79557903151203746, -8.349269920398814548 ) ) ;
#16749=CARTESIAN_POINT ( 'NONE',  ( 20.78981288118261261, 4.511901260326916407, -24.21075109639451384 ) ) ;
#16755=CARTESIAN_POINT ( 'NONE',  ( -24.04802182397615340, 0.2326015010894557367, -19.46165338998660133 ) ) ;
#16756=CARTESIAN_POINT ( 'NONE',  ( 20.49706908807578287, 0.3883427504116042650, -30.00000000000000355 ) ) ;
#16759=CARTESIAN_POINT ( 'NONE',  ( 6.155076441694338207, 21.71698211341367113, -30.00000000000000000 ) ) ;
#16761=AXIS2_PLACEMENT_3D ( 'NONE', #39178, #26589, #17056 ) ;
#16764=CARTESIAN_POINT ( 'NONE',  ( -30.90412082983252873, -0.04211290444285954726, 0.000000000000000000 ) ) ;
#16765=AXIS2_PLACEMENT_3D ( 'NONE', #15605, #37140, #18853 ) ;
#16773=CARTESIAN_POINT ( 'NONE',  ( 24.52772961496341608, -22.70861085562849624, -12.04500047335969271 ) ) ;
#16776=CARTESIAN_POINT ( 'NONE',  ( 13.48825381686340741, 24.00059731804531538, -14.41398086289930269 ) ) ;
#16779=CARTESIAN_POINT ( 'NONE',  ( -16.15633541497567194, 17.24146705615139652, -16.81735594647537013 ) ) ;
#16781=CARTESIAN_POINT ( 'NONE',  ( 14.25957742305259046, -25.05340746124562301, -11.60179240159362912 ) ) ;
#16782=DIRECTION ( 'NONE',  ( 0.000000000000000000, 0.000000000000000000, 1.000000000000000000 ) ) ;
#16783=CARTESIAN_POINT ( 'NONE',  ( 11.01382701200410352, 17.34314758767475695, -28.70727912091412293 ) ) ;
#16785=CARTESIAN_POINT ( 'NONE',  ( 12.92727378465670895, 21.65459399332963386, -17.43760083564437124 ) ) ;
#16787=CARTESIAN_POINT ( 'NONE',  ( -14.90130370912292967, 25.90675389883749347, -9.703026954905764612 ) ) ;
#16789=CARTESIAN_POINT ( 'NONE',  ( -14.00737455831331069, -24.60610348959216864, -12.55177947858446785 ) ) ;
#16793=CARTESIAN_POINT ( 'NONE',  ( -17.22654052972206173, -11.11309616262812838, -30.00000000000001421 ) ) ;
#16794=CARTESIAN_POINT ( 'NONE',  ( -1.866162468650815365, -20.97895390888915301, -24.40979417473883473 ) ) ;
#16795=CARTESIAN_POINT ( 'NONE',  ( 15.30672036741259490, 24.25326656399939296, -10.20631967863550749 ) ) ;
#16797=CARTESIAN_POINT ( 'NONE',  ( 23.15824302559796521, 9.164155139735443711, -8.398248912862177562 ) ) ;
#16798=CARTESIAN_POINT ( 'NONE',  ( 28.32385402320780798, -24.64261966148930583, -4.999999999999998224 ) ) ;
#16799=CARTESIAN_POINT ( 'NONE',  ( 2.510240364580639039, -24.77672057670806183, -5.000000000000004441 ) ) ;
#16804=CARTESIAN_POINT ( 'NONE',  ( -31.17348492595634113, -2.327576281512217626, -10.48814752622052104 ) ) ;
#16808=DIRECTION ( 'NONE',  ( -0.000000000000000000, -0.000000000000000000, -1.000000000000000000 ) ) ;
#16810=CARTESIAN_POINT ( 'NONE',  ( 34.95664498758854677, -15.33017443246186495, -4.999999999999996447 ) ) ;
#16814=CARTESIAN_POINT ( 'NONE',  ( -15.43632923247374755, 26.71034459555102103, -5.000000000000004441 ) ) ;
#16816=VECTOR ( 'NONE', #14581, 1000.000000000000000 ) ;
#16820=CARTESIAN_POINT ( 'NONE',  ( -1.871070526050384597, 37.10316175800964800, -8.844908016778285642 ) ) ;
#16828=CARTESIAN_POINT ( 'NONE',  ( 14.18620732935935003, 29.69268515973297440, -6.373436630974609329 ) ) ;
#16832=CARTESIAN_POINT ( 'NONE',  ( -20.14604714284210729, 14.61654826405655072, -6.936879617510046891 ) ) ;
#16835=CARTESIAN_POINT ( 'NONE',  ( 15.53709981414127483, -26.75515487142352100, -5.473964991478021069 ) ) ;
#16837=CARTESIAN_POINT ( 'NONE',  ( 11.27293877700655678, 18.06695805791709830, -25.00947300646876670 ) ) ;
#16838=CARTESIAN_POINT ( 'NONE',  ( -20.90924525106831666, -8.502318254486386451, -30.00000000000000711 ) ) ;
#16840=CARTESIAN_POINT ( 'NONE',  ( -25.39332128722019988, -23.88597321859529288, -10.24008034875545370 ) ) ;
#16841=CARTESIAN_POINT ( 'NONE',  ( 6.121139850082340850, -20.67279834681676576, -23.15975327329053002 ) ) ;
#16842=CARTESIAN_POINT ( 'NONE',  ( 15.45245795801566935, 26.38988594971563728, -6.417325671787477148 ) ) ;
#16843=CARTESIAN_POINT ( 'NONE',  ( 17.10314071577965933, 11.30215440122589499, -29.42840768176305133 ) ) ;
#16848=CARTESIAN_POINT ( 'NONE',  ( -5.336011467082187210, 20.01953256073105081, -27.79733467733078456 ) ) ;
#16851=CARTESIAN_POINT ( 'NONE',  ( -11.78982961964231535, -21.49398613183140228, -18.46362487464430302 ) ) ;
#16856=CARTESIAN_POINT ( 'NONE',  ( 26.53299061067440334, 0.2339631145021888736, -15.44550104827009740 ) ) ;
#16861=CARTESIAN_POINT ( 'NONE',  ( -30.08539553338631123, 0.1183567654270563652, -8.769032276601203435 ) ) ;
#16863=CARTESIAN_POINT ( 'NONE',  ( 20.28784519644407425, -4.806164102564737028, -27.11309778525960468 ) ) ;
#16868=EDGE_CURVE ( 'NONE', #29585, #17337, #17857, .T. ) ;
#16873=( NAMED_UNIT ( * ) PLANE_ANGLE_UNIT ( ) SI_UNIT ( $, .RADIAN. ) );
#16874=CARTESIAN_POINT ( 'NONE',  ( -17.09830543661136559, -11.32827756084940951, -30.00000000000001776 ) ) ;
#16877=CARTESIAN_POINT ( 'NONE',  ( 18.89396845472720088, 16.74745873269439400, -8.388403218796401717 ) ) ;
#16878=CARTESIAN_POINT ( 'NONE',  ( 9.653912746977081127, 30.01279398118651542, -13.05665368966775475 ) ) ;
#16883=CARTESIAN_POINT ( 'NONE',  ( 10.59539299448435479, -18.54736905940730551, -24.94025571391961194 ) ) ;
#16888=CARTESIAN_POINT ( 'NONE',  ( -11.04584868602368353, 17.42116418599707117, -28.07775973395273539 ) ) ;
#16890=CARTESIAN_POINT ( 'NONE',  ( 9.384463268206888031, -18.58243950274592393, -26.85571026258529059 ) ) ;
#16894=CARTESIAN_POINT ( 'NONE',  ( -11.17084153242268485, 24.05774765238854940, -17.12906072756529596 ) ) ;
#16895=CARTESIAN_POINT ( 'NONE',  ( -17.08966009880722936, -22.85233454443725165, -15.10154554499656854 ) ) ;
#16898=CARTESIAN_POINT ( 'NONE',  ( -21.87366440923314315, -5.401708001756898803, -23.22369624925320508 ) ) ;
#16901=CARTESIAN_POINT ( 'NONE',  ( 28.72940827134124575, 0.2944283357868948681, -11.60603752271954292 ) ) ;
#16906=CARTESIAN_POINT ( 'NONE',  ( -23.32189782144615009, 0.5388808099659079254, -20.54027897587359064 ) ) ;
#16909=CARTESIAN_POINT ( 'NONE',  ( 22.68321730624148813, -1.879180904300666199, -22.42295850830599235 ) ) ;
#16920=CARTESIAN_POINT ( 'NONE',  ( 5.831757820639368539, 35.44601310684239337, -9.755031229041589924 ) ) ;
#16924=CARTESIAN_POINT ( 'NONE',  ( -18.40039352423243457, 9.187127761490295086, -28.29769893192780827 ) ) ;
#16925=CARTESIAN_POINT ( 'NONE',  ( 20.17145048931689644, -26.36706761496765949, -9.037115501373188309 ) ) ;
#16928=EDGE_LOOP ( 'NONE', ( #38571, #6585, #15296, #38105 ) ) ;
#16929=CARTESIAN_POINT ( 'NONE',  ( 11.03496570447431147, 17.67526184817850066, -26.82193291291117276 ) ) ;
#16931=CARTESIAN_POINT ( 'NONE',  ( -13.28422579199402520, 19.31593456181959212, -19.64488464522398203 ) ) ;
#16933=FACE_OUTER_BOUND ( 'NONE', #20570, .T. ) ;
#16934=CARTESIAN_POINT ( 'NONE',  ( 11.09155550310888394, 17.39098317871841459, -28.08047184062978374 ) ) ;
#16936=CARTESIAN_POINT ( 'NONE',  ( 18.32281867441876599, -9.405883636210713661, -28.44593439518221345 ) ) ;
#16939=CARTESIAN_POINT ( 'NONE',  ( -14.38234336660450019, 25.38722357239544891, -11.56793431969083130 ) ) ;
#16941=CARTESIAN_POINT ( 'NONE',  ( -10.22076385035975932, -18.36610753837789289, -26.18274680826524303 ) ) ;
#16944=CARTESIAN_POINT ( 'NONE',  ( -23.64546601257486103, -9.782033131034459927, -19.68101090808202613 ) ) ;
#16945=CARTESIAN_POINT ( 'NONE',  ( -13.77000343459438803, -24.97058995738720455, -11.61570562419389141 ) ) ;
#16947=CARTESIAN_POINT ( 'NONE',  ( 16.72342278700635987, 21.93126413797296692, -7.859335597179046395 ) ) ;
#16948=VERTEX_POINT ( 'NONE', #12144 ) ;
#16949=CARTESIAN_POINT ( 'NONE',  ( 24.35141779062506018, 2.949667068470618325, -16.65809308903522634 ) ) ;
#16954=CARTESIAN_POINT ( 'NONE',  ( -20.53768214670897407, 0.6048634969346144974, -28.69806880511274016 ) ) ;
#16955=CARTESIAN_POINT ( 'NONE',  ( 31.60127994866165224, -0.7964638025070724936, -5.469550557027236692 ) ) ;
#16961=CARTESIAN_POINT ( 'NONE',  ( -20.56897251348186728, 2.201150519725052046, -27.52994173289911473 ) ) ;
#16963=CARTESIAN_POINT ( 'NONE',  ( -30.41237130417910706, 3.314011747244090422, -13.58461195433496371 ) ) ;
#16974=CARTESIAN_POINT ( 'NONE',  ( 27.36121244743086578, -25.22392150776288133, -4.999999999999999112 ) ) ;
#16977=CARTESIAN_POINT ( 'NONE',  ( 10.65171411591334127, 17.77866102667491788, -27.41507814813356347 ) ) ;
#16981=CARTESIAN_POINT ( 'NONE',  ( -17.26788437172030299, 20.57138498279865857, -7.871131841751277669 ) ) ;
#16984=CARTESIAN_POINT ( 'NONE',  ( 14.87191199626541582, -25.96639945386176151, -9.239640580059129249 ) ) ;
#16986=CARTESIAN_POINT ( 'NONE',  ( 15.34748833658096956, 26.58512746428727525, -6.887971585101123395 ) ) ;
#16988=CARTESIAN_POINT ( 'NONE',  ( 11.17889170011724254, 17.76029153187228005, -26.22429826898334326 ) ) ;
#16990=CARTESIAN_POINT ( 'NONE',  ( -15.37572116813434775, 26.83420713582532002, -5.945198187637174669 ) ) ;
#16991=CARTESIAN_POINT ( 'NONE',  ( 36.48557158514975640, -11.24999999999995559, 10.00000000000000000 ) ) ;
#16992=CARTESIAN_POINT ( 'NONE',  ( -9.564252382813446474, -18.27657358539217825, -28.07775981309165658 ) ) ;
#16994=CARTESIAN_POINT ( 'NONE',  ( -16.89362134160771944, -11.62925611732713804, -29.21493252340928848 ) ) ;
#16995=CARTESIAN_POINT ( 'NONE',  ( -6.662515794070015041, -20.56860814960122852, -23.12314935263888316 ) ) ;
#16996=CARTESIAN_POINT ( 'NONE',  ( 15.47267297930532592, 24.57749586628517235, -9.256576209186675896 ) ) ;
#16998=CARTESIAN_POINT ( 'NONE',  ( 21.96684812253698738, 7.874168224664914284, -15.89034991468182412 ) ) ;
#17004=CARTESIAN_POINT ( 'NONE',  ( -26.65769201652798870, -1.128111410740069376, -16.27386567072153412 ) ) ;
#17009=DIRECTION ( 'NONE',  ( 1.000000000000000000, 0.000000000000000000, 0.000000000000000000 ) ) ;
#17012=CARTESIAN_POINT ( 'NONE',  ( 19.09512323183120941, -9.087989146580193633, -26.26778683489222033 ) ) ;
#17018=DIRECTION ( 'NONE',  ( 0.000000000000000000, 0.000000000000000000, -1.000000000000000000 ) ) ;
#17019=CARTESIAN_POINT ( 'NONE',  ( -0.5717484631679848883, 29.10109329946823209, -16.62448788259939647 ) ) ;
#17028=CARTESIAN_POINT ( 'NONE',  ( 13.89517812676522190, 27.95167899239444154, -10.04991680958497291 ) ) ;
#17032=CARTESIAN_POINT ( 'NONE',  ( -20.04575374383065878, 13.19209304670532568, -11.88046426404956257 ) ) ;
#17035=CARTESIAN_POINT ( 'NONE',  ( 15.48339541183756296, -26.71562014373387939, -5.945909248297312821 ) ) ;
#17037=CARTESIAN_POINT ( 'NONE',  ( 14.01165143047478878, 23.97925642646874422, -13.50911357394699408 ) ) ;
#17038=CARTESIAN_POINT ( 'NONE',  ( -11.10756861982300947, 19.59949212537556562, -20.90349153980999830 ) ) ;
#17041=CARTESIAN_POINT ( 'NONE',  ( -27.28398544816837301, -24.17053003994573501, -8.444893248965209764 ) ) ;
#17043=CARTESIAN_POINT ( 'NONE',  ( 2.765300921622650066, -20.42095854668841781, -28.28989953578760819 ) ) ;
#17044=CARTESIAN_POINT ( 'NONE',  ( 15.23366524578394454, 25.71175763003608594, -8.771869565430169047 ) ) ;
#17045=CARTESIAN_POINT ( 'NONE',  ( 20.95229438974030955, 12.90995417087104435, -7.918639165910762223 ) ) ;
#17048=CARTESIAN_POINT ( 'NONE',  ( -5.786258051655946311, 33.33688689327384935, -12.01593827444259510 ) ) ;
#17056=DIRECTION ( 'NONE',  ( -1.000000000000000000, 0.000000000000000000, 0.000000000000000000 ) ) ;
#17058=CARTESIAN_POINT ( 'NONE',  ( -30.46048998099726290, 0.1440795296772170719, -7.358614350216769573 ) ) ;
#17060=CARTESIAN_POINT ( 'NONE',  ( 26.21350394291775388, -7.054572422158140732, -17.77726368305027194 ) ) ;
#17064=CARTESIAN_POINT ( 'NONE',  ( 19.48557158514982746, -11.25000000000009415, -0.000000000000000000 ) ) ;
#17077=CARTESIAN_POINT ( 'NONE',  ( 18.30429174972384843, 17.59035370715124103, -9.358262485240686601 ) ) ;
#17079=CARTESIAN_POINT ( 'NONE',  ( 11.69942483974685921, 33.41113235942790993, -5.889308325164201108 ) ) ;
#17084=CARTESIAN_POINT ( 'NONE',  ( 13.44501532575884717, -23.11853366065025739, -15.40642888925075127 ) ) ;
#17085=PLANE ( 'NONE',  #29503 ) ;
#17088=CARTESIAN_POINT ( 'NONE',  ( -15.01279892861110987, 25.98643013970960780, -9.237413099304763620 ) ) ;
#17091=CARTESIAN_POINT ( 'NONE',  ( 14.88344483570274335, -26.39785593533024155, -7.359431359455702371 ) ) ;
#17093=VERTEX_POINT ( 'NONE', #34282 ) ;
#17095=CARTESIAN_POINT ( 'NONE',  ( -9.677466622934531415, 26.64163155314981068, -15.96543401049129507 ) ) ;
#17098=AXIS2_PLACEMENT_3D ( 'NONE', #17835, #27359, #2386 ) ;
#17100=CARTESIAN_POINT ( 'NONE',  ( -28.07610024992567332, -6.064277111074432014, -15.90283520499208691 ) ) ;
#17103=CARTESIAN_POINT ( 'NONE',  ( 27.64211024490576207, 0.3180281332077250500, -13.52072714143753096 ) ) ;
#17109=CARTESIAN_POINT ( 'NONE',  ( -29.60645524828415276, 0.03829841260466283065, -10.17951810148429637 ) ) ;
#17112=CARTESIAN_POINT ( 'NONE',  ( 21.44822029382961404, -1.048543745050170450, -24.81695474169817928 ) ) ;
#17128=CARTESIAN_POINT ( 'NONE',  ( 4.995981679244292373, 37.69300919626899571, -5.860311672130957383 ) ) ;
#17132=CARTESIAN_POINT ( 'NONE',  ( 13.75932650634318399, -16.19533518725610577, -25.84441635423754136 ) ) ;
#17136=CARTESIAN_POINT ( 'NONE',  ( 12.87995330630399060, 21.73368077170972512, -17.42658506456785261 ) ) ;
#17137=VECTOR ( 'NONE', #24509, 1000.000000000000000 ) ;
#17139=CARTESIAN_POINT ( 'NONE',  ( -11.48487407195851695, 17.12429978707877254, -28.10317327323546976 ) ) ;
#17142=CARTESIAN_POINT ( 'NONE',  ( 13.24447573026784397, 22.17338430882927724, -16.44949393079923894 ) ) ;
#17144=CARTESIAN_POINT ( 'NONE',  ( 17.87465767731121957, -11.31086339180266798, -26.25773876253557759 ) ) ;
#17146=CARTESIAN_POINT ( 'NONE',  ( -12.74236390228968041, 21.95782657198702736, -17.39615765752699517 ) ) ;
#17147=DIRECTION ( 'NONE',  ( -0.000000000000000000, -0.000000000000000000, 1.000000000000000000 ) ) ;
#17148=CARTESIAN_POINT ( 'NONE',  ( -11.66927690283585228, -19.78180214246283697, -21.50613042839750833 ) ) ;
#17153=CARTESIAN_POINT ( 'NONE',  ( -21.02740630788312259, -8.711873245778782859, -23.03796868434001865 ) ) ;
#17154=CARTESIAN_POINT ( 'NONE',  ( -12.62124997321451048, -23.07266609165860771, -15.47605775495894243 ) ) ;
#17156=CARTESIAN_POINT ( 'NONE',  ( 13.79761723546635643, 16.77350094813697368, -23.03736194697137307 ) ) ;
#17158=CARTESIAN_POINT ( 'NONE',  ( 27.31048934271396433, 3.779197449542496035, -6.904998494663478148 ) ) ;
#17163=CARTESIAN_POINT ( 'NONE',  ( -21.30018192981278347, 0.6028086581825573553, -24.99559268264187750 ) ) ;
#17164=CARTESIAN_POINT ( 'NONE',  ( 28.75502359630104721, -0.3820146305305825440, -12.49841367032799866 ) ) ;
#17168=CARTESIAN_POINT ( 'NONE',  ( -28.09305766860465425, 2.631505933142144649, -7.850560883495491638 ) ) ;
#17169=CARTESIAN_POINT ( 'NONE',  ( 15.29245034862073460, 32.56469986092002955, -13.99876745781544685 ) ) ;
#17178=CARTESIAN_POINT ( 'NONE',  ( -24.40045231895073385, 6.107632861236318433, -11.80004717437143746 ) ) ;
#17181=CARTESIAN_POINT ( 'NONE',  ( 27.56730585349385620, -23.98784956095697396, -8.441368152517451762 ) ) ;
#17185=CARTESIAN_POINT ( 'NONE',  ( 15.26389162175653880, 27.29890105065966921, -4.999999999999999112 ) ) ;
#17188=CARTESIAN_POINT ( 'NONE',  ( -17.31869546780055558, 18.97017784545571573, -10.80183007974773624 ) ) ;
#17190=CARTESIAN_POINT ( 'NONE',  ( 15.33814677726094189, -26.70409432335911859, -5.000000000000000888 ) ) ;
#17192=CARTESIAN_POINT ( 'NONE',  ( 11.08133522239378088, 17.49689473911582027, -27.44844487583075221 ) ) ;
#17194=CARTESIAN_POINT ( 'NONE',  ( 11.03000241580673979, 17.43158562307755943, -28.07681393002727077 ) ) ;
#17196=CARTESIAN_POINT ( 'NONE',  ( -15.30416065479365351, 26.73672882626205194, -6.885395080861467676 ) ) ;
#17198=CARTESIAN_POINT ( 'NONE',  ( -11.14927767355199784, -20.47484563554826664, -20.54567832761641100 ) ) ;
#17200=CARTESIAN_POINT ( 'NONE',  ( -29.68001125634650705, -19.19152806808636313, -11.07052693527171705 ) ) ;
#17201=CARTESIAN_POINT ( 'NONE',  ( -6.807649496723200855, -24.62777695444815151, -9.837064774307107129 ) ) ;
#17202=CARTESIAN_POINT ( 'NONE',  ( 15.77104256730297749, 25.16267426227344828, -6.891571856456937262 ) ) ;
#17204=CARTESIAN_POINT ( 'NONE',  ( 24.02933105728603991, 8.309275822838595005, -5.000000000000000000 ) ) ;
#17210=CARTESIAN_POINT ( 'NONE',  ( -20.53668341592966939, -1.131593473639494807, -28.63651727350685050 ) ) ;
#17214=DIRECTION ( 'NONE',  ( -1.000000000000000000, 0.000000000000000000, 0.000000000000000000 ) ) ;
#17217=CARTESIAN_POINT ( 'NONE',  ( 34.23814126792781565, -17.55187814006816538, -4.999999999999996447 ) ) ;
#17224=CARTESIAN_POINT ( 'NONE',  ( 0.4114189264675333080, 38.49512827994399800, -5.435433640322397508 ) ) ;
#17233=CARTESIAN_POINT ( 'NONE',  ( 12.88278855606390394, 23.95175969909016089, -15.32450620224983950 ) ) ;
#17237=CARTESIAN_POINT ( 'NONE',  ( -19.45999784437984914, 12.76325622095678725, -14.91856487225177474 ) ) ;
#17242=CARTESIAN_POINT ( 'NONE',  ( 15.52090202525632279, -26.75102145164868972, -5.474045156224585540 ) ) ;
#17245=CARTESIAN_POINT ( 'NONE',  ( 14.82688042600062239, 25.65053735475629182, -10.17772289843519573 ) ) ;
#17246=CARTESIAN_POINT ( 'NONE',  ( -18.07620401364299667, 24.68088026512193522, -5.000000000000000000 ) ) ;
#17248=CARTESIAN_POINT ( 'NONE',  ( -19.89493131341646048, -18.69241546286294309, -17.73959074223588317 ) ) ;
#17249=CARTESIAN_POINT ( 'NONE',  ( 2.901613786040809551, -20.88678771515551702, -24.38864445180290375 ) ) ;
#17250=CARTESIAN_POINT ( 'NONE',  ( 12.54845838944650183, 20.28352347061387917, -19.52372391363399728 ) ) ;
#17251=CARTESIAN_POINT ( 'NONE',  ( 18.20215074981739889, 13.29937655356881265, -17.99813131470672900 ) ) ;
#17254=CARTESIAN_POINT ( 'NONE',  ( -4.991427726885995675, 21.31633811110100041, -24.36793799711855968 ) ) ;
#17257=ORIENTED_EDGE ( 'NONE', *, *, #11017, .T. ) ;
#17261=EDGE_CURVE ( 'NONE', #1450, #35955, #38728, .T. ) ;
#17264=CARTESIAN_POINT ( 'NONE',  ( -30.68739395818431959, 0.1797671858537340517, -4.999999999999999112 ) ) ;
#17266=CARTESIAN_POINT ( 'NONE',  ( 33.70584737762637673, -11.25103427847470172, -9.773660813979208939 ) ) ;
#17275=CARTESIAN_POINT ( 'NONE',  ( 3.863783140547853712E-14, -86.77689918168233874, -0.000000000000000000 ) ) ;
#17284=CARTESIAN_POINT ( 'NONE',  ( 19.07008944147191443, 16.95185708702321747, -5.480395098389816866 ) ) ;
#17285=CARTESIAN_POINT ( 'NONE',  ( 8.205360533218383878, 25.51929248090862501, -17.85775526361365806 ) ) ;
#17289=CARTESIAN_POINT ( 'NONE',  ( 9.937768194491171769, -17.93102150851172993, -30.00000000000000000 ) ) ;
#17294=CARTESIAN_POINT ( 'NONE',  ( -15.28567255210324838, 26.54645022884873384, -7.357307290646502018 ) ) ;
#17297=CARTESIAN_POINT ( 'NONE',  ( 9.195945848978588799, -18.32167064559432035, -30.00000000000000000 ) ) ;
#17301=CARTESIAN_POINT ( 'NONE',  ( -7.104430329252444665, 19.30332660575202297, -28.55946829698027045 ) ) ;
#17304=CARTESIAN_POINT ( 'NONE',  ( -20.91604292039119173, -3.820787406694753585, -25.84273227370559312 ) ) ;
#17307=CARTESIAN_POINT ( 'NONE',  ( 27.69998584925471619, 0.2404071644066830549, -13.51635162220101627 ) ) ;
#17312=CARTESIAN_POINT ( 'NONE',  ( -30.72389070028295777, -0.02887358500283720292, -6.887897371773664013 ) ) ;
#17315=EDGE_CURVE ( 'NONE', #18367, #33916, #26113, .T. ) ;
#17316=CARTESIAN_POINT ( 'NONE',  ( 33.22294079836321856, -4.074934819707171307, -8.143877639058281659 ) ) ;
#17329=CARTESIAN_POINT ( 'NONE',  ( 3.355814016059087468, 25.38759446419620147, -19.67824355085762278 ) ) ;
#17333=CARTESIAN_POINT ( 'NONE',  ( 18.63134831210867404, -25.78775970246520188, -10.44478608498117289 ) ) ;
#17337=VERTEX_POINT ( 'NONE', #33053 ) ;
#17338=CARTESIAN_POINT ( 'NONE',  ( 15.37925838865456996, 26.91354363167639363, -5.473566364682137753 ) ) ;
#17340=CARTESIAN_POINT ( 'NONE',  ( -14.94814311929064132, 25.28441830965897807, -10.18638070629203618 ) ) ;
#17344=CARTESIAN_POINT ( 'NONE',  ( 14.87527538485814027, 25.50334810396817176, -10.18232127768725626 ) ) ;
#17346=CARTESIAN_POINT ( 'NONE',  ( 21.26206063148141467, -12.57871523600208441, -20.68868112704091189 ) ) ;
#17348=CARTESIAN_POINT ( 'NONE',  ( -14.44959290368749016, 27.62540214084364010, -9.158983685620894377 ) ) ;
#17350=CARTESIAN_POINT ( 'NONE',  ( -10.42186838066264087, -18.08256185635291047, -26.76705096067638934 ) ) ;
#17355=CARTESIAN_POINT ( 'NONE',  ( -19.46103219778806093, -6.726610151890429989, -28.47929083369243131 ) ) ;
#17356=CARTESIAN_POINT ( 'NONE',  ( -14.92665030077538724, -26.52727164316652164, -6.417579119027339907 ) ) ;
#17358=CARTESIAN_POINT ( 'NONE',  ( 13.23034956895627268, 15.71535633465425619, -28.78767767912723130 ) ) ;
#17360=CARTESIAN_POINT ( 'NONE',  ( 20.35897324780223272, 3.107494928291200331, -28.17405716974139196 ) ) ;
#17366=CARTESIAN_POINT ( 'NONE',  ( -30.52913824356789618, -0.1914677198932651925, -8.288054658077042447 ) ) ;
#17368=CARTESIAN_POINT ( 'NONE',  ( 31.23646475641210429, -0.5774691780063523350, -6.872549786655949511 ) ) ;
#17372=CARTESIAN_POINT ( 'NONE',  ( -23.62278170705122449, 1.244602331402794304, -19.58093624668523347 ) ) ;
#17373=CARTESIAN_POINT ( 'NONE',  ( -22.40982762235195835, 2.618079236897030704, -21.24786896499725231 ) ) ;
#17374=CARTESIAN_POINT ( 'NONE',  ( 75.15099915297797395, 43.38844959084117647, 0.000000000000000000 ) ) ;
#17378=VECTOR ( 'NONE', #16595, 1000.000000000000000 ) ;
#17384=CARTESIAN_POINT ( 'NONE',  ( -21.96241518972654205, 5.878577984738289963, -18.91332339141946051 ) ) ;
#17387=CARTESIAN_POINT ( 'NONE',  ( 16.73034041975913766, -16.38034227348617478, -22.03442445900950375 ) ) ;
#17391=CARTESIAN_POINT ( 'NONE',  ( 10.70229295774111478, 17.48483442551455269, -30.00000000000000000 ) ) ;
#17394=CARTESIAN_POINT ( 'NONE',  ( -15.84802793396828235, 21.63412679409943706, -11.70048637574523553 ) ) ;
#17396=CARTESIAN_POINT ( 'NONE',  ( 9.656026013581104905, -18.45733997954168260, -26.83334999707987834 ) ) ;
#17398=CARTESIAN_POINT ( 'NONE',  ( 12.40569181072914873, 20.47107099798277119, -19.49903299958157632 ) ) ;
#17400=CARTESIAN_POINT ( 'NONE',  ( 10.98647152928299597, 17.30743895948370081, -30.00000000000000000 ) ) ;
#17402=CARTESIAN_POINT ( 'NONE',  ( -10.94140927258908746, 17.38955668528554810, -28.70426223197859628 ) ) ;
#17404=CARTESIAN_POINT ( 'NONE',  ( -9.982340082043387852, -18.80733487794834247, -25.01271746743459801 ) ) ;
#17406=CARTESIAN_POINT ( 'NONE',  ( -30.31686021207967840, -19.60108723602752079, -10.17585211697064551 ) ) ;
#17407=CARTESIAN_POINT ( 'NONE',  ( -8.528322800344751542, -23.99199305410463978, -12.74934014457994813 ) ) ;
#17408=CARTESIAN_POINT ( 'NONE',  ( 12.64274550584182677, 19.31738184857981722, -20.62888840247773459 ) ) ;
#17410=CARTESIAN_POINT ( 'NONE',  ( 19.41880252833811227, 6.610239277501288591, -30.00000000000000355 ) ) ;
#17415=CARTESIAN_POINT ( 'NONE',  ( -30.59866543348816847, -1.498850244747759852, -10.54007705693969399 ) ) ;
#17422=VECTOR ( 'NONE', #6450, 1000.000000000000000 ) ;
#17430=CARTESIAN_POINT ( 'NONE',  ( 0.3823767728919280073, 35.39900042147797876, -11.06749343438611177 ) ) ;
#17437=CARTESIAN_POINT ( 'NONE',  ( 9.576129340711554860, 18.19128242950044694, -28.64815163939478637 ) ) ;
#17441=CARTESIAN_POINT ( 'NONE',  ( -19.02768546262373661, 16.45169234481391385, -8.391276880365140300 ) ) ;
#17444=CARTESIAN_POINT ( 'NONE',  ( 14.63889446902708791, -25.46407214954848897, -10.65228754373935516 ) ) ;
#17446=CARTESIAN_POINT ( 'NONE',  ( 14.01698243316408465, 23.96616428142242583, -13.51035568235244888 ) ) ;
#17448=CARTESIAN_POINT ( 'NONE',  ( 16.84920187454417828, 29.09530251867925443, -5.000000000000000000 ) ) ;
#17451=CARTESIAN_POINT ( 'NONE',  ( -24.43528513514284484, -21.68118427706984619, -12.95374139831338844 ) ) ;
#17452=CARTESIAN_POINT ( 'NONE',  ( 4.888870946759487524, -21.71378906137520559, -20.01250066659168070 ) ) ;
#17453=CARTESIAN_POINT ( 'NONE',  ( 15.12975596931773303, 25.61721673019504664, -9.242751917011917229 ) ) ;
#17454=CARTESIAN_POINT ( 'NONE',  ( 20.13608159894178229, 13.64158595004140118, -10.38155476756366546 ) ) ;
#17457=CARTESIAN_POINT ( 'NONE',  ( -4.687651652602798258, 27.18500950432644814, -17.67400160435538936 ) ) ;
#17465=CARTESIAN_POINT ( 'NONE',  ( -29.21513571016266653, 0.4812426229608742778, -10.19062845617733792 ) ) ;
#17467=CARTESIAN_POINT ( 'NONE',  ( 35.42524632062607282, -11.88397916807875809, -5.867122752966118959 ) ) ;
#17470=EDGE_CURVE ( 'NONE', #35629, #7370, #31443, .T. ) ;
#17483=CARTESIAN_POINT ( 'NONE',  ( 18.65259608150544324, 16.46909145568280763, -10.35352517064599809 ) ) ;
#17484=CARTESIAN_POINT ( 'NONE',  ( 7.508979622877860471, 21.09273152055256162, -23.33378713927033843 ) ) ;
#17490=CARTESIAN_POINT ( 'NONE',  ( 12.85713553451835622, -22.56248978612570966, -16.42156014717959067 ) ) ;
#17493=CARTESIAN_POINT ( 'NONE',  ( 18.07620401364302865, 24.68088026512193167, -13.58461195433497082 ) ) ;
#17494=CARTESIAN_POINT ( 'NONE',  ( -11.67752460253681335, 18.91976605311634074, -22.73368238245046058 ) ) ;
#17497=CARTESIAN_POINT ( 'NONE',  ( 13.68001087461786014, -26.27761246146546625, -5.946931794816848083 ) ) ;
#17502=CARTESIAN_POINT ( 'NONE',  ( -11.09189806811868451, 30.64568619558879092, -11.25123976201009768 ) ) ;
#17505=CARTESIAN_POINT ( 'NONE',  ( -25.24817616836305234, -4.671370533674584991, -18.94551454778549271 ) ) ;
#17508=CARTESIAN_POINT ( 'NONE',  ( 21.70043827152030147, 0.7738983909411112361, -23.85944868390605933 ) ) ;
#17513=CARTESIAN_POINT ( 'NONE',  ( -30.78169477786137165, -0.02024540836640525976, -6.417008053751995789 ) ) ;
#17517=CARTESIAN_POINT ( 'NONE',  ( 23.42190877138765970, -2.678843437355377333, -21.21129800221541473 ) ) ;
#17530=CARTESIAN_POINT ( 'NONE',  ( 7.126104678631604905, 36.82515065381944197, -4.999999999999999112 ) ) ;
#17534=CARTESIAN_POINT ( 'NONE',  ( 12.70332137780860648, -16.96759668345817929, -25.93924617538274546 ) ) ;
#17539=CARTESIAN_POINT ( 'NONE',  ( 10.89778913317478626, 17.36343269013392643, -29.34648515220084164 ) ) ;
#17541=CARTESIAN_POINT ( 'NONE',  ( -11.48506209758023466, 17.53631524467423120, -26.25656942401292682 ) ) ;
#17544=CARTESIAN_POINT ( 'NONE',  ( 15.33365340323996051, 26.38076590146513922, -7.358350115893553145 ) ) ;
#17546=CARTESIAN_POINT ( 'NONE',  ( 29.89701346908697488, -18.95835593754587123, -11.06832977680900498 ) ) ;
#17548=CARTESIAN_POINT ( 'NONE',  ( -10.65603027360134902, 17.51308114404589844, -29.99999999999999289 ) ) ;
#17550=CARTESIAN_POINT ( 'NONE',  ( -18.07817403047586780, -26.86642225889332281, -7.745473075693468878 ) ) ;
#17551=B_SPLINE_CURVE_WITH_KNOTS ( 'NONE', 3,
 ( #15084, #24229, #8798, #5741, #30131, #18148, #18336, #2892, #37020, #17552, #29926 ),
 .UNSPECIFIED., .F., .F.,
 ( 4, 1, 1, 1, 1, 1, 1, 1, 4 ),
 ( 0.000000000000000000, 0.1249999999999998612, 0.2499999999999997224, 0.3749999999999995559, 0.5000000000000000000, 0.6250000000000004441, 0.7500000000000003331, 0.8750000000000001110, 1.000000000000000000 ),
 .UNSPECIFIED. ) ;
#17552=CARTESIAN_POINT ( 'NONE',  ( 16.84920187454417828, 29.09530251867925443, -5.000000000000000000 ) ) ;
#17554=CARTESIAN_POINT ( 'NONE',  ( -19.53919056584213365, -7.419766065029655522, -27.01108906676794064 ) ) ;
#17555=CARTESIAN_POINT ( 'NONE',  ( -11.80268877440303932, -22.03891725494794684, -17.47952885073186380 ) ) ;
#17557=ORIENTED_EDGE ( 'NONE', *, *, #30446, .F. ) ;
#17558=CARTESIAN_POINT ( 'NONE',  ( 28.40256726208064819, 1.176742560656635961, -10.68423771036775349 ) ) ;
#17563=CARTESIAN_POINT ( 'NONE',  ( -21.28582742437048125, 0.7081099580931202730, -25.00715929252305614 ) ) ;
#17565=CARTESIAN_POINT ( 'NONE',  ( 26.94956399649580447, -0.4151258792086239269, -15.36823525240014021 ) ) ;
#17570=CARTESIAN_POINT ( 'NONE',  ( -26.58565005577111506, 1.039147901724387646, -14.52972379629277278 ) ) ;
#17571=CARTESIAN_POINT ( 'NONE',  ( -33.62187204924172335, 0.04418559750806146796, -5.000000000000000000 ) ) ;
#17572=DIRECTION ( 'NONE',  ( -1.000000000000000000, 0.000000000000000000, 0.000000000000000000 ) ) ;
#17581=CARTESIAN_POINT ( 'NONE',  ( -24.65099977277350618, 5.218662007276516412, -12.76667628574117330 ) ) ;
#17583=DIRECTION ( 'NONE',  ( 0.000000000000000000, 0.000000000000000000, 1.000000000000000000 ) ) ;
#17584=CARTESIAN_POINT ( 'NONE',  ( 23.98745773934783188, -24.95113523879620487, -9.823517314964597347 ) ) ;
#17591=CARTESIAN_POINT ( 'NONE',  ( 13.29767035538005970, 23.20272292486270516, -15.40656767438932384 ) ) ;
#17594=CARTESIAN_POINT ( 'NONE',  ( -15.42899087826043036, 19.21586207912160305, -15.69889121110926844 ) ) ;
#17597=CARTESIAN_POINT ( 'NONE',  ( 12.41340058665741175, 20.46094404086849750, -19.50037637990314821 ) ) ;
#17601=CARTESIAN_POINT ( 'NONE',  ( -11.82408859876377250, 19.45482954233215622, -21.60399388538399634 ) ) ;
#17602=DIRECTION ( 'NONE',  ( 1.000000000000000000, 0.000000000000000000, 0.000000000000000000 ) ) ;
#17603=CARTESIAN_POINT ( 'NONE',  ( -12.29769356462352903, -22.02265038325488433, -17.43646041213484565 ) ) ;
#17606=CARTESIAN_POINT ( 'NONE',  ( -32.63711378803102292, -17.08632674381000172, -9.283697192344297022 ) ) ;
#17607=CARTESIAN_POINT ( 'NONE',  ( -6.123308122133267695, -19.62006737319780569, -30.00000000000000711 ) ) ;
#17609=CARTESIAN_POINT ( 'NONE',  ( 12.54359778609175891, 18.68447145445714597, -21.72596103221125929 ) ) ;
#17611=CARTESIAN_POINT ( 'NONE',  ( 22.44265844834124124, 7.045391211222152172, -15.86482432176597790 ) ) ;
#17617=CARTESIAN_POINT ( 'NONE',  ( -22.04621557984713220, -1.995498420971771436, -23.53374920157571637 ) ) ;
#17619=CARTESIAN_POINT ( 'NONE',  ( 28.94423758251556222, 0.03876896675481636412, -11.59331513696461258 ) ) ;
#17622=ADVANCED_FACE ( 'NONE', ( #18397 ), #15737, .F. ) ;
#17632=CARTESIAN_POINT ( 'NONE',  ( 75.15099915297797395, 43.38844959084117647, 0.000000000000000000 ) ) ;
#17633=CARTESIAN_POINT ( 'NONE',  ( 0.2238614515109842162, 21.14277272035508659, -26.25630678787392824 ) ) ;
#17634=CIRCLE ( 'NONE', #27353, 60.00000000000014211 ) ;
#17642=CARTESIAN_POINT ( 'NONE',  ( 14.77883339423700448, 28.03561339302072497, -7.318319975446966552 ) ) ;
#17645=CARTESIAN_POINT ( 'NONE',  ( -18.07518878564494713, 14.05505073002865579, -16.95006174505777707 ) ) ;
#17649=CARTESIAN_POINT ( 'NONE',  ( 13.39743745724321045, -23.62495958482203307, -14.47428836996529000 ) ) ;
#17651=CARTESIAN_POINT ( 'NONE',  ( 13.47602490618416304, 22.84703953731449744, -15.44714390386671710 ) ) ;
#17652=CARTESIAN_POINT ( 'NONE',  ( -20.66458278928016057, 17.76169105511799273, -5.000000000000000888 ) ) ;
#17654=CARTESIAN_POINT ( 'NONE',  ( -27.48658736596179963, -21.56671790654684884, -11.09299434450578659 ) ) ;
#17655=CARTESIAN_POINT ( 'NONE',  ( 1.801982192410312766, -24.64865591106047660, -7.429003440711998252 ) ) ;
#17656=CARTESIAN_POINT ( 'NONE',  ( 13.10586528640805604, 21.36746738750283114, -17.46679796181676281 ) ) ;
#17657=CARTESIAN_POINT ( 'NONE',  ( 17.51797765111094307, 10.67563444151121033, -29.99999999999999645 ) ) ;
#17660=CARTESIAN_POINT ( 'NONE',  ( -4.727343333413158710, 20.18853994959099651, -27.77675044586279895 ) ) ;
#17669=CARTESIAN_POINT ( 'NONE',  ( -20.52066404987779791, 0.9821139164781407249, -28.71129986131551703 ) ) ;
#17671=CARTESIAN_POINT ( 'NONE',  ( 27.05781474705212375, -9.043496247948464628, -16.72532308214699270 ) ) ;
#17672=ORIENTED_EDGE ( 'NONE', *, *, #31617, .F. ) ;
#17685=CARTESIAN_POINT ( 'NONE',  ( 15.29022352314591870, 13.67480013622697044, -30.00000000000001066 ) ) ;
#17686=CARTESIAN_POINT ( 'NONE',  ( 7.754350537738645244, 21.81137704913313868, -22.19334008859113538 ) ) ;
#17688=CARTESIAN_POINT ( 'NONE',  ( -22.36636065667467221, 10.81625050891080164, -5.966924272146592045 ) ) ;
#17693=CARTESIAN_POINT ( 'NONE',  ( 10.12794487532474719, -18.74775046445166993, -24.99559475216551263 ) ) ;
#17695=CARTESIAN_POINT ( 'NONE',  ( 18.07620401364302865, 24.68088026512193522, -5.000000000000000000 ) ) ;
#17696=CARTESIAN_POINT ( 'NONE',  ( -14.52552742914873640, 24.99026629062174365, -11.59761377287194151 ) ) ;
#17697=CARTESIAN_POINT ( 'NONE',  ( 13.56094288467416753, -26.09349823019973869, -7.365016121655886039 ) ) ;
#17703=CARTESIAN_POINT ( 'NONE',  ( -8.754768201593860155, 24.05476072843883983, -18.96584428646194098 ) ) ;
#17709=CARTESIAN_POINT ( 'NONE',  ( 30.42199879797928119, 0.05422021819292949935, -7.828243430681267157 ) ) ;
#17714=CARTESIAN_POINT ( 'NONE',  ( -26.49304050658699339, 0.2940916338183011125, -15.45185423700121774 ) ) ;
#17717=CARTESIAN_POINT ( 'NONE',  ( 20.99914968644306867, -2.977695377099063290, -25.90524470544396962 ) ) ;
#17731=CARTESIAN_POINT ( 'NONE',  ( 4.643464871730170529, 23.98615981536725883, -20.80716177970646541 ) ) ;
#17733=CARTESIAN_POINT ( 'NONE',  ( -12.11431921870781281, -16.53859995802357474, -30.00000000000001066 ) ) ;
#17736=CARTESIAN_POINT ( 'NONE',  ( 19.77033395158426288, -27.21289834263597740, -5.910049683774938778 ) ) ;
#17739=PLANE ( 'NONE',  #16167 ) ;
#17742=CARTESIAN_POINT ( 'NONE',  ( 13.42936096295450099, 22.94210890876663456, -15.43620599078790434 ) ) ;
#17744=CARTESIAN_POINT ( 'NONE',  ( -12.53790509067911074, 19.44194302981471623, -20.61120958872907138 ) ) ;
#17748=CARTESIAN_POINT ( 'NONE',  ( 11.12672621128664296, 17.36766021414478089, -28.08254997068604553 ) ) ;
#17751=CARTESIAN_POINT ( 'NONE',  ( 32.51966212229606867, -20.60195123665384287, -4.999999999999998224 ) ) ;
#17753=CARTESIAN_POINT ( 'NONE',  ( -11.39209870729926166, 19.18961260050172513, -22.68434712264469155 ) ) ;
#17755=CARTESIAN_POINT ( 'NONE',  ( -10.28721823975710059, -17.89894537374451744, -28.03678530533794344 ) ) ;
#17759=CARTESIAN_POINT ( 'NONE',  ( -30.05994772858080921, -10.30773001763154539, -13.86984580451319538 ) ) ;
#17760=CARTESIAN_POINT ( 'NONE',  ( -15.22509278422137768, -26.60142203870535127, -6.417211518553083138 ) ) ;
#17763=CARTESIAN_POINT ( 'NONE',  ( 27.48662654444790476, 1.221943985062914795, -12.60017615557705462 ) ) ;
#17767=CARTESIAN_POINT ( 'NONE',  ( -22.75659833837781676, 0.5252670190201254030, -21.60573177101157327 ) ) ;
#17768=ORIENTED_EDGE ( 'NONE', *, *, #7689, .F. ) ;
#17769=CARTESIAN_POINT ( 'NONE',  ( 21.02639339174489308, 0.1643985004216583778, -26.16791350077025058 ) ) ;
#17774=CARTESIAN_POINT ( 'NONE',  ( -26.91927498037264499, 4.412534205184938330, -5.000000000000001776 ) ) ;
#17778=AXIS2_PLACEMENT_3D ( 'NONE', #7607, #26905, #14311 ) ;
#17785=CARTESIAN_POINT ( 'NONE',  ( -23.75513742221500024, 6.044705833718418297, -13.79811425570447980 ) ) ;
#17788=CARTESIAN_POINT ( 'NONE',  ( 15.71069447272513742, -14.48203284589343376, -25.69054009000548788 ) ) ;
#17792=CARTESIAN_POINT ( 'NONE',  ( 15.18466250546081220, 27.13099485538614175, -6.876955971306166759 ) ) ;
#17796=CARTESIAN_POINT ( 'NONE',  ( -13.48553142464132115, 15.75358007923588843, -27.02007185819866208 ) ) ;
#17799=CARTESIAN_POINT ( 'NONE',  ( 13.77977818563562096, 23.37426034515904760, -14.47731727276712554 ) ) ;
#17801=CARTESIAN_POINT ( 'NONE',  ( 11.18323034263230120, 17.75715498309746820, -26.22476241273412256 ) ) ;
#17803=CARTESIAN_POINT ( 'NONE',  ( -15.32605299005571808, 26.83348367465769968, -6.414615797237237516 ) ) ;
#17805=CARTESIAN_POINT ( 'NONE',  ( -12.34719756161035242, -22.02191913002371848, -17.43064001291457288 ) ) ;
#17807=CARTESIAN_POINT ( 'NONE',  ( -17.55945971783640758, -10.59693620792911872, -29.21186350523559483 ) ) ;
#17809=CARTESIAN_POINT ( 'NONE',  ( -7.003108942385479097, -21.17426981051016810, -20.95153987240063742 ) ) ;
#17811=CARTESIAN_POINT ( 'NONE',  ( 12.01362727457946278, 17.13078155611268727, -26.30899361330535058 ) ) ;
#17813=CARTESIAN_POINT ( 'NONE',  ( 25.09257354179462496, 6.456226081335884714, -7.888698583467808056 ) ) ;
#17818=CARTESIAN_POINT ( 'NONE',  ( -23.76582790367996267, -0.8399181250771553531, -20.35841962654769688 ) ) ;
#17820=CARTESIAN_POINT ( 'NONE',  ( 20.61369574458117171, 0.7924611088881369225, -28.07461411969941878 ) ) ;
#17823=CARTESIAN_POINT ( 'NONE',  ( 27.08779848459123585, 7.221796966026763798, -5.000000000000007105 ) ) ;
#17830=CARTESIAN_POINT ( 'NONE',  ( 1.341253818658974861, 32.42268633335680050, -13.80665395263008399 ) ) ;
#17835=CARTESIAN_POINT ( 'NONE',  ( 3.863783140547853712E-14, -86.77689918168233874, -5.000000000000000000 ) ) ;
#17839=CARTESIAN_POINT ( 'NONE',  ( 10.41341893350470293, 19.30400416985194667, -23.68959501837800019 ) ) ;
#17842=CARTESIAN_POINT ( 'NONE',  ( -17.18163521729151455, 14.39254400151518176, -19.00291312292943857 ) ) ;
#17846=CARTESIAN_POINT ( 'NONE',  ( 10.26099256397509407, -19.15184415471343016, -23.84939042261497377 ) ) ;
#17848=CARTESIAN_POINT ( 'NONE',  ( 15.00904765070272973, 25.99870026096500908, -9.236802632963790671 ) ) ;
#17853=CARTESIAN_POINT ( 'NONE',  ( -18.63416092258458434, -14.56412937407352715, -21.89936666682847743 ) ) ;
#17854=CARTESIAN_POINT ( 'NONE',  ( 4.218053344389335990, -20.12689330800646204, -28.26382229294831561 ) ) ;
#17855=CARTESIAN_POINT ( 'NONE',  ( 11.18139086956414729, 17.23420873180600665, -28.71418858328174295 ) ) ;
#17856=CARTESIAN_POINT ( 'NONE',  ( 17.78547439015788001, 10.85037366618364274, -25.51180193807143581 ) ) ;
#17857=LINE ( 'NONE', #30443, #3718 ) ;
#17858=CARTESIAN_POINT ( 'NONE',  ( -4.188474181932830831, 20.68942421501040840, -26.33881144299988009 ) ) ;
#17864=CARTESIAN_POINT ( 'NONE',  ( -21.25244676704415525, 0.9439152883838316521, -25.03239665970995631 ) ) ;
#17866=CARTESIAN_POINT ( 'NONE',  ( 19.63120307387857011, -5.935663759831210307, -29.99999999999999289 ) ) ;
#17867=EDGE_CURVE ( 'NONE', #6755, #37897, #8983, .T. ) ;
#17881=CARTESIAN_POINT ( 'NONE',  ( 21.38147419243281178, -17.48660460948667250, -17.66603181204244066 ) ) ;
#17882=EDGE_CURVE ( 'NONE', #3976, #29462, #15449, .T. ) ;
#17883=CARTESIAN_POINT ( 'NONE',  ( 15.91426628502474294, 13.28120225394148157, -26.57843054152041518 ) ) ;
#17884=CARTESIAN_POINT ( 'NONE',  ( 12.37861635401602456, 32.45732457598138154, -6.338864116293123629 ) ) ;
#17886=CARTESIAN_POINT ( 'NONE',  ( -18.47830230920279959, 9.218715770337659876, -27.17425712858404907 ) ) ;
#17890=CARTESIAN_POINT ( 'NONE',  ( 11.54108096491583701, -20.40438889209876905, -20.49457141818385253 ) ) ;
#17893=CARTESIAN_POINT ( 'NONE',  ( -12.92333245884202242, 21.66144175116086856, -17.43645980981951737 ) ) ;
#17894=CARTESIAN_POINT ( 'NONE',  ( -13.73731780760944332, -15.49063096320742083, -27.84253586294682137 ) ) ;
#17895=CARTESIAN_POINT ( 'NONE',  ( 9.195945848978588799, -18.32167064559432035, -29.35440300966851623 ) ) ;
#17899=CARTESIAN_POINT ( 'NONE',  ( -11.70053153659217315, 32.50725898910726386, -8.095625848918006184 ) ) ;
#17903=AXIS2_PLACEMENT_3D ( 'NONE', #123, #6599, #13095 ) ;
#17906=CARTESIAN_POINT ( 'NONE',  ( 30.82841397905490055, -0.0004293619779054370315, -5.946085982635294087 ) ) ;
#17909=ORIENTED_EDGE ( 'NONE', *, *, #9645, .F. ) ;
#17910=CARTESIAN_POINT ( 'NONE',  ( -20.60997075700326775, 0.8574756231443084742, -28.07786192183081653 ) ) ;
#17913=CARTESIAN_POINT ( 'NONE',  ( 28.35998102576435542, -3.361797673834487021, -15.09859322067980436 ) ) ;
#17927=CARTESIAN_POINT ( 'NONE',  ( 7.982650572986060844, 35.32968916061959419, -8.454540784394524167 ) ) ;
#17932=CARTESIAN_POINT ( 'NONE',  ( 16.28755400353538718, -21.47407573242956857, -17.03663477892219547 ) ) ;
#17937=CARTESIAN_POINT ( 'NONE',  ( 10.98606895505122338, 17.46037643935285999, -28.07419226985351557 ) ) ;
#17939=CARTESIAN_POINT ( 'NONE',  ( -15.20434278248479210, 25.80297669556701834, -8.770905639422021949 ) ) ;
#17942=CARTESIAN_POINT ( 'NONE',  ( 15.21665582495734625, 26.14138673791106982, -8.298772713743886698 ) ) ;
#17944=CARTESIAN_POINT ( 'NONE',  ( 20.07973543493038093, -12.71120667207603638, -21.84040384482505814 ) ) ;
#17946=CARTESIAN_POINT ( 'NONE',  ( -10.71119831444032222, 17.63713612967008260, -28.05781784345192165 ) ) ;
#17948=CARTESIAN_POINT ( 'NONE',  ( -15.78324407152631181, -23.72706283566519048, -14.26634486285669290 ) ) ;
#17951=CARTESIAN_POINT ( 'NONE',  ( -22.28223702159144537, -7.691998452970532085, -21.94978931996465477 ) ) ;
#17952=CARTESIAN_POINT ( 'NONE',  ( -14.83319764216063774, -26.20259247624118970, -8.300228564017693600 ) ) ;
#17955=CARTESIAN_POINT ( 'NONE',  ( 24.80179831294707782, 2.145886827218380422, -16.59895774698153303 ) ) ;
#17956=DIRECTION ( 'NONE',  ( 1.000000000000000000, 0.000000000000000000, 0.000000000000000000 ) ) ;
#17959=CARTESIAN_POINT ( 'NONE',  ( -20.61531321053539756, 0.7630595300999895025, -28.07314328191137065 ) ) ;
#17961=CARTESIAN_POINT ( 'NONE',  ( 29.62581357150819983, -0.8124887880752176272, -11.51961869691573703 ) ) ;
#17966=CARTESIAN_POINT ( 'NONE',  ( -27.71315567531769375, 2.639235371980216627, -9.283902402946985433 ) ) ;
#17967=CARTESIAN_POINT ( 'NONE',  ( 12.05832241004688399, 18.99596958976722760, -30.00000000000000000 ) ) ;
#17970=EDGE_CURVE ( 'NONE', #35955, #15787, #32332, .T. ) ;
#17976=CARTESIAN_POINT ( 'NONE',  ( -25.02193947835522536, 6.168178570904315983, -9.344460451553976199 ) ) ;
#17979=CARTESIAN_POINT ( 'NONE',  ( 24.74805592918939112, -25.69571450645518240, -8.048384647129612546 ) ) ;
#17981=CARTESIAN_POINT ( 'NONE',  ( 11.03704933452659098, 18.24793296388573083, -24.97710597946171518 ) ) ;
#17985=CARTESIAN_POINT ( 'NONE',  ( -15.42171207023761426, 20.87087894025797752, -13.66180630862146117 ) ) ;
#17990=DIRECTION ( 'NONE',  ( 0.000000000000000000, 0.000000000000000000, 1.000000000000000000 ) ) ;
#17991=CARTESIAN_POINT ( 'NONE',  ( 14.94931401584148034, 25.75487660405273616, -9.709665385797562109 ) ) ;
#17995=CARTESIAN_POINT ( 'NONE',  ( -14.77757630377099929, 25.80207083792462441, -10.16863076474116312 ) ) ;
#17997=CARTESIAN_POINT ( 'NONE',  ( -15.34706751505450661, -26.51099793413068184, -7.357307595070670558 ) ) ;
#18000=CARTESIAN_POINT ( 'NONE',  ( -17.91007841644879761, -10.80895702151930848, -26.96531573143874638 ) ) ;
#18001=CARTESIAN_POINT ( 'NONE',  ( -13.94379063328525525, -26.36485034788368864, -5.474070472473820281 ) ) ;
#18003=CARTESIAN_POINT ( 'NONE',  ( 16.07071250763885217, 24.35835661434920141, -6.420932443739101103 ) ) ;
#18005=CARTESIAN_POINT ( 'NONE',  ( 25.16591491352843235, 6.464046969047158697, -7.403904741422770996 ) ) ;
#18010=CARTESIAN_POINT ( 'NONE',  ( -30.79868169068296879, -1.128537211814402585, -9.633236635348129795 ) ) ;
#18011=CARTESIAN_POINT ( 'NONE',  ( 31.01989312948269628, -0.1972547478048194691, -5.943848862614698803 ) ) ;
#18015=CARTESIAN_POINT ( 'NONE',  ( 23.06249103411542478, 13.31513540672987972, -13.39439507595155199 ) ) ;
#18023=FACE_OUTER_BOUND ( 'NONE', #28604, .T. ) ;
#18024=CARTESIAN_POINT ( 'NONE',  ( 1.244695916669324998, 30.19017886107374693, -15.67990371887574952 ) ) ;
#18031=CARTESIAN_POINT ( 'NONE',  ( 12.96901561809162651, 24.98310741220821996, -14.31814338936165498 ) ) ;
#18034=CARTESIAN_POINT ( 'NONE',  ( -15.92546573256853648, 12.96094696367512533, -28.84886678414710914 ) ) ;
#18037=CARTESIAN_POINT ( 'NONE',  ( 11.91801038985816596, -21.48403732790968235, -18.45078833793485273 ) ) ;
#18039=CARTESIAN_POINT ( 'NONE',  ( 12.93090914344494813, 21.64873284080854887, -17.43820100889082170 ) ) ;
#18040=CARTESIAN_POINT ( 'NONE',  ( 15.35905905661863180, 26.71843228421901628, -6.416469466895263096 ) ) ;
#18046=CARTESIAN_POINT ( 'NONE',  ( -23.70091659983786414, -19.77374023286659721, -14.78722173017111174 ) ) ;
#18047=CARTESIAN_POINT ( 'NONE',  ( 1.236634163872074366, -20.51914614933548719, -29.42994913469717488 ) ) ;
#18048=CARTESIAN_POINT ( 'NONE',  ( 11.33092883969515441, 17.46816179166363980, -26.84939659920764043 ) ) ;
#18049=CARTESIAN_POINT ( 'NONE',  ( 20.64747291529165807, 12.71173510070245882, -10.38670938929076115 ) ) ;
#18051=CARTESIAN_POINT ( 'NONE',  ( -5.326384147119485490, 37.63231972733477448, -4.999999999999993783 ) ) ;
#18059=CARTESIAN_POINT ( 'NONE',  ( -30.14481262437536913, 0.2169452752166688425, -8.299854351458789026 ) ) ;
#18061=CARTESIAN_POINT ( 'NONE',  ( 29.16243740633159476, -8.764958120439876765, -14.83744052011651249 ) ) ;
#18077=CARTESIAN_POINT ( 'NONE',  ( 17.00786847495595566, -13.87811437483023980, -24.29345988331185424 ) ) ;
#18078=CARTESIAN_POINT ( 'NONE',  ( 19.86842276243890382, 14.78994251298874296, -8.402377087950958057 ) ) ;
#18080=CARTESIAN_POINT ( 'NONE',  ( 9.808884097217401177, 27.70084310347472822, -14.97692238110015417 ) ) ;
#18082=CARTESIAN_POINT ( 'NONE',  ( -18.65382632816861275, 9.289903503710515764, -25.50617801253576999 ) ) ;
#18085=CARTESIAN_POINT ( 'NONE',  ( 15.10432571242179911, -26.01895073574682726, -9.232258709681612885 ) ) ;
#18089=CARTESIAN_POINT ( 'NONE',  ( 27.08779848459123585, 7.221796966026769127, -13.42901749168596304 ) ) ;
#18091=CARTESIAN_POINT ( 'NONE',  ( -13.18985422166703181, 22.27197207924475109, -16.43952829204636146 ) ) ;
#18092=CARTESIAN_POINT ( 'NONE',  ( -16.53877156149134819, -18.57266078395657161, -19.93956889360425322 ) ) ;
#18093=CARTESIAN_POINT ( 'NONE',  ( 13.17310952450038464, -25.48991742312072262, -9.735372911299624121 ) ) ;
#18097=CARTESIAN_POINT ( 'NONE',  ( -11.15150138062039709, 34.02824952835918992, -5.447195920641812350 ) ) ;
#18104=CARTESIAN_POINT ( 'NONE',  ( 20.48067366615298468, 0.8901913013804804153, -30.00000000000000000 ) ) ;
#18109=CARTESIAN_POINT ( 'NONE',  ( -30.87691200222618804, -0.01437998035276831163, -4.999999999999999112 ) ) ;
#18113=CARTESIAN_POINT ( 'NONE',  ( 34.26529024853127936, -5.222454321802834087, -5.897803579761220938 ) ) ;
#18126=CARTESIAN_POINT ( 'NONE',  ( 7.809096289090598830, 34.47606966685644636, -9.783655936083253124 ) ) ;
#18130=CARTESIAN_POINT ( 'NONE',  ( 19.25558875303204687, -26.58026616919283924, -8.617268851883771674 ) ) ;
#18135=CARTESIAN_POINT ( 'NONE',  ( 11.14038654638060244, 17.78806815055257573, -26.22011444304219907 ) ) ;
#18137=CARTESIAN_POINT ( 'NONE',  ( -11.06345206700481931, 17.40955828997764243, -28.07880555279562174 ) ) ;
#18139=CARTESIAN_POINT ( 'NONE',  ( 12.56610953508889494, -22.55658933108479758, -16.45058249204709355 ) ) ;
#18141=CARTESIAN_POINT ( 'NONE',  ( 15.46782449521607283, 26.59794325776330481, -5.474156741759839129 ) ) ;
#18143=CARTESIAN_POINT ( 'NONE',  ( 31.77261430474117532, -21.49768664888851788, -5.435972644969311318 ) ) ;
#18145=CARTESIAN_POINT ( 'NONE',  ( -14.73108631288593529, 28.24757970853271516, -7.312183354124210055 ) ) ;
#18147=CARTESIAN_POINT ( 'NONE',  ( -17.13315098722738483, -24.25158645364346910, -13.25521884679562490 ) ) ;
#18148=CARTESIAN_POINT ( 'NONE',  ( 4.336808689942017736E-15, 40.84107189184581443, -5.000000000000008882 ) ) ;
#18150=CARTESIAN_POINT ( 'NONE',  ( -32.58686633885861994, -12.27975601045717191, -11.10035766972282190 ) ) ;
#18151=CARTESIAN_POINT ( 'NONE',  ( -14.90633381827083070, -26.31176259071834522, -7.829649256883607578 ) ) ;
#18154=CARTESIAN_POINT ( 'NONE',  ( 23.35664678750010381, 2.976149040520807532, -18.70198339929852338 ) ) ;
#18158=CARTESIAN_POINT ( 'NONE',  ( -30.68763588371861672, -0.09248980374888614298, -7.355207434232696961 ) ) ;
#18159=EDGE_LOOP ( 'NONE', ( #32774, #15157, #12073, #28724, #39476, #8310, #4958 ) ) ;
#18160=CARTESIAN_POINT ( 'NONE',  ( 21.03689950211181880, -0.002815931881645192866, -26.15313960796883208 ) ) ;
#18161=AXIS2_PLACEMENT_3D ( 'NONE', #27310, #17583, #36458 ) ;
#18164=CARTESIAN_POINT ( 'NONE',  ( -22.98279762503596757, 2.766379843953515216, -19.73711539544465410 ) ) ;
#18165=AXIS2_PLACEMENT_3D ( 'NONE', #40187, #6061, #12358 ) ;
#18173=CARTESIAN_POINT ( 'NONE',  ( -21.48723061098553444, 7.511881048007619022, -17.95007373264360595 ) ) ;
#18176=CARTESIAN_POINT ( 'NONE',  ( 24.96780582346026733, -24.47691348509939857, -9.803478453495912959 ) ) ;
#18178=CARTESIAN_POINT ( 'NONE',  ( 13.06109374962291092, 22.50549497211172323, -16.41044510421365743 ) ) ;
#18182=CARTESIAN_POINT ( 'NONE',  ( -13.76573679096662417, 19.44551850793918035, -18.63149991976310460 ) ) ;
#18186=CARTESIAN_POINT ( 'NONE',  ( 14.95212139095325199, 25.74619849441134534, -9.709798330206572459 ) ) ;
#18191=CARTESIAN_POINT ( 'NONE',  ( -15.35513899590904430, 26.99708482749830907, -5.000000000000001776 ) ) ;
#18193=CARTESIAN_POINT ( 'NONE',  ( -15.57263558642641854, -26.76429566359157164, -5.473788325833539581 ) ) ;
#18195=CARTESIAN_POINT ( 'NONE',  ( -33.36938334175751208, -17.47479766793881240, -7.973135956092645138 ) ) ;
#18196=CARTESIAN_POINT ( 'NONE',  ( -13.40655439899805756, -25.53642076282103091, -9.731694637308171636 ) ) ;
#18198=CARTESIAN_POINT ( 'NONE',  ( 16.28462322236242343, 23.84466805338936624, -5.948220019300794803 ) ) ;
#18201=CARTESIAN_POINT ( 'NONE',  ( 24.10931265530348000, 7.304982279079090368, -9.852240822340444737 ) ) ;
#18202=CARTESIAN_POINT ( 'NONE',  ( 16.66551504892489888, -27.04635334451238649, -4.999999999999997335 ) ) ;
#18205=DIRECTION ( 'NONE',  ( -1.000000000000000000, 0.000000000000000000, 0.000000000000000000 ) ) ;
#18207=CARTESIAN_POINT ( 'NONE',  ( -20.74142061204233656, -0.1647452484960928165, -27.38238928991409082 ) ) ;
#18208=CARTESIAN_POINT ( 'NONE',  ( 29.41506271722083810, 0.006098485709055394971, -10.64827624646466653 ) ) ;
#18211=CARTESIAN_POINT ( 'NONE',  ( 30.41237130417911771, 3.314011747244131723, -13.58461195433497437 ) ) ;
#18220=CARTESIAN_POINT ( 'NONE',  ( 3.503895337239875118, 34.07186797344890294, -11.98835608762611216 ) ) ;
#18227=CARTESIAN_POINT ( 'NONE',  ( 14.84946995997173325, 27.27879204989079298, -8.260274125225500086 ) ) ;
#18230=CARTESIAN_POINT ( 'NONE',  ( -19.46326072101385307, 15.42234476947875699, -8.889095617120403858 ) ) ;
#18234=CARTESIAN_POINT ( 'NONE',  ( 15.08555043039248389, -26.14723064015357679, -8.767643119045953171 ) ) ;
#18235=CARTESIAN_POINT ( 'NONE',  ( -21.68568904104562023, -27.13690135270087822, -4.999999999999999112 ) ) ;
#18237=CARTESIAN_POINT ( 'NONE',  ( 14.72587059535505283, 25.43166455451370567, -10.65085080139201956 ) ) ;
#18243=CARTESIAN_POINT ( 'NONE',  ( -29.90225311088989812, -23.39525860678804037, -5.437566589666127825 ) ) ;
#18244=CARTESIAN_POINT ( 'NONE',  ( -0.3830839531904912665, -24.55156499636435186, -8.408222294404422925 ) ) ;
#18245=CARTESIAN_POINT ( 'NONE',  ( 11.28710791291100435, 17.16441204958988109, -28.71847994827210471 ) ) ;
#18246=CARTESIAN_POINT ( 'NONE',  ( 22.15128575431291935, 11.07349831676230778, -6.938905347179290750 ) ) ;
#18250=CARTESIAN_POINT ( 'NONE',  ( -4.192884458248775204, 37.73304570911393085, -6.703245015772555604 ) ) ;
#18252=CARTESIAN_POINT ( 'NONE',  ( -20.50046019883160398, -3.737008032862233708, -27.16541881878944764 ) ) ;
#18254=ORIENTED_EDGE ( 'NONE', *, *, #34125, .F. ) ;
#18257=CARTESIAN_POINT ( 'NONE',  ( -24.90203731630741757, 0.9589847940253315439, -17.49505980781958669 ) ) ;
#18258=CARTESIAN_POINT ( 'NONE',  ( 32.62865313406591383, -11.96328060321731357, -11.10430041822750447 ) ) ;
#18260=AXIS2_PLACEMENT_3D ( 'NONE', #33560, #23799, #30701 ) ;
#18270=CARTESIAN_POINT ( 'NONE',  ( -1.657330241813901317, 20.83889105489772220, -26.97771945235741242 ) ) ;
#18274=CARTESIAN_POINT ( 'NONE',  ( 29.07166297330496008, -23.76421018344883862, -6.712234129069530653 ) ) ;
#18275=CARTESIAN_POINT ( 'NONE',  ( 16.61895836664333714, 12.92996417114949459, -24.37923977068471970 ) ) ;
#18276=CARTESIAN_POINT ( 'NONE',  ( 13.12592325053682174, 31.71798720882053502, -5.454496241009516133 ) ) ;
#18278=CARTESIAN_POINT ( 'NONE',  ( -21.81785358434161637, 11.77199115278586028, -5.482921482795456214 ) ) ;
#18280=CARTESIAN_POINT ( 'NONE',  ( 13.12731182914002659, -23.09957666458869951, -15.43892246686051095 ) ) ;
#18282=CARTESIAN_POINT ( 'NONE',  ( 13.47223693944937750, 18.09844039693851769, -21.24786896499729139 ) ) ;
#18284=CARTESIAN_POINT ( 'NONE',  ( -13.47489597303660069, 22.84936685448861482, -15.44687488758540717 ) ) ;
#18286=CARTESIAN_POINT ( 'NONE',  ( -24.97569650337160496, -26.32149808972361527, -5.444941899105278260 ) ) ;
#18287=CARTESIAN_POINT ( 'NONE',  ( 10.76261159742561802, -25.66954346325781700, -5.000000000000002665 ) ) ;
#18292=CARTESIAN_POINT ( 'NONE',  ( -9.771457654459068110, 32.72495824132072784, -10.28232596613767669 ) ) ;
#18298=CARTESIAN_POINT ( 'NONE',  ( 30.15129433585467567, 0.04742302619024474364, -8.768128520917576552 ) ) ;
#18299=CARTESIAN_POINT ( 'NONE',  ( 3.465511072935331782, 38.21601825462830249, -4.999999999999999112 ) ) ;
#18303=CARTESIAN_POINT ( 'NONE',  ( -29.79738327385628693, 0.04873725983771388937, -9.709267053127604186 ) ) ;
#18306=CARTESIAN_POINT ( 'NONE',  ( 33.87848217329536027, -7.057063397675949368, -8.961058107038109455 ) ) ;
#18310=DIRECTION ( 'NONE',  ( 1.000000000000000000, 0.000000000000000000, 0.000000000000000000 ) ) ;
#18317=FACE_OUTER_BOUND ( 'NONE', #33782, .T. ) ;
#18318=CARTESIAN_POINT ( 'NONE',  ( 7.070389571528393979, 36.44087030134537741, -7.144592491976538007 ) ) ;
#18321=CARTESIAN_POINT ( 'NONE',  ( 17.92107859924769286, -26.25758313345151507, -9.565594702903538860 ) ) ;
#18326=CARTESIAN_POINT ( 'NONE',  ( -11.28570022020756092, 17.50099206051545053, -26.84538423779353167 ) ) ;
#18329=CARTESIAN_POINT ( 'NONE',  ( 10.99009283189107222, -20.50363791108294720, -20.56400601000566297 ) ) ;
#18334=CARTESIAN_POINT ( 'NONE',  ( -14.41188954600920624, 29.53590640632083719, -5.462209281689084150 ) ) ;
#18335=CARTESIAN_POINT ( 'NONE',  ( -17.98125570054222067, -25.38052975340228556, -11.37714725492202028 ) ) ;
#18336=CARTESIAN_POINT ( 'NONE',  ( 6.023418944065099367, 39.81932404830325112, -4.999999999999995559 ) ) ;
#18338=EDGE_CURVE ( 'NONE', #7027, #23669, #34827, .T. ) ;
#18339=CARTESIAN_POINT ( 'NONE',  ( -22.42412062115972660, -6.996450698531886836, -21.99081150208999702 ) ) ;
#18341=CARTESIAN_POINT ( 'NONE',  ( -10.95620176796833611, -20.50974478584956628, -20.56786716869152798 ) ) ;
#18345=CARTESIAN_POINT ( 'NONE',  ( 20.62687364291603487, 1.714078824949687441, -27.50299618919958178 ) ) ;
#18349=CARTESIAN_POINT ( 'NONE',  ( -30.86467312755451076, -0.1056312804566766766, -6.415435717435306273 ) ) ;
#18351=CARTESIAN_POINT ( 'NONE',  ( 24.87279611354669484, -0.2351948277588876701, -18.36342014254012156 ) ) ;
#18356=CARTESIAN_POINT ( 'NONE',  ( -27.15297274608521505, 3.518273904157881660, -8.818013410083365144 ) ) ;
#18367=VERTEX_POINT ( 'NONE', #19531 ) ;
#18368=CARTESIAN_POINT ( 'NONE',  ( -19.48816862725384169, 6.402609444000542993, -30.00000000000000355 ) ) ;
#18371=CARTESIAN_POINT ( 'NONE',  ( 14.60836822939834434, -16.15617325942540106, -24.48969730763191066 ) ) ;
#18374=CARTESIAN_POINT ( 'NONE',  ( 13.34594308816744324, 23.10805189355821554, -15.41729477589293928 ) ) ;
#18377=CARTESIAN_POINT ( 'NONE',  ( -16.15419993190558401, 23.97630781949517598, -6.895672015151252054 ) ) ;
#18380=CIRCLE ( 'NONE', #23571, 17.00000000000000000 ) ;
#18382=CARTESIAN_POINT ( 'NONE',  ( 11.00415319253780488, 17.29620292487934563, -29.34878042274528198 ) ) ;
#18386=CARTESIAN_POINT ( 'NONE',  ( -15.33616239741719234, 27.06134930142311745, -5.472843250504300094 ) ) ;
#18388=CARTESIAN_POINT ( 'NONE',  ( -9.670677759005913643, -18.31648422485758232, -27.44423000158573700 ) ) ;
#18391=CARTESIAN_POINT ( 'NONE',  ( -19.55581111739057931, -11.80372462897835817, -22.98306217881111380 ) ) ;
#18392=CARTESIAN_POINT ( 'NONE',  ( -13.18739005314428248, -25.19688251061680617, -10.68449307879287780 ) ) ;
#18394=CARTESIAN_POINT ( 'NONE',  ( 16.02269691061813006, 23.35602331712748025, -8.798133084021126038 ) ) ;
#18396=CARTESIAN_POINT ( 'NONE',  ( 24.81717070478679688, 5.495116086519474585, -11.78307908032107854 ) ) ;
#18397=FACE_OUTER_BOUND ( 'NONE', #36826, .T. ) ;
#18401=CARTESIAN_POINT ( 'NONE',  ( -31.94197113782983877, -1.240068278442397531, -5.930863948769548699 ) ) ;
#18403=CARTESIAN_POINT ( 'NONE',  ( 30.24433606442397959, -0.05178948828996779441, -8.764081122583004202 ) ) ;
#18407=EDGE_LOOP ( 'NONE', ( #38172, #33584, #18854, #19033, #8621, #14249 ) ) ;
#18417=CARTESIAN_POINT ( 'NONE',  ( 1.910055380441378681, 26.73820970956909449, -18.62404870119007327 ) ) ;
#18424=CARTESIAN_POINT ( 'NONE',  ( 14.30852138182742728, 26.56022758966166109, -10.58015527044261894 ) ) ;
#18427=CARTESIAN_POINT ( 'NONE',  ( -17.91835549149922713, 18.20411370326764811, -9.837959905343433675 ) ) ;
#18431=CARTESIAN_POINT ( 'NONE',  ( 11.90604067169677904, -21.48480776871750209, -18.45226974073501580 ) ) ;
#18432=CARTESIAN_POINT ( 'NONE',  ( -16.57032929827895273, -22.18377021195244936, -16.08031649169519994 ) ) ;
#18433=CARTESIAN_POINT ( 'NONE',  ( 15.01833821314311379, 25.96818848446423189, -9.238322678839528734 ) ) ;
#18434=CARTESIAN_POINT ( 'NONE',  ( 14.83401637327768618, 25.62822920609098176, -10.17906930079575112 ) ) ;
#18438=CARTESIAN_POINT ( 'NONE',  ( -9.450798935534860945, -18.19154675410751310, -30.00000000000000000 ) ) ;
#18441=CARTESIAN_POINT ( 'NONE',  ( -28.36389015409294601, -22.24485741755683677, -9.748513342677570748 ) ) ;
#18442=CARTESIAN_POINT ( 'NONE',  ( 1.575182151896790339, -22.97049887755249031, -15.95023905627559024 ) ) ;
#18443=CARTESIAN_POINT ( 'NONE',  ( 11.31999918839495933, 17.23783125480536782, -28.09381573830394174 ) ) ;
#18444=CARTESIAN_POINT ( 'NONE',  ( 21.17511726572084285, 11.79403841473552461, -10.38720750812251481 ) ) ;
#18447=CARTESIAN_POINT ( 'NONE',  ( -5.177819697455928072, 36.33475957580800042, -8.863124948621987187 ) ) ;
#18449=CARTESIAN_POINT ( 'NONE',  ( -25.16898798258920777, -3.892907297832375324, -19.00733652691929265 ) ) ;
#18454=CARTESIAN_POINT ( 'NONE',  ( -24.28611727277358412, 1.006298860692754316, -18.51342557011203738 ) ) ;
#18455=CARTESIAN_POINT ( 'NONE',  ( 34.22374188224875979, -12.56921889987730800, -8.873390837788807772 ) ) ;
#18467=CARTESIAN_POINT ( 'NONE',  ( -1.624100677291492101, 20.43571491435562493, -29.21538960015010034 ) ) ;
#18472=CARTESIAN_POINT ( 'NONE',  ( 28.65116837111353476, -23.44305233603574123, -7.996273562022556902 ) ) ;
#18473=CARTESIAN_POINT ( 'NONE',  ( 16.00867692525036290, 13.39373376902821278, -25.45607993003914871 ) ) ;
#18474=CARTESIAN_POINT ( 'NONE',  ( 8.790171551589970989, 18.84476076792456567, -27.27665836229843777 ) ) ;
#18477=CARTESIAN_POINT ( 'NONE',  ( -21.15630055661832287, 12.66096790527163485, -7.428688768124617425 ) ) ;
#18479=CARTESIAN_POINT ( 'NONE',  ( 12.75462202092051101, -22.56042021202167547, -16.43275011361073368 ) ) ;
#18481=CARTESIAN_POINT ( 'NONE',  ( 1.354211015180573125E-14, -26.63027081345975589, -13.39439507595156265 ) ) ;
#18482=CARTESIAN_POINT ( 'NONE',  ( -14.92500765838162735, 25.83139737525633706, -9.707172920663500904 ) ) ;
#18483=CARTESIAN_POINT ( 'NONE',  ( -16.46163937660932675, -19.62796718106372751, -18.96315420958638143 ) ) ;
#18484=CARTESIAN_POINT ( 'NONE',  ( 13.11109743797562466, -26.17839091903269733, -5.474232844414386179 ) ) ;
#18490=CARTESIAN_POINT ( 'NONE',  ( -9.875490294415444126, 29.82293549085830264, -13.06707053424541520 ) ) ;
#18496=CARTESIAN_POINT ( 'NONE',  ( 29.35229056070877718, 0.07664280817823312941, -10.65354559736987383 ) ) ;
#18497=CARTESIAN_POINT ( 'NONE',  ( -6.749995343096113487, 37.10960504752362255, -4.999999999999997335 ) ) ;
#18501=CARTESIAN_POINT ( 'NONE',  ( -23.91902260382858714, 0.5374607429489602906, -19.50238920718228641 ) ) ;
#18504=CARTESIAN_POINT ( 'NONE',  ( 22.03414195915153684, -3.843093978875791628, -23.35154269917405756 ) ) ;
#18519=CARTESIAN_POINT ( 'NONE',  ( 7.047533809553444328, 27.34333616107158349, -16.78122118766336257 ) ) ;
#18521=CARTESIAN_POINT ( 'NONE',  ( 18.05419321018431589, -26.43384140100978641, -9.107442122467894308 ) ) ;
#18522=DIRECTION ( 'NONE',  ( 1.000000000000000000, 0.000000000000000000, 0.000000000000000000 ) ) ;
#18523=VECTOR ( 'NONE', #28358, 1000.000000000000000 ) ;
#18527=CARTESIAN_POINT ( 'NONE',  ( -15.43019833371434579, 26.73233873233005653, -5.000000000000002665 ) ) ;
#18530=CARTESIAN_POINT ( 'NONE',  ( 14.95787899955085543, -26.32395102021559197, -7.829361611777857277 ) ) ;
#18533=ORIENTED_EDGE ( 'NONE', *, *, #5935, .F. ) ;
#18535=CARTESIAN_POINT ( 'NONE',  ( -12.50895407495804434, 23.45396610927918957, -16.29466274982731733 ) ) ;
#18536=CARTESIAN_POINT ( 'NONE',  ( -20.24725042846177203, -26.82317351284016027, -7.696457707553546967 ) ) ;
#18540=CARTESIAN_POINT ( 'NONE',  ( -19.78566680745120365, -6.173659883245491642, -27.77246204399593665 ) ) ;
#18541=CARTESIAN_POINT ( 'NONE',  ( -10.62033910827488725, -20.04172040370476537, -21.64366540849149700 ) ) ;
#18544=CARTESIAN_POINT ( 'NONE',  ( 23.24001508372326441, 0.7665741418457661105, -20.56782922800247704 ) ) ;
#18548=CARTESIAN_POINT ( 'NONE',  ( -28.37955323983597467, 0.09052745480185327154, -12.54540266281936844 ) ) ;
#18550=CARTESIAN_POINT ( 'NONE',  ( 21.89958531435420497, -0.4341651203043321861, -23.71319811986195703 ) ) ;
#18551=CARTESIAN_POINT ( 'NONE',  ( -0.2953921336507466799, -20.50164038595707439, -29.99999999999999645 ) ) ;
#18554=CARTESIAN_POINT ( 'NONE',  ( -27.86048499494648567, 2.636343818125510108, -8.804713555145298187 ) ) ;
#18568=CARTESIAN_POINT ( 'NONE',  ( -24.63660806518388924, 7.092056224046558555, -7.894412173378091424 ) ) ;
#18571=CARTESIAN_POINT ( 'NONE',  ( 16.18034479685473670, -16.82698281147069252, -22.08061376403061971 ) ) ;
#18573=CARTESIAN_POINT ( 'NONE',  ( 11.31663199219571148, 18.58087735513076666, -23.82738904643892397 ) ) ;
#18575=CARTESIAN_POINT ( 'NONE',  ( -15.87128850075231590, 24.35504432729732471, -7.840557014529688118 ) ) ;
#18578=CARTESIAN_POINT ( 'NONE',  ( 11.02183263331336072, 17.28494426090127334, -29.34916159435818273 ) ) ;
#18584=CARTESIAN_POINT ( 'NONE',  ( -10.95724656110390960, 17.57990422145660503, -27.43878361132108878 ) ) ;
#18587=CARTESIAN_POINT ( 'NONE',  ( -14.18625507368043159, -24.63497049750179357, -12.53935437351460003 ) ) ;
#18592=CARTESIAN_POINT ( 'NONE',  ( -18.66148164344931004, -9.085586588243005579, -27.71109438505605738 ) ) ;
#18593=CARTESIAN_POINT ( 'NONE',  ( -10.80975121954417695, -21.57342429178983068, -18.55613864020834214 ) ) ;
#18595=CARTESIAN_POINT ( 'NONE',  ( 15.94824334694384582, 24.12454408679510820, -7.842198151814580243 ) ) ;
#18597=CARTESIAN_POINT ( 'NONE',  ( 26.43854853772318947, 4.666896068008411724, -7.871277590448321426 ) ) ;
#18601=CARTESIAN_POINT ( 'NONE',  ( -17.08966005440910507, -22.85233455234303079, -15.10154554898533874 ) ) ;
#18603=CARTESIAN_POINT ( 'NONE',  ( -31.18229473435558319, -0.3319675162687183989, -4.999999999999999112 ) ) ;
#18604=CARTESIAN_POINT ( 'NONE',  ( 30.03507885031549662, -0.2128173951707619527, -9.691532691046774062 ) ) ;
#18608=CARTESIAN_POINT ( 'NONE',  ( 22.52744239175980567, -0.1803094636422790109, -30.00000000000000000 ) ) ;
#18618=CARTESIAN_POINT ( 'NONE',  ( 2.734349871686851507, 38.15652731944587828, -6.277973080134718664 ) ) ;
#18625=CARTESIAN_POINT ( 'NONE',  ( 13.28887463864177043, 24.39605242036939714, -14.37461945989296552 ) ) ;
#18628=CARTESIAN_POINT ( 'NONE',  ( -16.90813000154546231, 15.39385669201410423, -17.92356762543468562 ) ) ;
#18631=CARTESIAN_POINT ( 'NONE',  ( 15.23417145244625281, -26.39024772874911307, -7.827869052557821838 ) ) ;
#18632=CARTESIAN_POINT ( 'NONE',  ( -12.63282099796252034, -16.15870876741617579, -30.00000000000001066 ) ) ;
#18633=DIRECTION ( 'NONE',  ( 0.000000000000000000, 0.000000000000000000, 1.000000000000000000 ) ) ;
#18634=CARTESIAN_POINT ( 'NONE',  ( 11.05947062229327926, 17.51160466381875835, -27.44674441618432326 ) ) ;
#18637=CARTESIAN_POINT ( 'NONE',  ( -14.75295324041043799, -25.80753188146049482, -9.710811175497244818 ) ) ;
#18639=CARTESIAN_POINT ( 'NONE',  ( -18.13230426550196839, -12.48663698560311275, -24.23425696877543700 ) ) ;
#18640=CARTESIAN_POINT ( 'NONE',  ( -0.2861739033633732832, -21.20374024808155156, -23.33089809976452500 ) ) ;
#18641=CARTESIAN_POINT ( 'NONE',  ( 14.23250866199382436, 23.46649709690858643, -13.53614068862031061 ) ) ;
#18642=CARTESIAN_POINT ( 'NONE',  ( 22.42968607831754113, 10.03218932006194386, -9.389054437147178689 ) ) ;
#18644=CARTESIAN_POINT ( 'NONE',  ( -3.836448945760380536, 22.38753517863213816, -23.07412469210595773 ) ) ;
#18645=VERTEX_POINT ( 'NONE', #38828 ) ;
#18646=CARTESIAN_POINT ( 'NONE',  ( -27.06678414647392117, -5.014901417910227366, -16.91862960005362382 ) ) ;
#18654=CARTESIAN_POINT ( 'NONE',  ( -25.51179355227999679, 0.9159808143456273921, -16.49580793394636302 ) ) ;
#18655=CARTESIAN_POINT ( 'NONE',  ( 22.98695121338641201, -8.481255122890857479, -20.78017015740226725 ) ) ;
#18664=CARTESIAN_POINT ( 'NONE',  ( -4.032443027607593322, 36.05064863044662360, -9.738485491014769124 ) ) ;
#18668=CARTESIAN_POINT ( 'NONE',  ( 17.44545305909492683, -13.38241287727507256, -24.26558710457006285 ) ) ;
#18669=CARTESIAN_POINT ( 'NONE',  ( 16.23943293897244544, 12.53170227796935343, -30.00000000000000355 ) ) ;
#18671=CARTESIAN_POINT ( 'NONE',  ( 11.98794441292618984, 28.67068012064173388, -12.24360472531066968 ) ) ;
#18674=CARTESIAN_POINT ( 'NONE',  ( -20.80119427603082016, 12.44190052851605444, -10.38726145399924050 ) ) ;
#18676=CARTESIAN_POINT ( 'NONE',  ( 15.68314276670921359, -26.79173994879206688, -5.473249617827911528 ) ) ;
#18677=LINE ( 'NONE', #12573, #6121 ) ;
#18679=CARTESIAN_POINT ( 'NONE',  ( -5.636483973512888213, -22.01575377102104625, -29.99999999999999645 ) ) ;
#18682=CARTESIAN_POINT ( 'NONE',  ( -15.15864152013962673, 26.33530742007706138, -8.295770841832171172 ) ) ;
#18683=CARTESIAN_POINT ( 'NONE',  ( -13.12770624849639844, -15.75833046460326692, -30.00000000000001421 ) ) ;
#18684=CARTESIAN_POINT ( 'NONE',  ( 10.69843551445597463, -25.55873913893780269, -6.902590252133971482 ) ) ;
#18688=CARTESIAN_POINT ( 'NONE',  ( -6.721507432170120033, 20.19422004900923895, -25.81187786869902112 ) ) ;
#18693=CARTESIAN_POINT ( 'NONE',  ( 30.89317523684279010, -0.03095884371312801128, -5.474201754116363006 ) ) ;
#18699=CARTESIAN_POINT ( 'NONE',  ( -23.30556412954694778, 0.5841231897993812705, -20.54594922719505234 ) ) ;
#18702=CARTESIAN_POINT ( 'NONE',  ( 28.84037157294331521, -5.093697924006990618, -14.99084036193530345 ) ) ;
#18707=CIRCLE ( 'NONE', #1190, 16.00000000000000000 ) ;
#18720=CARTESIAN_POINT ( 'NONE',  ( 6.275750612750602642, 24.42035190817285795, -19.81826795694746224 ) ) ;
#18721=CARTESIAN_POINT ( 'NONE',  ( 11.21453531681511784, -17.17359087135386631, -29.31171484545407324 ) ) ;
#18722=DIRECTION ( 'NONE',  ( -0.000000000000000000, -0.000000000000000000, 1.000000000000000000 ) ) ;
#18726=CARTESIAN_POINT ( 'NONE',  ( -12.67439586582248268, 21.02274553044240690, -18.45589385857095266 ) ) ;
#18729=CARTESIAN_POINT ( 'NONE',  ( 15.08885268118981493, -26.51893482596228679, -6.888510563021540634 ) ) ;
#18734=CARTESIAN_POINT ( 'NONE',  ( -10.57894702805681320, 19.19023191218746049, -23.71264430011183677 ) ) ;
#18735=CARTESIAN_POINT ( 'NONE',  ( -11.63857182560571069, -18.06026089823302883, -24.81603628889719815 ) ) ;
#18739=CARTESIAN_POINT ( 'NONE',  ( -20.89731588449937050, -6.521350128711503658, -24.35897028945197107 ) ) ;
#18740=CARTESIAN_POINT ( 'NONE',  ( -11.05277117942599929, -20.49230150080012436, -20.55679038895522481 ) ) ;
#18743=CARTESIAN_POINT ( 'NONE',  ( 26.35681613863516048, 0.5053618088134171904, -15.46827064861124512 ) ) ;
#18748=CARTESIAN_POINT ( 'NONE',  ( -20.48364860518192998, 0.8189024673161406920, -30.00000000000000000 ) ) ;
#18750=CARTESIAN_POINT ( 'NONE',  ( 25.24172059964007175, -1.134046536396660310, -18.25343667544089499 ) ) ;
#18751=CARTESIAN_POINT ( 'NONE',  ( 17.12152044068272971, -11.27946124554793883, -30.00000000000003553 ) ) ;
#18754=CARTESIAN_POINT ( 'NONE',  ( -26.44546049722394798, 4.400203990190252767, -8.831313265021430325 ) ) ;
#18763=CARTESIAN_POINT ( 'NONE',  ( -30.90412082983564446, -0.04211290444597337590, -5.000000000000000888 ) ) ;
#18765=CARTESIAN_POINT ( 'NONE',  ( -23.22194232212845577, 6.892050143596356371, -13.82897816699491678 ) ) ;
#18768=CARTESIAN_POINT ( 'NONE',  ( 21.28768541942379144, -24.85472925722318749, -11.24091203251788684 ) ) ;
#18770=CARTESIAN_POINT ( 'NONE',  ( 14.18431540342452912, 24.75056589267492058, -12.52692153250820617 ) ) ;
#18772=CARTESIAN_POINT ( 'NONE',  ( -15.01220060599063189, 22.71241345319973348, -12.61924114651307960 ) ) ;
#18775=CARTESIAN_POINT ( 'NONE',  ( 11.33221106479448714, 18.02071959632803910, -25.01755605303010555 ) ) ;
#18779=CARTESIAN_POINT ( 'NONE',  ( -10.83390719878747355, 17.40340976726015398, -29.99999999999999289 ) ) ;
#18781=CARTESIAN_POINT ( 'NONE',  ( -15.70264670462719714, -26.79635097760029794, -5.000000000000000888 ) ) ;
#18786=CARTESIAN_POINT ( 'NONE',  ( -25.09485740259016850, -12.19075756865849947, -17.60690265804054278 ) ) ;
#18787=CARTESIAN_POINT ( 'NONE',  ( -11.29805317986360258, -25.35288615261349676, -8.807478906485194159 ) ) ;
#18789=CARTESIAN_POINT ( 'NONE',  ( 14.35723387269807461, 20.24307895078839792, -16.61037614182657052 ) ) ;
#18792=CARTESIAN_POINT ( 'NONE',  ( 25.84550903417051160, 5.566988420567247076, -7.396971983680807661 ) ) ;
#18799=CARTESIAN_POINT ( 'NONE',  ( -30.61729485247184002, -0.2875646607849730585, -8.283315588427790033 ) ) ;
#18800=CARTESIAN_POINT ( 'NONE',  ( 20.83381800968227182, 0.6014786412957214834, -26.81279315949302955 ) ) ;
#18804=CARTESIAN_POINT ( 'NONE',  ( 8.937590682902566641, -20.71651963383554218, -21.24786896499729494 ) ) ;
#18812=CARTESIAN_POINT ( 'NONE',  ( 37.28744356507513658, -7.587582650827097375, -5.000000000000016875 ) ) ;
#18813=CARTESIAN_POINT ( 'NONE',  ( 1.444440266932477623, 20.45847851156178265, -29.21425697047676451 ) ) ;
#18821=CARTESIAN_POINT ( 'NONE',  ( 10.13018406787138304, 17.82246755199521360, -29.33001752643188453 ) ) ;
#18824=CARTESIAN_POINT ( 'NONE',  ( -18.04083112182678406, 18.37157263296915133, -8.860390942907290679 ) ) ;
#18827=CARTESIAN_POINT ( 'NONE',  ( 10.84768000140452848, -19.98809413286245018, -21.61592137937718761 ) ) ;
#18828=CARTESIAN_POINT ( 'NONE',  ( -21.44652559126361879, -26.87240656024164664, -7.228200811290371952 ) ) ;
#18829=CARTESIAN_POINT ( 'NONE',  ( 14.29473281614541946, 24.46189118728469225, -12.55068749070381884 ) ) ;
#18830=CARTESIAN_POINT ( 'NONE',  ( 14.52401956015651230, 24.99458846522630751, -11.59728651514169684 ) ) ;
#18833=CARTESIAN_POINT ( 'NONE',  ( -14.78861890278166413, -25.81514123692260299, -9.710278502422099223 ) ) ;
#18836=CARTESIAN_POINT ( 'NONE',  ( -20.30545432580447240, -13.99291260258515379, -20.70863365825785962 ) ) ;
#18837=CARTESIAN_POINT ( 'NONE',  ( -2.563881278962895749, -24.61887866671625247, -7.916840171043283192 ) ) ;
#18838=CARTESIAN_POINT ( 'NONE',  ( 15.21168623108442475, 24.52100632137278069, -10.20105120338589622 ) ) ;
#18840=CARTESIAN_POINT ( 'NONE',  ( 18.89612423569448296, 9.643090400953798991, -23.32574488315787065 ) ) ;
#18843=CARTESIAN_POINT ( 'NONE',  ( -33.03352659232529476, -3.420569429262189765, -7.712445482004824271 ) ) ;
#18849=CARTESIAN_POINT ( 'NONE',  ( -20.65398372803566573, 1.346249621251496054, -27.47960346742159743 ) ) ;
#18850=CARTESIAN_POINT ( 'NONE',  ( 19.23659220497393108, -7.112289578705963677, -29.22637812988511641 ) ) ;
#18853=DIRECTION ( 'NONE',  ( -1.000000000000000000, 0.000000000000000000, 0.000000000000000000 ) ) ;
#18854=ORIENTED_EDGE ( 'NONE', *, *, #15113, .F. ) ;
#18861=CARTESIAN_POINT ( 'NONE',  ( -2.050360002403428972, 25.60080579252921495, -19.64802405917689754 ) ) ;
#18868=CARTESIAN_POINT ( 'NONE',  ( 14.23294558246579022, 29.80882899807581055, -4.999999999999997335 ) ) ;
#18870=CARTESIAN_POINT ( 'NONE',  ( -21.06328208572556093, 12.60356320803115970, -8.409244101891895085 ) ) ;
#18872=CARTESIAN_POINT ( 'NONE',  ( 14.22674418391079243, -24.64141992797763336, -12.53611091602331662 ) ) ;
#18875=CARTESIAN_POINT ( 'NONE',  ( 14.90698185259310016, 25.88873565208333005, -9.704017660486000452 ) ) ;
#18876=CARTESIAN_POINT ( 'NONE',  ( 8.937590682902566641, -20.71651963383554218, -30.00000000000000000 ) ) ;
#18878=CARTESIAN_POINT ( 'NONE',  ( -15.45681155788697936, -16.36624024623564111, -23.23867721921044804 ) ) ;
#18879=CARTESIAN_POINT ( 'NONE',  ( 10.50810896484892254, -25.22781171335135042, -8.817308065532962758 ) ) ;
#18880=CARTESIAN_POINT ( 'NONE',  ( 12.19824770565493566, 19.84438704282505839, -20.55290514491795406 ) ) ;
#18882=CARTESIAN_POINT ( 'NONE',  ( 17.05875634882093195, -11.52365334420840881, -28.44935981325557250 ) ) ;
#18886=CARTESIAN_POINT ( 'NONE',  ( -10.90236520000052245, 33.11211960170862767, -8.515142989435695142 ) ) ;
#18891=CARTESIAN_POINT ( 'NONE',  ( 20.81362228500634970, 0.8536333317955857591, -26.83237868093558731 ) ) ;
#18895=CARTESIAN_POINT ( 'NONE',  ( -27.71741899510553608, 0.2170695715558252636, -13.51503484893205531 ) ) ;
#18898=CARTESIAN_POINT ( 'NONE',  ( 20.21125490546006276, -3.489748019849370220, -29.27149083989724687 ) ) ;
#18909=CARTESIAN_POINT ( 'NONE',  ( -19.61636114005775511, 5.963768710578694510, -30.00000000000001776 ) ) ;
#18913=CARTESIAN_POINT ( 'NONE',  ( 17.34393471781637075, 19.49149365859844352, -9.816462853724280180 ) ) ;
#18914=CARTESIAN_POINT ( 'NONE',  ( 9.500382936455952887, 32.89299068974253260, -10.27676952640711505 ) ) ;
#18918=CARTESIAN_POINT ( 'NONE',  ( 16.58821223849002635, -25.78030334186819772, -10.53774966371608279 ) ) ;
#18922=CARTESIAN_POINT ( 'NONE',  ( -11.46775114909779880, 17.91482654455204937, -25.03573280478206797 ) ) ;
#18924=CARTESIAN_POINT ( 'NONE',  ( 12.17258182436908065, -22.02639489287507502, -17.44778068929893067 ) ) ;
#18929=CARTESIAN_POINT ( 'NONE',  ( -13.49361715555115282, 27.40176124217998321, -11.42939491410920994 ) ) ;
#18930=CARTESIAN_POINT ( 'NONE',  ( -11.98442307596994816, -17.42517490280342329, -26.00811570201611289 ) ) ;
#18933=CARTESIAN_POINT ( 'NONE',  ( -21.06133918572757224, -5.879866026727245121, -24.39648093831449671 ) ) ;
#18934=CARTESIAN_POINT ( 'NONE',  ( -12.16148876965757530, -22.02675247291305283, -17.44874281179136943 ) ) ;
#18937=CARTESIAN_POINT ( 'NONE',  ( 26.41552486178371950, 1.278391022459212545, -14.54603937267712332 ) ) ;
#18942=CARTESIAN_POINT ( 'NONE',  ( -20.97406219683946915, 0.7643328109957392424, -26.22104410486783976 ) ) ;
#18944=CARTESIAN_POINT ( 'NONE',  ( 23.71077850922558738, -0.6311408168542613772, -20.38398171457574293 ) ) ;
#18945=CARTESIAN_POINT ( 'NONE',  ( 19.42600269443267891, -6.688926838600538716, -30.00000000000002842 ) ) ;
#18948=CARTESIAN_POINT ( 'NONE',  ( -21.52205650746854815, 4.298041411267772283, -21.99797594555649383 ) ) ;
#18960=CARTESIAN_POINT ( 'NONE',  ( -19.76188599801438173, 5.707498807444228106, -28.24951685685252656 ) ) ;
#18963=CARTESIAN_POINT ( 'NONE',  ( 19.41504592165321696, -20.20693249214978238, -16.82202162988696514 ) ) ;
#18965=CARTESIAN_POINT ( 'NONE',  ( 10.94815433824005169, 17.73468434523852721, -26.81376961522255087 ) ) ;
#18967=CARTESIAN_POINT ( 'NONE',  ( -15.96668161688104703, 24.53857560187668696, -6.893541485189635942 ) ) ;
#18971=CARTESIAN_POINT ( 'NONE',  ( 11.02183263331336072, 17.28494426090127334, -30.00000000000000000 ) ) ;
#18975=CARTESIAN_POINT ( 'NONE',  ( -15.09256969434682460, 26.55329248168451883, -8.287362166344871994 ) ) ;
#18977=CARTESIAN_POINT ( 'NONE',  ( -9.607720528598306942, -18.16065568266596841, -28.70352573344614910 ) ) ;
#18980=CARTESIAN_POINT ( 'NONE',  ( -19.27656959047015306, -9.383399175354611543, -25.58674328688679722 ) ) ;
#18981=CARTESIAN_POINT ( 'NONE',  ( -11.92233111337420048, -22.55166628322649558, -16.49877645844951246 ) ) ;
#18983=CARTESIAN_POINT ( 'NONE',  ( 12.56326696322676639, 16.68910371357088351, -26.36019947833989718 ) ) ;
#18985=CARTESIAN_POINT ( 'NONE',  ( 22.21757360568209094, 4.531282118560625349, -19.88525668396988877 ) ) ;
#18990=CARTESIAN_POINT ( 'NONE',  ( -12.11431921993760952, -16.53859995959433604, -28.58492679012440618 ) ) ;
#18992=CARTESIAN_POINT ( 'NONE',  ( -20.64150323923506747, 0.1775972471279622378, -28.04374465433520314 ) ) ;
#18993=CARTESIAN_POINT ( 'NONE',  ( 30.67384541073807114, -0.3508467513185977715, -8.280288242715185376 ) ) ;
#18997=CARTESIAN_POINT ( 'NONE',  ( 2.168404344971008868E-14, -26.63027081345975589, -4.999999999999999112 ) ) ;
#19001=EDGE_CURVE ( 'NONE', #14160, #40031, #2592, .T. ) ;
#19004=CARTESIAN_POINT ( 'NONE',  ( 27.20167217099651680, 3.999461679709010564, -5.000000000000004441 ) ) ;
#19005=CARTESIAN_POINT ( 'NONE',  ( 2.248380420413196301, 31.20224717405769965, -14.73880478081109224 ) ) ;
#19008=AXIS2_PLACEMENT_3D ( 'NONE', #31363, #9233, #15131 ) ;
#19013=CARTESIAN_POINT ( 'NONE',  ( 10.42368143308724093, 18.08059978384341449, -26.76484793057170819 ) ) ;
#19017=CARTESIAN_POINT ( 'NONE',  ( -18.13727770824980823, 18.50383905080510161, -7.888881962196643727 ) ) ;
#19020=CARTESIAN_POINT ( 'NONE',  ( 15.35224999201118301, -26.63338943820685145, -6.417067792862570563 ) ) ;
#19021=CARTESIAN_POINT ( 'NONE',  ( -14.68365521139617513, -18.63605605981938496, -21.13871917996053540 ) ) ;
#19022=CARTESIAN_POINT ( 'NONE',  ( 15.34221292749994703, 26.60361493431586410, -6.887934399220042359 ) ) ;
#19023=CARTESIAN_POINT ( 'NONE',  ( 15.09678720978786792, 26.15351954639106680, -8.766955913214280471 ) ) ;
#19026=CARTESIAN_POINT ( 'NONE',  ( -12.18907228018264988, -22.02585773758839593, -17.44635340709443128 ) ) ;
#19029=CARTESIAN_POINT ( 'NONE',  ( -17.27544398881353516, -12.67674546857244167, -25.60352082169515242 ) ) ;
#19031=CARTESIAN_POINT ( 'NONE',  ( -4.648451212885357009, -24.43533398093167364, -9.867068457485020261 ) ) ;
#19032=CARTESIAN_POINT ( 'NONE',  ( 11.33961468246317139, 17.07831742606941461, -29.35587556166173684 ) ) ;
#19033=ORIENTED_EDGE ( 'NONE', *, *, #21986, .T. ) ;
#19034=CARTESIAN_POINT ( 'NONE',  ( 18.89829205095695031, 8.796968066745694870, -25.49925083140837501 ) ) ;
#19038=CARTESIAN_POINT ( 'NONE',  ( -25.85780729842050008, -3.254098561623225194, -18.03984462349898266 ) ) ;
#19040=AXIS2_PLACEMENT_3D ( 'NONE', #3420, #9528, #15816 ) ;
#19045=CARTESIAN_POINT ( 'NONE',  ( -30.01474851606876726, 0.8478221152901143087, -5.946541633344167188 ) ) ;
#19046=CARTESIAN_POINT ( 'NONE',  ( 34.71864531128215248, -13.96902139200064852, -7.560095839640886162 ) ) ;
#19058=CARTESIAN_POINT ( 'NONE',  ( -1.963563434085775716, 24.56407772697490088, -20.71148629140979125 ) ) ;
#19059=DIRECTION ( 'NONE',  ( 1.000000000000000000, 0.000000000000000000, 0.000000000000000000 ) ) ;
#19065=CARTESIAN_POINT ( 'NONE',  ( 8.342340113773577315, 19.48526559538274228, -25.93911266913574920 ) ) ;
#19068=CARTESIAN_POINT ( 'NONE',  ( -20.15622055155539272, 12.04428324321301425, -13.90711018673853872 ) ) ;
#19070=CARTESIAN_POINT ( 'NONE',  ( 15.43512952755564349, -26.60538963749703356, -6.886851144620130150 ) ) ;
#19072=CARTESIAN_POINT ( 'NONE',  ( 11.02889904915459063, 17.53211054968905813, -27.44436270301952163 ) ) ;
#19073=CARTESIAN_POINT ( 'NONE',  ( -31.47283671532259675, -25.12609584734821411, -5.000000000000010658 ) ) ;
#19074=AXIS2_PLACEMENT_3D ( 'NONE', #9856, #2969, #37690 ) ;
#19075=CARTESIAN_POINT ( 'NONE',  ( -18.50717619730081864, -19.59423608300353692, -17.82256473852398670 ) ) ;
#19076=CARTESIAN_POINT ( 'NONE',  ( 8.329568172293271289, -18.84798106794158201, -28.13937053122434051 ) ) ;
#19077=CARTESIAN_POINT ( 'NONE',  ( 15.29674875102894482, 26.18853547279510607, -7.828964019014474474 ) ) ;
#19078=CARTESIAN_POINT ( 'NONE',  ( 17.19085919694937203, -11.61334556840082399, -27.71234399686709438 ) ) ;
#19082=CARTESIAN_POINT ( 'NONE',  ( -5.372192365448402285, 20.15702040454593913, -27.08516113732625641 ) ) ;
#19089=CARTESIAN_POINT ( 'NONE',  ( 30.65562841553949625, -0.05914043160616395262, -7.356430913030059138 ) ) ;
#19093=CARTESIAN_POINT ( 'NONE',  ( -29.31499521850481216, 0.1194913391831431554, -10.65473379611367655 ) ) ;
#19094=CARTESIAN_POINT ( 'NONE',  ( -19.71199081357663729, -26.17691209550672937, -9.501020233452134534 ) ) ;
#19096=CARTESIAN_POINT ( 'NONE',  ( 21.98133561711489392, -4.524757649539990823, -23.29269831984457184 ) ) ;
#19105=FACE_OUTER_BOUND ( 'NONE', #33950, .T. ) ;
#19109=CARTESIAN_POINT ( 'NONE',  ( 1.087821238877949126, 20.47389780075598509, -30.00000000000000711 ) ) ;
#19112=CARTESIAN_POINT ( 'NONE',  ( 17.57104634348523220, 19.83623530875129148, -7.877413894578867648 ) ) ;
#19113=CARTESIAN_POINT ( 'NONE',  ( 4.967200795408929004, 22.09671430245085944, -23.13287681390427863 ) ) ;
#19115=CARTESIAN_POINT ( 'NONE',  ( 10.16493647378288934, -17.96286526707443798, -28.04375298610375111 ) ) ;
#19120=CARTESIAN_POINT ( 'NONE',  ( -14.74829102090526511, 25.36468816584346087, -10.65391712686787073 ) ) ;
#19122=CARTESIAN_POINT ( 'NONE',  ( 14.94022447862385405, -26.11394648050683998, -8.769034538900596587 ) ) ;
#19126=CARTESIAN_POINT ( 'NONE',  ( -12.20352377363692575, 22.79644703365081071, -17.28398000730053141 ) ) ;
#19128=CARTESIAN_POINT ( 'NONE',  ( -12.15296444596746639, -16.58779297045509438, -28.59925402683893836 ) ) ;
#19131=CARTESIAN_POINT ( 'NONE',  ( -20.30734916839453774, -5.667360972306529021, -26.38649982237350144 ) ) ;
#19132=CARTESIAN_POINT ( 'NONE',  ( -9.488776258477622960, -18.31424688356152330, -28.08193020798964668 ) ) ;
#19135=CARTESIAN_POINT ( 'NONE',  ( 29.99944291653464035, 0.2112700481506303019, -8.770229588436221135 ) ) ;
#19136=CARTESIAN_POINT ( 'NONE',  ( 10.98647152987756748, 17.30743896080529609, -28.69679681820503347 ) ) ;
#19140=CARTESIAN_POINT ( 'NONE',  ( -29.85246077738104731, -0.01121920330367918127, -9.705672615991840502 ) ) ;
#19142=CARTESIAN_POINT ( 'NONE',  ( 30.98664919647288940, -1.692235243981042858, -10.06380571118922518 ) ) ;
#19155=CARTESIAN_POINT ( 'NONE',  ( -22.95459534405085122, 9.880914000425169874, -5.965707660850015692 ) ) ;
#19156=CARTESIAN_POINT ( 'NONE',  ( 14.59364668521135755, -15.19212837545807382, -26.41884767242281384 ) ) ;
#19158=CARTESIAN_POINT ( 'NONE',  ( 14.87809943308360339, 25.97911021677501608, -9.699071928801664910 ) ) ;
#19160=CARTESIAN_POINT ( 'NONE',  ( -15.56594212721577541, 25.60277546647914448, -7.361410068878811330 ) ) ;
#19163=CARTESIAN_POINT ( 'NONE',  ( 15.12327263463977722, 26.06678387642238448, -8.768336635076099839 ) ) ;
#19167=CARTESIAN_POINT ( 'NONE',  ( -14.75774405092634645, 25.86145994709132978, -10.16509986974211976 ) ) ;
#19169=CARTESIAN_POINT ( 'NONE',  ( -9.543759016413366325, -18.14299990126706419, -29.34740481499151343 ) ) ;
#19172=CARTESIAN_POINT ( 'NONE',  ( -25.74471773230272476, -13.48393985794896111, -16.62992022540315062 ) ) ;
#19173=CARTESIAN_POINT ( 'NONE',  ( -13.68829447021390422, -25.58996436347754866, -9.727192414191598857 ) ) ;
#19174=CYLINDRICAL_SURFACE ( 'NONE', #10521, 57.00000000000006395 ) ;
#19175=CARTESIAN_POINT ( 'NONE',  ( 16.87377372029358469, 22.19217076240406428, -5.000000000000004441 ) ) ;
#19177=CARTESIAN_POINT ( 'NONE',  ( 23.39580328310244894, 5.396513899929180624, -15.78908983431174740 ) ) ;
#19185=CARTESIAN_POINT ( 'NONE',  ( -26.97206810645275255, -0.4441396946580338789, -15.36407590373037912 ) ) ;
#19186=CARTESIAN_POINT ( 'NONE',  ( 24.03547544862108154, 0.2628772248198613104, -19.46575558521258387 ) ) ;
#19191=ORIENTED_EDGE ( 'NONE', *, *, #11017, .F. ) ;
#19193=CARTESIAN_POINT ( 'NONE',  ( 5.636483973512839363, -22.01575377102105691, -30.00000000000001421 ) ) ;
#19199=CARTESIAN_POINT ( 'NONE',  ( 2.752814969234745668, 20.95510515482600056, -26.29072956667404171 ) ) ;
#19208=CARTESIAN_POINT ( 'NONE',  ( 15.09735744684384962, 27.15937815847784620, -7.340727882394975978 ) ) ;
#19211=CARTESIAN_POINT ( 'NONE',  ( -17.44085994297563147, 17.55310934480021956, -12.80343249213678547 ) ) ;
#19215=CARTESIAN_POINT ( 'NONE',  ( 15.42968591400663847, -26.70185147947299598, -5.946084178125359720 ) ) ;
#19216=CARTESIAN_POINT ( 'NONE',  ( 17.00000000000000000, 22.50000000000000711, 10.00000000000000000 ) ) ;
#19217=CARTESIAN_POINT ( 'NONE',  ( 15.10684921377551326, 26.12025004395372818, -8.767816402119800401 ) ) ;
#19219=CARTESIAN_POINT ( 'NONE',  ( 15.01137483442351517, 25.99107282686816234, -9.237182367602107647 ) ) ;
#19220=VERTEX_POINT ( 'NONE', #15573 ) ;
#19222=CARTESIAN_POINT ( 'NONE',  ( -10.15894275696289917, -19.18740761933786843, -23.86200704285396768 ) ) ;
#19224=CARTESIAN_POINT ( 'NONE',  ( -28.27972534383151526, -19.54013907706369935, -11.98161375967031717 ) ) ;
#19225=CARTESIAN_POINT ( 'NONE',  ( -4.747314164036073869, -24.73656458911068512, -7.904840398386835609 ) ) ;
#19226=CARTESIAN_POINT ( 'NONE',  ( 11.88480245227968091, 18.08769387689092412, -23.91349747340691678 ) ) ;
#19228=CARTESIAN_POINT ( 'NONE',  ( 20.78437466676830780, 10.47168160296281769, -14.91585341470220349 ) ) ;
#19232=CARTESIAN_POINT ( 'NONE',  ( -29.68610188510462322, -2.963264296338544490, -13.23833758059748966 ) ) ;
#19238=CARTESIAN_POINT ( 'NONE',  ( -20.56034067317128944, 1.524475442768058020, -28.10962306186307913 ) ) ;
#19239=CARTESIAN_POINT ( 'NONE',  ( 34.42547319207020706, -15.07984268493967051, -7.554536495709903932 ) ) ;
#19243=VERTEX_POINT ( 'NONE', #39753 ) ;
#19247=ORIENTED_EDGE ( 'NONE', *, *, #24047, .F. ) ;
#19248=CARTESIAN_POINT ( 'NONE',  ( -0.6412407266015724971, 32.46939045798620072, -13.80435559440418203 ) ) ;
#19255=CARTESIAN_POINT ( 'NONE',  ( 11.69931679021635418, 27.94617659413938782, -13.18484883679364472 ) ) ;
#19258=CARTESIAN_POINT ( 'NONE',  ( -19.02464814996286080, 10.35021103555779476, -21.17776305350152555 ) ) ;
#19261=CARTESIAN_POINT ( 'NONE',  ( 11.59088340238572989, -20.97132811465274926, -19.49109192369429167 ) ) ;
#19263=CARTESIAN_POINT ( 'NONE',  ( 10.96081938953363277, 17.37715277537162351, -28.70507073696821720 ) ) ;
#19264=CARTESIAN_POINT ( 'NONE',  ( 17.81784622497951176, -13.85677843414110555, -19.80438750953540961 ) ) ;
#19265=DIRECTION ( 'NONE',  ( -1.000000000000000000, 0.000000000000000000, 0.000000000000000000 ) ) ;
#19268=CARTESIAN_POINT ( 'NONE',  ( -23.68773345865362856, -25.06554053738202015, -9.830582403723438389 ) ) ;
#19269=CARTESIAN_POINT ( 'NONE',  ( 7.051063895666721315, -19.39164703839861659, -28.19631161156121735 ) ) ;
#19270=CARTESIAN_POINT ( 'NONE',  ( 14.93246635580137038, 25.33278714524708164, -10.18550836669002990 ) ) ;
#19271=CARTESIAN_POINT ( 'NONE',  ( 30.91129473722968157, -20.93446817436120000, -8.409707594405761100 ) ) ;
#19275=CARTESIAN_POINT ( 'NONE',  ( -5.279954849186515808, 19.80786611602342973, -29.99999999999998224 ) ) ;
#19276=AXIS2_PLACEMENT_3D ( 'NONE', #25527, #38529, #16396 ) ;
#19280=VERTEX_POINT ( 'NONE', #21271 ) ;
#19281=CARTESIAN_POINT ( 'NONE',  ( 21.27883545512939634, 0.7584189411604885800, -25.01272306973745074 ) ) ;
#19286=CARTESIAN_POINT ( 'NONE',  ( -30.03482762601120015, 0.1729744975902109405, -8.769734599055784230 ) ) ;
#19289=CARTESIAN_POINT ( 'NONE',  ( 35.19752256302763271, -8.465509976530269043, -5.879991153137873461 ) ) ;
#19304=CIRCLE ( 'NONE', #1807, 62.00000000000002132 ) ;
#19307=CARTESIAN_POINT ( 'NONE',  ( 17.10940565685277193, 17.54728818196264584, -13.79989119490213767 ) ) ;
#19309=CARTESIAN_POINT ( 'NONE',  ( 10.02000509642858361, 34.97447782610390732, -5.444435539378085664 ) ) ;
#19311=CARTESIAN_POINT ( 'NONE',  ( 15.94139939152667829, -26.45195379938700242, -8.269321208413121127 ) ) ;
#19315=CARTESIAN_POINT ( 'NONE',  ( -15.10507689876119564, 26.12566811475226558, -8.768196822005435820 ) ) ;
#19317=CARTESIAN_POINT ( 'NONE',  ( 11.95185560643699318, -22.03370127656497246, -17.46682300787701791 ) ) ;
#19318=CYLINDRICAL_SURFACE ( 'NONE', #8841, 18.00000000000001421 ) ;
#19322=CARTESIAN_POINT ( 'NONE',  ( -12.64160356943281727, 29.64681118489703948, -10.41304400021260612 ) ) ;
#19323=CARTESIAN_POINT ( 'NONE',  ( -13.59760056006964035, -18.39269960460429232, -22.34963270891807952 ) ) ;
#19328=CARTESIAN_POINT ( 'NONE',  ( -34.55393062045996544, -7.546469469217721660, -7.629845520436306927 ) ) ;
#19331=CARTESIAN_POINT ( 'NONE',  ( 20.47688798105681940, 0.9740165025114795316, -30.00000000000000000 ) ) ;
#19337=CARTESIAN_POINT ( 'NONE',  ( -20.48364860518192998, 0.8189024673161406920, -29.34763341778235812 ) ) ;
#19340=CARTESIAN_POINT ( 'NONE',  ( 25.62407562875491962, -2.247368772962396122, -18.13072093081501279 ) ) ;
#19342=CARTESIAN_POINT ( 'NONE',  ( 15.20858617250272005, 13.81569066517950795, -30.00000000000002842 ) ) ;
#19354=CARTESIAN_POINT ( 'NONE',  ( -20.48481815786151827, 8.169629148835463539, -20.07635314567754747 ) ) ;
#19355=CARTESIAN_POINT ( 'NONE',  ( 20.89534821297474565, -25.82708108466523100, -9.908281912035883821 ) ) ;
#19358=CARTESIAN_POINT ( 'NONE',  ( 14.22661425981019256, 24.64141455453919249, -12.53612259479494995 ) ) ;
#19359=ORIENTED_EDGE ( 'NONE', *, *, #17315, .T. ) ;
#19360=CARTESIAN_POINT ( 'NONE',  ( -12.01347213543522585, 16.66139596754671715, -28.74651697924976190 ) ) ;
#19363=CARTESIAN_POINT ( 'NONE',  ( 11.20926058852595908, 17.73831205782239806, -26.22754255443350857 ) ) ;
#19364=ORIENTED_EDGE ( 'NONE', *, *, #32198, .F. ) ;
#19365=CARTESIAN_POINT ( 'NONE',  ( 32.29060608969265900, -17.80231044390160378, -9.282265745321158334 ) ) ;
#19368=CARTESIAN_POINT ( 'NONE',  ( -10.72725030361012521, 17.46952664121795351, -29.99999999999999289 ) ) ;
#19370=CARTESIAN_POINT ( 'NONE',  ( -9.745989649151084677, -18.27917357566746048, -27.43878329331307242 ) ) ;
#19373=CARTESIAN_POINT ( 'NONE',  ( -18.23120227974498420, -9.562336488320314132, -28.44603666067110836 ) ) ;
#19374=CARTESIAN_POINT ( 'NONE',  ( -8.933264501347940367, -18.58110093778079275, -28.11105939349013028 ) ) ;
#19376=CARTESIAN_POINT ( 'NONE',  ( 13.40733656136086616, 18.39885974385108014, -20.74996682341825505 ) ) ;
#19378=CARTESIAN_POINT ( 'NONE',  ( 24.84641422454732407, 2.937850337337710727, -15.64433848410505945 ) ) ;
#19379=DIRECTION ( 'NONE',  ( 1.000000000000000000, 0.000000000000000000, 0.000000000000000000 ) ) ;
#19383=CARTESIAN_POINT ( 'NONE',  ( -31.27312981421062688, -0.4309787749141147928, -5.471709692244465906 ) ) ;
#19384=AXIS2_PLACEMENT_3D ( 'NONE', #35492, #16808, #17009 ) ;
#19385=CARTESIAN_POINT ( 'NONE',  ( 20.70843681679315651, 0.6154661857135520497, -27.43333504746348694 ) ) ;
#19390=CARTESIAN_POINT ( 'NONE',  ( -12.33616729053607486, -27.99489201236593061, -13.58461195433496194 ) ) ;
#19396=CARTESIAN_POINT ( 'NONE',  ( 4.258837352292506928, 31.86736653883517079, -13.83424449677746360 ) ) ;
#19398=EDGE_CURVE ( 'NONE', #3976, #19822, #11724, .T. ) ;
#19399=ORIENTED_EDGE ( 'NONE', *, *, #5365, .F. ) ;
#19402=CARTESIAN_POINT ( 'NONE',  ( 27.24828611745593321, -25.13066665804571542, -6.297441403926967496 ) ) ;
#19405=CARTESIAN_POINT ( 'NONE',  ( 14.69283426033394768, 26.51965037005133752, -9.670188778881371405 ) ) ;
#19408=CARTESIAN_POINT ( 'NONE',  ( -15.72881319288876156, 16.59632136301366856, -18.88276093887042606 ) ) ;
#19412=CARTESIAN_POINT ( 'NONE',  ( 9.476873889470034840, -18.17797724348699973, -29.34878039533210625 ) ) ;
#19415=CARTESIAN_POINT ( 'NONE',  ( 15.29332824945628566, 26.51959359426387763, -7.358051658420890817 ) ) ;
#19417=CARTESIAN_POINT ( 'NONE',  ( 15.23218277980890356, 26.40650644525691249, -7.827771362956440271 ) ) ;
#19421=CARTESIAN_POINT ( 'NONE',  ( -12.35792326267267072, 20.53483958506731710, -19.48932210671636867 ) ) ;
#19423=CARTESIAN_POINT ( 'NONE',  ( -9.495857434766111993, -18.21849447287409518, -28.70794251271205866 ) ) ;
#19425=CARTESIAN_POINT ( 'NONE',  ( -19.54867522336399688, -13.46797132751421167, -21.85517049677807933 ) ) ;
#19426=CARTESIAN_POINT ( 'NONE',  ( -3.274116759621854111, -20.28896347757955354, -29.42369938977917343 ) ) ;
#19427=CARTESIAN_POINT ( 'NONE',  ( 14.33614363210685205, 23.23110485604417619, -13.54771175783602466 ) ) ;
#19429=CARTESIAN_POINT ( 'NONE',  ( 19.78994368857117081, 10.03402965537161329, -19.05768763028667223 ) ) ;
#19433=CARTESIAN_POINT ( 'NONE',  ( -23.42691890934632326, -2.892262406529196195, -21.19212511098400142 ) ) ;
#19435=ORIENTED_EDGE ( 'NONE', *, *, #9638, .T. ) ;
#19439=CARTESIAN_POINT ( 'NONE',  ( 23.47267981164478101, -10.30042122731402543, -19.66540645570583123 ) ) ;
#19443=ORIENTED_EDGE ( 'NONE', *, *, #14464, .T. ) ;
#19449=CARTESIAN_POINT ( 'NONE',  ( -1.909966974610407098, 38.03150725742897720, -7.118504882345924933 ) ) ;
#19456=CARTESIAN_POINT ( 'NONE',  ( 10.13776086571952995, 19.50640881937047055, -23.64984537069171111 ) ) ;
#19459=CARTESIAN_POINT ( 'NONE',  ( -19.63432798946420021, 15.59186056508892904, -6.934370416219701738 ) ) ;
#19462=CARTESIAN_POINT ( 'NONE',  ( 12.69066353061625740, -22.55866965907024735, -16.43980381259239110 ) ) ;
#19463=EDGE_CURVE ( 'NONE', #20607, #39696, #40148, .T. ) ;
#19465=CARTESIAN_POINT ( 'NONE',  ( 14.71862476482751347, 25.45363487584512185, -10.64941651680690349 ) ) ;
#19466=CARTESIAN_POINT ( 'NONE',  ( 2.927345865710861972E-15, 22.57051819516765789, -30.00000000000001421 ) ) ;
#19469=CARTESIAN_POINT ( 'NONE',  ( -15.47784844748352384, -15.42996703057364982, -24.40905844545180159 ) ) ;
#19470=CARTESIAN_POINT ( 'NONE',  ( 6.083101977165589425, -24.65543650029558620, -9.357407788547908112 ) ) ;
#19471=CARTESIAN_POINT ( 'NONE',  ( 15.02539757819879895, 25.52099869179298253, -9.713273572205364914 ) ) ;
#19472=CARTESIAN_POINT ( 'NONE',  ( 24.95130836960470688, -16.89649762504703290, -15.68942752906997029 ) ) ;
#19473=CYLINDRICAL_SURFACE ( 'NONE', #7605, 17.99999999999989697 ) ;
#19477=CARTESIAN_POINT ( 'NONE',  ( -5.944679600751215709, 19.85052517187110510, -27.81791890879877371 ) ) ;
#19480=CARTESIAN_POINT ( 'NONE',  ( 24.57639991767630505, 0.3971110913580137569, -18.44753617970850357 ) ) ;
#19486=CARTESIAN_POINT ( 'NONE',  ( -30.68756512533535386, 0.07659338870116388920, -6.417149656870462238 ) ) ;
#19489=CARTESIAN_POINT ( 'NONE',  ( 27.17392716606788738, -6.462269799051562735, -16.83742809164828813 ) ) ;
#19501=CARTESIAN_POINT ( 'NONE',  ( 0.09913434393121192678, 20.50242196421552165, -30.00000000000001066 ) ) ;
#19506=CARTESIAN_POINT ( 'NONE',  ( 14.31276673011558209, 14.78156386205161610, -28.23264745093075234 ) ) ;
#19507=CARTESIAN_POINT ( 'NONE',  ( 6.253476071100840805, 21.63181789309742697, -23.22608574772441870 ) ) ;
#19510=CARTESIAN_POINT ( 'NONE',  ( 11.35509078104043112, -19.86412214972710899, -21.54793691088456242 ) ) ;
#19516=CARTESIAN_POINT ( 'NONE',  ( -11.13735207663799542, 17.60437961019085762, -26.83156383840440640 ) ) ;
#19519=CARTESIAN_POINT ( 'NONE',  ( 14.20559445519923081, -25.38033748439481840, -10.66220569548931252 ) ) ;
#19524=CARTESIAN_POINT ( 'NONE',  ( -12.65601555930210509, 32.35306062433939900, -5.000000000000000888 ) ) ;
#19527=CARTESIAN_POINT ( 'NONE',  ( -22.71460563496382079, -4.894690698724015299, -22.13699196390837187 ) ) ;
#19530=CARTESIAN_POINT ( 'NONE',  ( 20.47484565207173546, 1.015995796922180006, -30.00000000000000355 ) ) ;
#19531=CARTESIAN_POINT ( 'NONE',  ( 35.48538791413476190, -11.24999995268670006, -5.000000000000002665 ) ) ;
#19535=CARTESIAN_POINT ( 'NONE',  ( -20.97084573062722868, 0.7958700342359013025, -26.22383286897646926 ) ) ;
#19536=DIRECTION ( 'NONE',  ( -0.000000000000000000, -0.000000000000000000, 1.000000000000000000 ) ) ;
#19539=CARTESIAN_POINT ( 'NONE',  ( 23.89622136170986266, -1.342169087894246715, -20.29735455761264262 ) ) ;
#19554=CARTESIAN_POINT ( 'NONE',  ( -20.88678011286848601, 9.201183980115258620, -16.96328878660644790 ) ) ;
#19556=CARTESIAN_POINT ( 'NONE',  ( 13.60358058528764325, -16.01930624727132368, -26.49426777756269402 ) ) ;
#19559=CARTESIAN_POINT ( 'NONE',  ( 15.24511751409066385, 26.68580942243475462, -7.353470569735968354 ) ) ;
#19561=CARTESIAN_POINT ( 'NONE',  ( -12.56632571172008817, 18.66082033402736684, -21.73012474470345623 ) ) ;
#19565=CARTESIAN_POINT ( 'NONE',  ( 11.35793817090670643, 18.00059461891385837, -25.02099990739169755 ) ) ;
#19567=CARTESIAN_POINT ( 'NONE',  ( 31.99386290378327402, -17.63808712151127622, -9.726114945743994156 ) ) ;
#19570=CARTESIAN_POINT ( 'NONE',  ( -14.33922274708733369, 25.50030895700567157, -11.55966223143600047 ) ) ;
#19572=CARTESIAN_POINT ( 'NONE',  ( -13.23125664540841839, -22.57002348086217580, -16.38072535630667304 ) ) ;
#19576=CARTESIAN_POINT ( 'NONE',  ( -20.06706900687590078, -9.031097061974783458, -24.24539032328864607 ) ) ;
#19577=CARTESIAN_POINT ( 'NONE',  ( -14.31977663809412959, -26.17573132815211423, -7.833052140176563150 ) ) ;
#19579=CARTESIAN_POINT ( 'NONE',  ( 12.40596010115784864, 16.36831411943918724, -28.76043401885274164 ) ) ;
#19581=CARTESIAN_POINT ( 'NONE',  ( 24.35497143909449846, 3.753685042505659375, -15.69857805530405770 ) ) ;
#19586=CARTESIAN_POINT ( 'NONE',  ( -22.80720800583724994, 0.3548441269305998569, -21.58251948928919717 ) ) ;
#19588=CARTESIAN_POINT ( 'NONE',  ( 29.81871666203916860, -0.4633601488208085595, -10.61095171305142237 ) ) ;
#19592=CARTESIAN_POINT ( 'NONE',  ( -20.55563217186186620, -29.52600041847739831, -13.99876745781540777 ) ) ;
#19606=CARTESIAN_POINT ( 'NONE',  ( 15.49469401537697877, -13.43643885346290467, -29.23020519650644999 ) ) ;
#19609=CARTESIAN_POINT ( 'NONE',  ( 10.57951390145473880, 17.61515124497404727, -28.68921471184503247 ) ) ;
#19610=DIRECTION ( 'NONE',  ( 0.000000000000000000, 0.000000000000000000, 1.000000000000000000 ) ) ;
#19612=CARTESIAN_POINT ( 'NONE',  ( -15.94292200871946363, 16.92080024915129144, -17.84332993048722571 ) ) ;
#19614=CARTESIAN_POINT ( 'NONE',  ( 10.52269179291350376, -19.57971688490037110, -22.73667610652659477 ) ) ;
#19616=CARTESIAN_POINT ( 'NONE',  ( 15.02065328176380810, 25.96055969456606505, -9.238703151935258262 ) ) ;
#19618=CARTESIAN_POINT ( 'NONE',  ( 15.41558956916364664, 26.78481017491955285, -5.000000000000000000 ) ) ;
#19620=CARTESIAN_POINT ( 'NONE',  ( -11.02719225547328818, 17.53326252175294897, -27.44422965767462586 ) ) ;
#19622=CARTESIAN_POINT ( 'NONE',  ( -15.23983141892431981, -26.39157610348082983, -7.828191424447879854 ) ) ;
#19625=CARTESIAN_POINT ( 'NONE',  ( -31.59563369834444302, -19.08695624603514673, -9.281276475905125167 ) ) ;
#19626=CARTESIAN_POINT ( 'NONE',  ( -3.293094573708170714, -20.34456577815404188, -28.28364186545810455 ) ) ;
#19627=CARTESIAN_POINT ( 'NONE',  ( 11.39019116559808076, 17.18986029501263602, -28.09783186015068779 ) ) ;
#19629=CARTESIAN_POINT ( 'NONE',  ( 20.92795771179241626, 8.548002118599240973, -17.98415772267350832 ) ) ;
#19630=CARTESIAN_POINT ( 'NONE',  ( 31.12126637737784307, -22.29934860316716438, -5.000000000000000000 ) ) ;
#19634=CARTESIAN_POINT ( 'NONE',  ( -26.72032155736675207, -3.378370715629333887, -17.03970011708248222 ) ) ;
#19640=CARTESIAN_POINT ( 'NONE',  ( 34.13230107285825454, -16.19066397787869249, -7.548977151778921701 ) ) ;
#19650=CARTESIAN_POINT ( 'NONE',  ( -0.5026506373464326716, 25.74991689940979711, -19.62692947300378776 ) ) ;
#19657=CARTESIAN_POINT ( 'NONE',  ( 14.21692097054198634, 29.76874005997475692, -5.917914220045247475 ) ) ;
#19660=CARTESIAN_POINT ( 'NONE',  ( -16.80464701721349385, 11.74058409121013469, -29.42729362730365494 ) ) ;
#19665=CARTESIAN_POINT ( 'NONE',  ( 15.55330811712816796, -26.75926366330655881, -5.473885071091127763 ) ) ;
#19667=CARTESIAN_POINT ( 'NONE',  ( 15.38114701770948223, 26.81500699202883808, -5.945400566827167665 ) ) ;
#19668=CARTESIAN_POINT ( 'NONE',  ( -9.163310636333559245, 20.63632441393290762, -29.99999999999998579 ) ) ;
#19671=CARTESIAN_POINT ( 'NONE',  ( -14.92586248739858057, -14.88347242730710285, -26.39567461636375612 ) ) ;
#19672=CARTESIAN_POINT ( 'NONE',  ( 6.239928823093291221, -25.04180554674758596, -6.442187431363892713 ) ) ;
#19673=CARTESIAN_POINT ( 'NONE',  ( 15.26025490481548452, 25.99765090567122172, -8.299852100227690599 ) ) ;
#19674=CARTESIAN_POINT ( 'NONE',  ( 20.51130358758450001, 13.93060706563202800, -6.938413485835397410 ) ) ;
#19675=DIRECTION ( 'NONE',  ( -0.000000000000000000, -0.000000000000000000, 1.000000000000000000 ) ) ;
#19677=EDGE_LOOP ( 'NONE', ( #7733, #29082, #37528, #10269 ) ) ;
#19678=CARTESIAN_POINT ( 'NONE',  ( -9.303379230217553086, 35.08951236559498454, -7.168276996282715530 ) ) ;
#19683=CARTESIAN_POINT ( 'NONE',  ( 20.81893642488379115, 0.7903601759063493271, -26.82748604854442931 ) ) ;
#19688=CARTESIAN_POINT ( 'NONE',  ( -27.04348299841949910, 0.3741087672331259162, -14.48585235329367826 ) ) ;
#19692=CARTESIAN_POINT ( 'NONE',  ( 27.20974068289347159, -7.315317279060644218, -16.79268240890852937 ) ) ;
#19705=DIRECTION ( 'NONE',  ( 0.000000000000000000, 0.000000000000000000, 1.000000000000000000 ) ) ;
#19707=CARTESIAN_POINT ( 'NONE',  ( -1.541676259743169464, 20.48416492902245167, -30.00000000000001421 ) ) ;
#19710=CARTESIAN_POINT ( 'NONE',  ( 17.19287287506014295, 19.26288574755855620, -10.79497166203956660 ) ) ;
#19711=CARTESIAN_POINT ( 'NONE',  ( 6.954109223000227047, 24.07807191830993077, -19.86921157130286275 ) ) ;
#19719=CARTESIAN_POINT ( 'NONE',  ( 10.01866435034643743, -18.04234178223556029, -28.05214097278188490 ) ) ;
#19723=CARTESIAN_POINT ( 'NONE',  ( -14.53535404462992098, 24.96185776678678891, -11.59977167594924019 ) ) ;
#19726=CARTESIAN_POINT ( 'NONE',  ( 10.46771542449441306, -20.07731438429163617, -21.66176537328637508 ) ) ;
#19728=VERTEX_POINT ( 'NONE', #27951 ) ;
#19730=CARTESIAN_POINT ( 'NONE',  ( -9.705446205519352887, 20.57320699630038519, -22.42486721958433549 ) ) ;
#19733=MECHANICAL_DESIGN_GEOMETRIC_PRESENTATION_REPRESENTATION('',(#8047),#12601);
#19734=CARTESIAN_POINT ( 'NONE',  ( -21.94754318934862169, -4.722844451827508117, -23.27871882223563205 ) ) ;
#19737=CARTESIAN_POINT ( 'NONE',  ( 30.70366785093425932, 0.06005377067882849973, -6.417126122636190644 ) ) ;
#19738=CARTESIAN_POINT ( 'NONE',  ( 15.41558956916364842, 26.78481017491955285, -5.948412119462402003 ) ) ;
#19741=CARTESIAN_POINT ( 'NONE',  ( -30.79516076619654896, -0.03407914214386141560, -6.416988314164135510 ) ) ;
#19745=CARTESIAN_POINT ( 'NONE',  ( 30.29736254084309621, -2.797781772719168725, -12.30903580646858941 ) ) ;
#19747=CARTESIAN_POINT ( 'NONE',  ( 20.21580222128064364, 3.470454069710441569, -30.00000000000000355 ) ) ;
#19751=DIRECTION ( 'NONE',  ( 1.000000000000000000, 0.000000000000000000, -0.000000000000000000 ) ) ;
#19759=CARTESIAN_POINT ( 'NONE',  ( -19.49657363026103951, 7.925481962114715451, -24.37616138078942640 ) ) ;
#19761=CARTESIAN_POINT ( 'NONE',  ( 14.87465728246612606, -18.53959208443260920, -21.11850284650765275 ) ) ;
#19763=CARTESIAN_POINT ( 'NONE',  ( -20.57924982997939622, -27.21273881503329051, -4.999999999999998224 ) ) ;
#19766=CARTESIAN_POINT ( 'NONE',  ( 13.96311103245068175, 24.09699048448357317, -13.49799974867627661 ) ) ;
#19769=CARTESIAN_POINT ( 'NONE',  ( -12.28865036616621786, 17.24410649058709311, -25.13873084831685745 ) ) ;
#19772=CARTESIAN_POINT ( 'NONE',  ( 11.03067133885425655, 17.27930474757444657, -30.00000000000000000 ) ) ;
#19774=CARTESIAN_POINT ( 'NONE',  ( 31.66152258591498736, -17.45444667796995120, -10.17335708870760946 ) ) ;
#19777=CARTESIAN_POINT ( 'NONE',  ( -10.78183262531012154, 17.59235075900286915, -28.06201921541798328 ) ) ;
#19779=CARTESIAN_POINT ( 'NONE',  ( -16.75447718561904864, -27.02424154557581915, -5.000000000000000000 ) ) ;
#19782=CARTESIAN_POINT ( 'NONE',  ( -28.46622419312624430, -12.75272502055737434, -14.74906803505498765 ) ) ;
#19783=CARTESIAN_POINT ( 'NONE',  ( -11.69238095878992745, -22.55098709441451632, -16.51565108365196721 ) ) ;
#19785=CARTESIAN_POINT ( 'NONE',  ( 13.21519265033025370, 15.68751749194264811, -30.00000000000001066 ) ) ;
#19787=CARTESIAN_POINT ( 'NONE',  ( 27.78359518671923212, 2.894372651951440112, -8.330351127553241142 ) ) ;
#19791=CARTESIAN_POINT ( 'NONE',  ( -26.62727581776185559, 0.09304277698053113610, -15.42802191721595406 ) ) ;
#19794=CARTESIAN_POINT ( 'NONE',  ( 31.41207073737789557, -0.7790156937066328169, -6.867375471341749638 ) ) ;
#19800=CARTESIAN_POINT ( 'NONE',  ( -21.88444403592365362, 6.126538576424530369, -30.00000000000001066 ) ) ;
#19813=CARTESIAN_POINT ( 'NONE',  ( 27.32249163041963413, -25.19218879630926367, -5.869363991529141344 ) ) ;
#19820=CARTESIAN_POINT ( 'NONE',  ( 10.51082547654175059, 17.86856945860100865, -27.40418496694546135 ) ) ;
#19822=VERTEX_POINT ( 'NONE', #29556 ) ;
#19823=CARTESIAN_POINT ( 'NONE',  ( -16.96185042632790640, 20.08371563433640716, -10.29097588471536362 ) ) ;
#19825=CARTESIAN_POINT ( 'NONE',  ( 9.484687302133613329, -18.22422652986723079, -28.70838076812352213 ) ) ;
#19826=CARTESIAN_POINT ( 'NONE',  ( 30.90412082983250741, -0.04211290444289944590, -5.000000000000000000 ) ) ;
#19827=CARTESIAN_POINT ( 'NONE',  ( 11.01823919507857141, 17.34030634537447213, -28.70746280985912691 ) ) ;
#19829=CARTESIAN_POINT ( 'NONE',  ( 15.39658735393897437, 26.76009586085592673, -5.946078209756686661 ) ) ;
#19831=CARTESIAN_POINT ( 'NONE',  ( -15.06796771947636771, 26.24911050298840820, -8.762714437537596268 ) ) ;
#19833=CARTESIAN_POINT ( 'NONE',  ( -10.22236381303094532, -19.16528309895199556, -23.85432085113489364 ) ) ;
#19835=VECTOR ( 'NONE', #13911, 1000.000000000000000 ) ;
#19837=CARTESIAN_POINT ( 'NONE',  ( -32.98459937871956527, -19.91850110786283423, -5.435368959122942378 ) ) ;
#19838=CARTESIAN_POINT ( 'NONE',  ( -4.803568943853530726, -24.90644357294165090, -5.962994550823584206 ) ) ;
#19839=CARTESIAN_POINT ( 'NONE',  ( 12.41354392755694391, 18.82514156286238105, -21.70496632052628527 ) ) ;
#19841=CARTESIAN_POINT ( 'NONE',  ( 19.02940903860087829, 8.038401761433641823, -27.15973525649786779 ) ) ;
#19846=CARTESIAN_POINT ( 'NONE',  ( -31.09817132049496280, -1.548763601471955464, -9.610625396712832114 ) ) ;
#19854=CARTESIAN_POINT ( 'NONE',  ( 33.95719716996227078, -16.10408066851575626, -7.976629801705419354 ) ) ;
#19864=CARTESIAN_POINT ( 'NONE',  ( -1.787501278500105206, 35.33670910843994761, -11.06934470569155415 ) ) ;
#19871=CARTESIAN_POINT ( 'NONE',  ( 13.06030798789831948, 27.04582189987735319, -12.35125024899165780 ) ) ;
#19872=CARTESIAN_POINT ( 'NONE',  ( 33.51290647813760870, -3.280245463519940063, -4.999999999999999112 ) ) ;
#19874=CARTESIAN_POINT ( 'NONE',  ( -19.55823056015679384, 15.51636888105696066, -7.909696038444731236 ) ) ;
#19877=CARTESIAN_POINT ( 'NONE',  ( 9.532625661562562414, -18.14880370279404076, -30.00000000000000000 ) ) ;
#19879=CARTESIAN_POINT ( 'NONE',  ( 13.47022650129216537, 22.85893131970043868, -15.44577212985798198 ) ) ;
#19880=CARTESIAN_POINT ( 'NONE',  ( -33.62187204924172335, 0.04418559750806146796, -5.000000000000000000 ) ) ;
#19882=CARTESIAN_POINT ( 'NONE',  ( -28.06200121101475986, -24.80525908879649322, -5.000000000000006217 ) ) ;
#19883=CARTESIAN_POINT ( 'NONE',  ( 6.004260983034707344, -24.46000915886378735, -10.33918878589541102 ) ) ;
#19884=CARTESIAN_POINT ( 'NONE',  ( 12.22994242602892712, 19.80693455908184930, -20.55844498058446135 ) ) ;
#19885=CARTESIAN_POINT ( 'NONE',  ( 18.83106894595607983, 13.86228728257169962, -14.90432550276213242 ) ) ;
#19889=CARTESIAN_POINT ( 'NONE',  ( -9.351165396203874991, 35.32073807392316667, -6.306370732072846153 ) ) ;
#19891=CARTESIAN_POINT ( 'NONE',  ( -15.33953269408914544, -26.67883706601617888, -5.946098135196418610 ) ) ;
#19892=AXIS2_PLACEMENT_3D ( 'NONE', #5788, #2742, #15134 ) ;
#19895=CARTESIAN_POINT ( 'NONE',  ( 30.03307712974922339, -0.01506494207477212556, -9.235894060447490617 ) ) ;
#19897=DIRECTION ( 'NONE',  ( 0.000000000000000000, 0.000000000000000000, 1.000000000000000000 ) ) ;
#19899=CARTESIAN_POINT ( 'NONE',  ( -21.69376705123304561, 0.8088866752443155672, -23.86354191580900874 ) ) ;
#19901=CARTESIAN_POINT ( 'NONE',  ( 31.75158787230413537, -7.547111399419645039, -12.10492256910596431 ) ) ;
#19914=CARTESIAN_POINT ( 'NONE',  ( 17.94915298279187965, 17.13629230656877667, -11.82338326548747887 ) ) ;
#19916=CARTESIAN_POINT ( 'NONE',  ( 9.390451618560783587, 29.18342345638610880, -13.98827517472965098 ) ) ;
#19922=CARTESIAN_POINT ( 'NONE',  ( 16.10068483903742376, -26.35529856002330718, -8.725391069711090353 ) ) ;
#19927=CARTESIAN_POINT ( 'NONE',  ( -15.41919230091076187, 26.77186013819068577, -5.474270845225373883 ) ) ;
#19929=CARTESIAN_POINT ( 'NONE',  ( 14.73589040286153562, -26.36289149956793310, -7.360008916301447712 ) ) ;
#19935=CARTESIAN_POINT ( 'NONE',  ( -9.018867048779389606, 18.89568106175847362, -26.64054324667225160 ) ) ;
#19936=CARTESIAN_POINT ( 'NONE',  ( -12.22510875462229762, -16.67830573107660541, -27.92440096918162595 ) ) ;
#19938=CARTESIAN_POINT ( 'NONE',  ( -35.08557715296313262, -7.694570891656546507, -5.446627638814927508 ) ) ;
#19941=CARTESIAN_POINT ( 'NONE',  ( 26.42155565230272529, 0.4047387329622965657, -15.46047363215482129 ) ) ;
#19945=CARTESIAN_POINT ( 'NONE',  ( -21.27851422119422153, 0.7607673571408221092, -25.01294376240213779 ) ) ;
#19947=ORIENTED_EDGE ( 'NONE', *, *, #26148, .F. ) ;
#19948=CARTESIAN_POINT ( 'NONE',  ( 33.15613636589012003, -3.183923766461477012, -6.816378949858656888 ) ) ;
#19965=CARTESIAN_POINT ( 'NONE',  ( -22.18267962388761205, 8.601427261759537757, -13.87176402086122096 ) ) ;
#19966=CARTESIAN_POINT ( 'NONE',  ( 20.32386968494314772, -26.55043266981761718, -8.585248161735293593 ) ) ;
#19971=CARTESIAN_POINT ( 'NONE',  ( 11.01761205127317211, 17.68717171916146214, -26.82030036599024569 ) ) ;
#19974=CARTESIAN_POINT ( 'NONE',  ( -11.90029320544120139, 17.22241791299109792, -26.29854751065716201 ) ) ;
#19978=CARTESIAN_POINT ( 'NONE',  ( 11.03067133885425655, 17.27930474757444657, -29.34935180445048886 ) ) ;
#19980=CARTESIAN_POINT ( 'NONE',  ( 33.48737131668896438, -18.46746012246179802, -6.696811483700092715 ) ) ;
#19984=CARTESIAN_POINT ( 'NONE',  ( -15.15253849576580514, 26.98910714531248090, -7.345250183262973742 ) ) ;
#19986=CARTESIAN_POINT ( 'NONE',  ( -9.644844900892618256, -18.14121070125914414, -28.70205165269834424 ) ) ;
#19990=CARTESIAN_POINT ( 'NONE',  ( -19.54202594190227416, -8.796642138048818893, -25.59909437478174610 ) ) ;
#19991=CARTESIAN_POINT ( 'NONE',  ( -14.81594859391628027, -26.54803943294492896, -5.946254171449712800 ) ) ;
#19993=CARTESIAN_POINT ( 'NONE',  ( 16.48001596753842435, 21.51165321008922859, -9.781392695578974283 ) ) ;
#19995=CARTESIAN_POINT ( 'NONE',  ( 26.24812223541028544, 2.914455890864420251, -12.67480056851672821 ) ) ;
#19999=CARTESIAN_POINT ( 'NONE',  ( -20.70520357564727476, 0.6698834183737596426, -27.43687480068400575 ) ) ;
#20000=CARTESIAN_POINT ( 'NONE',  ( 22.82302083792669478, 0.2992910856866396463, -21.57503696421676409 ) ) ;
#20004=CARTESIAN_POINT ( 'NONE',  ( -21.42264437035803581, 2.133308088443877981, -24.00964802334802073 ) ) ;
#20006=CARTESIAN_POINT ( 'NONE',  ( -3.091399026088746727, 22.35909668862748134, -29.99999999999999289 ) ) ;
#20018=CARTESIAN_POINT ( 'NONE',  ( 15.66978274593486198, -13.58963625838278055, -27.75455164708249356 ) ) ;
#20021=EDGE_CURVE ( 'NONE', #648, #7392, #36969, .T. ) ;
#20022=CARTESIAN_POINT ( 'NONE',  ( 11.30519648601890914, 19.26922631836183442, -22.66966561975009142 ) ) ;
#20025=CARTESIAN_POINT ( 'NONE',  ( -17.37423461678738690, 20.74184956833279969, -6.432056361720852600 ) ) ;
#20028=CARTESIAN_POINT ( 'NONE',  ( 15.06737607521339939, -26.25728709294644503, -8.298505300031854048 ) ) ;
#20030=CARTESIAN_POINT ( 'NONE',  ( 11.48833225930353130, 18.43385336031954225, -23.85456489029450111 ) ) ;
#20032=CARTESIAN_POINT ( 'NONE',  ( 10.97760868008098889, 17.31306259807076131, -29.34820719497326280 ) ) ;
#20034=CARTESIAN_POINT ( 'NONE',  ( -12.88510495915603293, 21.72514915063214502, -17.42774926625122589 ) ) ;
#20036=CARTESIAN_POINT ( 'NONE',  ( -9.778777969284597305, -18.56702052074433951, -26.22551016879890184 ) ) ;
#20040=CARTESIAN_POINT ( 'NONE',  ( -28.66680771549815887, -17.31871082804386219, -12.88878534390529040 ) ) ;
#20041=CARTESIAN_POINT ( 'NONE',  ( -4.708882860453130981, -19.97645208405714712, -28.83077065012970408 ) ) ;
#20042=CARTESIAN_POINT ( 'NONE',  ( 15.84467149865224833, 25.30824157118464868, -5.474055608616841262 ) ) ;
#20044=CARTESIAN_POINT ( 'NONE',  ( 23.21632290521470665, 9.180027527831590817, -7.909577862357840772 ) ) ;
#20045=CARTESIAN_POINT ( 'NONE',  ( 35.48538791413476190, -11.24999995268670006, -5.000000000000002665 ) ) ;
#20048=AXIS2_PLACEMENT_3D ( 'NONE', #34198, #270, #24847 ) ;
#20050=CARTESIAN_POINT ( 'NONE',  ( -29.97494448726338234, -2.192815450784864062, -12.34847330071091598 ) ) ;
#20057=CARTESIAN_POINT ( 'NONE',  ( 33.32532820267570628, -17.07072135929075429, -8.406244610255813043 ) ) ;
#20067=CARTESIAN_POINT ( 'NONE',  ( -1.577295330230392700, 31.28878489215165715, -14.73372383095288285 ) ) ;
#20074=CARTESIAN_POINT ( 'NONE',  ( 13.99360449555652686, 28.17614020743589265, -9.588039117105212839 ) ) ;
#20077=CARTESIAN_POINT ( 'NONE',  ( -20.11194080487678804, 14.58715024383956482, -7.424181446863920897 ) ) ;
#20081=CARTESIAN_POINT ( 'NONE',  ( 9.599968447380561543, -18.25860783104283769, -28.07576543594807461 ) ) ;
#20083=CARTESIAN_POINT ( 'NONE',  ( 11.08697006596329793, 17.63936566195119227, -26.82682961117613729 ) ) ;
#20084=CARTESIAN_POINT ( 'NONE',  ( -30.41237130417910706, 3.314011747244090422, -13.58461195433496371 ) ) ;
#20087=CARTESIAN_POINT ( 'NONE',  ( -22.94869330768877802, -20.35003466596009858, -14.81020240946884492 ) ) ;
#20088=CARTESIAN_POINT ( 'NONE',  ( 7.129976846286900205, -22.60938466117447732, -16.81300626758635630 ) ) ;
#20089=CARTESIAN_POINT ( 'NONE',  ( 15.54167675008477723, 26.33752833710220997, -5.000000000000000888 ) ) ;
#20090=CARTESIAN_POINT ( 'NONE',  ( 18.44994286627233038, 12.34598615494684637, -19.05470978867802145 ) ) ;
#20093=CARTESIAN_POINT ( 'NONE',  ( -4.084317376857201864, 20.18095795116958158, -28.48257084316769294 ) ) ;
#20102=CARTESIAN_POINT ( 'NONE',  ( -30.63398949461165088, 0.1319342208294977115, -6.417236068070889310 ) ) ;
#20105=CARTESIAN_POINT ( 'NONE',  ( 23.45217438398567111, -5.581096782014018487, -20.95586870486150843 ) ) ;
#20110=ORIENTED_EDGE ( 'NONE', *, *, #31497, .T. ) ;
#20116=SURFACE_STYLE_FILL_AREA ( #29048 ) ;
#20120=CARTESIAN_POINT ( 'NONE',  ( 15.98323640732827400, 14.59684562732355673, -22.14531699329461034 ) ) ;
#20121=CARTESIAN_POINT ( 'NONE',  ( 6.309536247299391221, 19.51471286317475773, -29.25949660933323671 ) ) ;
#20127=CARTESIAN_POINT ( 'NONE',  ( 11.72988935907280350, -20.95426047538857972, -19.47340356160194474 ) ) ;
#20132=CARTESIAN_POINT ( 'NONE',  ( -10.99444046889570537, 17.35561201924551256, -28.70647127135751475 ) ) ;
#20134=CARTESIAN_POINT ( 'NONE',  ( 12.30749475060790843, -22.55415536556771272, -16.47007971746634780 ) ) ;
#20138=CARTESIAN_POINT ( 'NONE',  ( -9.699844911044960938, 24.40834062817878447, -17.99019714132644765 ) ) ;
#20142=CARTESIAN_POINT ( 'NONE',  ( -25.28614151405769306, -6.243831222781579982, -18.83763890451589518 ) ) ;
#20145=CARTESIAN_POINT ( 'NONE',  ( 29.46685023586550400, 0.1954524857158681794, -10.18384896449856036 ) ) ;
#20150=CARTESIAN_POINT ( 'NONE',  ( -28.89319593916525264, 0.09792079263888439633, -11.59890374343908803 ) ) ;
#20153=CARTESIAN_POINT ( 'NONE',  ( 29.11583290636277255, -1.894276822915576863, -13.31891975639820025 ) ) ;
#20166=CARTESIAN_POINT ( 'NONE',  ( 3.215895501801615985, 24.37283748036874442, -20.74290920587755593 ) ) ;
#20170=CARTESIAN_POINT ( 'NONE',  ( 16.66225199357186426, -19.51117972168512082, -18.94818515844563933 ) ) ;
#20171=DIRECTION ( 'NONE',  ( 0.000000000000000000, 0.000000000000000000, -1.000000000000000000 ) ) ;
#20175=CARTESIAN_POINT ( 'NONE',  ( 14.24751785689744743, 24.58680083500108182, -12.54074944469350683 ) ) ;
#20177=CARTESIAN_POINT ( 'NONE',  ( -14.73975063325908152, 24.40991067048773644, -11.61570129997859269 ) ) ;
#20181=CARTESIAN_POINT ( 'NONE',  ( 14.96335647831743287, 25.71149453912319771, -9.710330481890405707 ) ) ;
#20183=CARTESIAN_POINT ( 'NONE',  ( 19.07715750984440817, -9.791667150159778288, -25.58058246820311865 ) ) ;
#20186=CARTESIAN_POINT ( 'NONE',  ( -11.67086652466456087, 19.61581206493572438, -21.57501891504949398 ) ) ;
#20188=CARTESIAN_POINT ( 'NONE',  ( -13.21758073316063431, -21.34862723106953197, -18.29696183777072704 ) ) ;
#20191=CARTESIAN_POINT ( 'NONE',  ( -19.06849745787630468, -8.585213063630757091, -26.98300186761300878 ) ) ;
#20192=CARTESIAN_POINT ( 'NONE',  ( -11.91314923935176928, -22.03502826895537936, -17.47013640216600905 ) ) ;
#20194=CARTESIAN_POINT ( 'NONE',  ( 17.13680108443139716, 20.87122319733086329, -7.868605303123856309 ) ) ;
#20196=CARTESIAN_POINT ( 'NONE',  ( 26.51973020456226493, 3.772046466887580607, -10.27100251072616288 ) ) ;
#20200=CARTESIAN_POINT ( 'NONE',  ( -29.52555509693227265, -0.1188359627376792682, -10.63800653123224293 ) ) ;
#20201=CARTESIAN_POINT ( 'NONE',  ( 24.79371228178270314, -0.05885538004481753738, -18.38622137752647134 ) ) ;
#20207=CARTESIAN_POINT ( 'NONE',  ( -20.44235121065545613, 1.535337040937289066, -29.36017822837253988 ) ) ;
#20208=CARTESIAN_POINT ( 'NONE',  ( -11.10756861982300947, 19.59949212537556562, -20.90349153980999830 ) ) ;
#20217=CARTESIAN_POINT ( 'NONE',  ( -21.97373458415457037, 5.076385617489679980, -19.92418931931740644 ) ) ;
#20220=CARTESIAN_POINT ( 'NONE',  ( 28.35230428231212230, -24.61827297795788638, -5.439370354368517013 ) ) ;
#20223=CARTESIAN_POINT ( 'NONE',  ( 15.24739647947424714, 27.26377957105179917, -5.940767840820030621 ) ) ;
#20227=CARTESIAN_POINT ( 'NONE',  ( -16.88103042039869450, 19.95524105454239816, -10.77970369993180277 ) ) ;
#20231=CARTESIAN_POINT ( 'NONE',  ( 9.910011124334165089, -18.83656552785947724, -25.02100245519685018 ) ) ;
#20234=CARTESIAN_POINT ( 'NONE',  ( 11.08571900862292026, 17.49394017797068557, -27.44878439575566631 ) ) ;
#20236=CARTESIAN_POINT ( 'NONE',  ( 11.29809999771842932, 18.04734829986520950, -25.01294377573191952 ) ) ;
#20238=CARTESIAN_POINT ( 'NONE',  ( -11.83932568694060450, 19.43865753690332809, -21.60690038723429751 ) ) ;
#20239=CARTESIAN_POINT ( 'NONE',  ( -20.23296131041716706, 28.12381335138030636, 3.000000000000000000 ) ) ;
#20240=CARTESIAN_POINT ( 'NONE',  ( -10.20105000702817932, -19.17274393931131371, -23.85688496074367393 ) ) ;
#20242=CARTESIAN_POINT ( 'NONE',  ( -17.41815810822877353, -11.99257218473442776, -26.26776909220020784 ) ) ;
#20243=CARTESIAN_POINT ( 'NONE',  ( -7.781299079984965061, -22.59512116915117375, -16.77857488574911571 ) ) ;
#20244=CARTESIAN_POINT ( 'NONE',  ( 15.76470487440841062, 24.68801468592181791, -7.838331335750884143 ) ) ;
#20246=CARTESIAN_POINT ( 'NONE',  ( 21.20949775426257844, 8.625473678353458240, -16.95001661513558844 ) ) ;
#20247=CARTESIAN_POINT ( 'NONE',  ( 20.23296131041715640, 28.12381335138032412, 0.000000000000000000 ) ) ;
#20249=CARTESIAN_POINT ( 'NONE',  ( -12.12384649078149934, -25.96922316649875739, -5.000000000000000888 ) ) ;
#20252=CARTESIAN_POINT ( 'NONE',  ( -21.46822025407879408, -1.246220581431492391, -24.79526857062417733 ) ) ;
#20258=CARTESIAN_POINT ( 'NONE',  ( 34.01930034203780906, -17.43549634978032969, -6.697537572123588134 ) ) ;
#20265=CARTESIAN_POINT ( 'NONE',  ( 0.9672072501420434509, 23.74532692743124329, -21.84035651827026214 ) ) ;
#20272=CARTESIAN_POINT ( 'NONE',  ( 14.23294558246579022, 29.80882899807581055, -5.461287637657078697 ) ) ;
#20276=CARTESIAN_POINT ( 'NONE',  ( -20.19236039815038808, 14.65651441764425833, -5.965904664850079087 ) ) ;
#20279=CARTESIAN_POINT ( 'NONE',  ( 15.01100859456593817, -25.99757226175481861, -9.236802265591313343 ) ) ;
#20281=CARTESIAN_POINT ( 'NONE',  ( 14.26815522538843872, 24.53214742665168302, -12.54540486666444643 ) ) ;
#20282=CARTESIAN_POINT ( 'NONE',  ( -19.79815887584811307, 19.84782313723621883, -13.42901749168595771 ) ) ;
#20285=CARTESIAN_POINT ( 'NONE',  ( -26.47200088153462261, -24.85570260301889789, -8.022744550273097630 ) ) ;
#20287=CARTESIAN_POINT ( 'NONE',  ( 4.020749035821322259, -24.85085155051347883, -5.964422724544506060 ) ) ;
#20288=CARTESIAN_POINT ( 'NONE',  ( 15.04807939094960290, 25.45191101363087682, -9.714351570550116222 ) ) ;
#20289=CARTESIAN_POINT ( 'NONE',  ( 17.67233557286219892, 11.74463701656010706, -23.32306369647684363 ) ) ;
#20292=CARTESIAN_POINT ( 'NONE',  ( -4.679325431169941929, 23.08454507055297711, -21.96044281907038354 ) ) ;
#20301=CARTESIAN_POINT ( 'NONE',  ( -20.47417334391911936, 1.028570030172704985, -30.00000000000000000 ) ) ;
#20304=CARTESIAN_POINT ( 'NONE',  ( 19.84734553509363053, -6.000422723447369044, -27.77669457348836701 ) ) ;
#20320=CARTESIAN_POINT ( 'NONE',  ( 17.86751023708650976, 15.56654134878274753, -14.86208373478310563 ) ) ;
#20322=CARTESIAN_POINT ( 'NONE',  ( 11.67450463981393405, 33.32297107450499141, -6.328599700080098422 ) ) ;
#20324=CARTESIAN_POINT ( 'NONE',  ( 0.000000000000000000, 22.50000000000000355, 10.00000000000000000 ) ) ;
#20327=CARTESIAN_POINT ( 'NONE',  ( 15.72657732487407323, -26.77584194611982937, -5.943392230339449078 ) ) ;
#20334=CARTESIAN_POINT ( 'NONE',  ( -15.33156057601598654, 26.64116238436768214, -6.887479782135956796 ) ) ;
#20337=CARTESIAN_POINT ( 'NONE',  ( 13.92713108795117449, -25.88915498332963594, -8.779116367686647493 ) ) ;
#20341=CARTESIAN_POINT ( 'NONE',  ( -7.677290147211063065, 19.01944725762398392, -29.28149183438886993 ) ) ;
#20345=CARTESIAN_POINT ( 'NONE',  ( -32.50609658070614216, -5.122312372317453288, -10.36378763344411169 ) ) ;
#20348=CARTESIAN_POINT ( 'NONE',  ( 22.20197406284108510, 0.7415789608456136994, -22.74446640454221225 ) ) ;
#20353=CARTESIAN_POINT ( 'NONE',  ( -24.55940606212222121, 0.4314668635417708287, -18.45227070181689299 ) ) ;
#20357=CARTESIAN_POINT ( 'NONE',  ( 27.51989245245352578, -3.247923778376513582, -16.07734993535055779 ) ) ;
#20372=CARTESIAN_POINT ( 'NONE',  ( 2.122071298695014541, 21.02571388690864751, -26.27783819818665734 ) ) ;
#20376=CARTESIAN_POINT ( 'NONE',  ( 19.37949815655151298, -26.73439600029011487, -8.164662001533008251 ) ) ;
#20381=CARTESIAN_POINT ( 'NONE',  ( 10.95089924463749220, 17.48332310871153794, -28.07209419957614216 ) ) ;
#20383=CARTESIAN_POINT ( 'NONE',  ( -13.83645454411932718, 22.14850785795266574, -15.49917614834808077 ) ) ;
#20386=CARTESIAN_POINT ( 'NONE',  ( 12.69086781283033893, 20.99879331917208347, -18.45872641518607793 ) ) ;
#20388=CARTESIAN_POINT ( 'NONE',  ( 31.77418123208467549, -18.80321225436984633, -9.280942705184974884 ) ) ;
#20391=CARTESIAN_POINT ( 'NONE',  ( -14.61013790624355302, 27.97863390761640900, -8.234326149446673071 ) ) ;
#20393=CARTESIAN_POINT ( 'NONE',  ( -10.34184770646355922, -17.97369560806122735, -27.39515243922713594 ) ) ;
#20397=CARTESIAN_POINT ( 'NONE',  ( -25.39605442066326901, -11.39641072833809865, -17.62077034726572577 ) ) ;
#20398=CARTESIAN_POINT ( 'NONE',  ( -14.96511953850379939, -26.58463093893972484, -5.946192477338447802 ) ) ;
#20400=CARTESIAN_POINT ( 'NONE',  ( 15.73537490736885402, 20.22929917737018712, -13.69120337137130861 ) ) ;
#20402=CARTESIAN_POINT ( 'NONE',  ( 28.74059262234505852, 2.003791175848793849, -7.369499878552438155 ) ) ;
#20406=CARTESIAN_POINT ( 'NONE',  ( -30.44000904125844187, -0.09666380877237282232, -8.292869882052704256 ) ) ;
#20407=CARTESIAN_POINT ( 'NONE',  ( 31.30187684039734819, -0.7690320538238586412, -7.331994754779891821 ) ) ;
#20411=CARTESIAN_POINT ( 'NONE',  ( -29.05832138661633124, 1.740516625605465828, -6.894049278760337351 ) ) ;
#20412=CARTESIAN_POINT ( 'NONE',  ( -1.775381057445013511E-14, 40.84107189184581443, -14.51648065752882566 ) ) ;
#20416=AXIS2_PLACEMENT_3D ( 'NONE', #39836, #33952, #6109 ) ;
#20421=CARTESIAN_POINT ( 'NONE',  ( -20.05673146015622521, 4.300176513202893958, -29.39846272892710388 ) ) ;
#20424=CARTESIAN_POINT ( 'NONE',  ( 15.35557683603447465, -14.15435181208574988, -27.05163929191509098 ) ) ;
#20427=CARTESIAN_POINT ( 'NONE',  ( 15.25529914957406952, 27.06982126769854347, -6.410865638208865569 ) ) ;
#20430=CARTESIAN_POINT ( 'NONE',  ( -16.60320053658520578, 21.21075288159243399, -9.787007994218763329 ) ) ;
#20433=CARTESIAN_POINT ( 'NONE',  ( 10.16741497705453767, -19.18446152325294918, -23.86097873014023563 ) ) ;
#20435=CARTESIAN_POINT ( 'NONE',  ( 15.24022193870092323, 26.37920915382371945, -7.827918218439406495 ) ) ;
#20439=CARTESIAN_POINT ( 'NONE',  ( -12.84659171310743808, 21.78875632697887355, -17.41907714049541411 ) ) ;
#20441=CARTESIAN_POINT ( 'NONE',  ( -15.10428467780321604, -26.15168814349211956, -8.766821641356482786 ) ) ;
#20444=CARTESIAN_POINT ( 'NONE',  ( -23.93117376754405612, -14.45163223871617042, -17.59434270118057242 ) ) ;
#20445=CARTESIAN_POINT ( 'NONE',  ( -4.698712440877560681, -19.95451542538867784, -29.41287879531005345 ) ) ;
#20446=CARTESIAN_POINT ( 'NONE',  ( 15.40307908694031802, 23.98740442282029761, -10.21161987371616142 ) ) ;
#20449=CARTESIAN_POINT ( 'NONE',  ( 19.71920213142633571, 7.415869230238018694, -24.35972737311789516 ) ) ;
#20451=CARTESIAN_POINT ( 'NONE',  ( -15.33886719106936170, -26.70425067113273698, -5.000000000000000000 ) ) ;
#20456=CARTESIAN_POINT ( 'NONE',  ( -20.49395421059513467, -1.780101454358719915, -28.61385821411536767 ) ) ;
#20462=CARTESIAN_POINT ( 'NONE',  ( 28.24618586764199080, -13.39106098617326168, -14.74144434279989468 ) ) ;
#20463=DIRECTION ( 'NONE',  ( -0.000000000000000000, -0.000000000000000000, -1.000000000000000000 ) ) ;
#20471=CARTESIAN_POINT ( 'NONE',  ( 0.9279571259586922860, 22.81800067625227157, -22.98705170056795311 ) ) ;
#20472=DIRECTION ( 'NONE',  ( 0.000000000000000000, 0.000000000000000000, 1.000000000000000000 ) ) ;
#20476=CYLINDRICAL_SURFACE ( 'NONE', #17098, 62.00000000000014211 ) ;
#20478=CARTESIAN_POINT ( 'NONE',  ( 9.842964772816607422, 17.98588232539188425, -30.00000000000000000 ) ) ;
#20482=CARTESIAN_POINT ( 'NONE',  ( -19.11280093006975989, 16.54705272908905656, -7.416057572179566293 ) ) ;
#20486=CARTESIAN_POINT ( 'NONE',  ( 9.523339034571952411, -18.15368110581538019, -29.34782467990711652 ) ) ;
#20488=CARTESIAN_POINT ( 'NONE',  ( 14.52155348942260815, 25.00168942016326667, -11.59674793591240949 ) ) ;
#20490=ADVANCED_FACE ( 'NONE', ( #36164 ), #10981, .T. ) ;
#20492=CARTESIAN_POINT ( 'NONE',  ( -17.73299320380208144, -16.64144535103558553, -20.85865150295031967 ) ) ;
#20493=CARTESIAN_POINT ( 'NONE',  ( 2.749517794474013233, -20.36689819698734993, -30.00000000000001421 ) ) ;
#20494=CARTESIAN_POINT ( 'NONE',  ( 15.54167675008477723, 26.33752833710220997, -5.474103952296149878 ) ) ;
#20495=CARTESIAN_POINT ( 'NONE',  ( 16.72854773719623012, 11.96534557194348913, -28.29306212330370585 ) ) ;
#20498=CARTESIAN_POINT ( 'NONE',  ( -5.263199493313895694, 30.38423091068325732, -14.78917777124115318 ) ) ;
#20506=CARTESIAN_POINT ( 'NONE',  ( -26.37949901244907380, 0.4700838887049326176, -15.46553941099261742 ) ) ;
#20508=CARTESIAN_POINT ( 'NONE',  ( 25.18967108100165220, -7.598938349516441981, -18.76223645604332191 ) ) ;
#20523=CARTESIAN_POINT ( 'NONE',  ( 18.59382115548298131, 17.96292538557851515, -5.479430875336894324 ) ) ;
#20524=CARTESIAN_POINT ( 'NONE',  ( 10.90930865498974178, 30.88252674679933918, -11.23868371367947283 ) ) ;
#20528=CARTESIAN_POINT ( 'NONE',  ( 14.86587968135671112, -25.51001094038641526, -10.63804553132061237 ) ) ;
#20531=CARTESIAN_POINT ( 'NONE',  ( 22.52744239175980567, -0.1803094636422790109, -30.00000000000000000 ) ) ;
#20533=CARTESIAN_POINT ( 'NONE',  ( -13.48645580646731545, 22.82557474682550946, -15.44962328438105281 ) ) ;
#20536=CARTESIAN_POINT ( 'NONE',  ( 11.27276115634963105, -22.55032744237014697, -16.54627474825828770 ) ) ;
#20538=AXIS2_PLACEMENT_3D ( 'NONE', #1096, #35423, #23234 ) ;
#20542=CARTESIAN_POINT ( 'NONE',  ( -10.56723897001253931, 29.14243252867948186, -13.10880484156706238 ) ) ;
#20546=CARTESIAN_POINT ( 'NONE',  ( -20.99207129727855303, -3.171358742653616059, -25.88939096934664263 ) ) ;
#20549=CARTESIAN_POINT ( 'NONE',  ( 25.82638031820449953, 0.3809398316192084688, -16.44928196465088988 ) ) ;
#20554=CARTESIAN_POINT ( 'NONE',  ( -22.72740238869282692, 0.6216207654525480741, -21.61878617671870018 ) ) ;
#20557=CARTESIAN_POINT ( 'NONE',  ( 33.18519186262097520, -5.002662412273467751, -9.016556272618601042 ) ) ;
#20570=EDGE_LOOP ( 'NONE', ( #34428, #15214, #1668, #37274 ) ) ;
#20573=CARTESIAN_POINT ( 'NONE',  ( 5.518227685048840314, 33.48242281877398341, -12.00997661136522510 ) ) ;
#20576=CARTESIAN_POINT ( 'NONE',  ( 12.27390640609045036, -16.43329545370340838, -29.99999999999998934 ) ) ;
#20582=CARTESIAN_POINT ( 'NONE',  ( 14.79314896790873135, 25.75459063161006767, -10.17147167629895144 ) ) ;
#20585=CARTESIAN_POINT ( 'NONE',  ( -11.29390458575034373, 17.10922195600983997, -29.35494707390875746 ) ) ;
#20589=CARTESIAN_POINT ( 'NONE',  ( 14.89811268554684176, 25.43506582924968029, -10.18359384596507056 ) ) ;
#20591=CARTESIAN_POINT ( 'NONE',  ( 32.18353893966516921, -20.39468426946134016, -7.117916671018453378 ) ) ;
#20593=CARTESIAN_POINT ( 'NONE',  ( -14.36325139127783501, 27.43616443481291256, -9.622046172864397562 ) ) ;
#20595=CARTESIAN_POINT ( 'NONE',  ( -16.93610668433033339, -26.60906881091851872, -8.235790559075788053 ) ) ;
#20599=CARTESIAN_POINT ( 'NONE',  ( -19.74691339681017865, -6.824302415588217485, -27.02994878819155034 ) ) ;
#20600=CARTESIAN_POINT ( 'NONE',  ( -14.39692894930127487, -25.73270398672122994, -9.716188519315773320 ) ) ;
#20603=CARTESIAN_POINT ( 'NONE',  ( 20.36878409817081703, 2.417852450439662348, -29.37451754486702171 ) ) ;
#20607=VERTEX_POINT ( 'NONE', #33530 ) ;
#20608=CARTESIAN_POINT ( 'NONE',  ( -20.48447659325206516, 0.7979435291051002466, -29.34725074627716879 ) ) ;
#20609=CARTESIAN_POINT ( 'NONE',  ( 20.86812861272620978, 0.01623219257051957895, -26.76714782918698532 ) ) ;
#20613=CARTESIAN_POINT ( 'NONE',  ( -24.19505052999625150, 1.198773395227752836, -18.53314538056739025 ) ) ;
#20614=CARTESIAN_POINT ( 'NONE',  ( -19.79815887584811307, 19.84782313723621883, -13.42901749168595771 ) ) ;
#20618=AXIS2_PLACEMENT_3D ( 'NONE', #40016, #12194, #24589 ) ;
#20624=CARTESIAN_POINT ( 'NONE',  ( -26.03581645590561422, 5.301338185016732929, -7.395082201969008118 ) ) ;
#20627=CARTESIAN_POINT ( 'NONE',  ( 18.00180999299007212, -17.62873692815191617, -19.82092202452991003 ) ) ;
#20630=CARTESIAN_POINT ( 'NONE',  ( 10.63104621300768216, 17.52826713075782905, -30.00000000000000355 ) ) ;
#20634=CARTESIAN_POINT ( 'NONE',  ( -16.99205359343081057, 21.87216257061389157, -5.475577676556287798 ) ) ;
#20638=CARTESIAN_POINT ( 'NONE',  ( 11.90609510123815262, 19.36740028416927828, -21.61948926389480263 ) ) ;
#20642=CARTESIAN_POINT ( 'NONE',  ( -12.30182166038729008, 20.60945325276725271, -19.47751875586111581 ) ) ;
#20643=CARTESIAN_POINT ( 'NONE',  ( 19.48557158514988075, -11.24999999999998224, 6.000000000000000000 ) ) ;
#20644=CARTESIAN_POINT ( 'NONE',  ( -9.798063751231428142, -18.55837220631304518, -26.22365102716438656 ) ) ;
#20646=CARTESIAN_POINT ( 'NONE',  ( -19.90297529439527935, -11.21068947634444513, -22.98220968216354265 ) ) ;
#20647=CARTESIAN_POINT ( 'NONE',  ( -8.349547994803288020, -23.65591986291670423, -13.74762987334840680 ) ) ;
#20649=CARTESIAN_POINT ( 'NONE',  ( 11.73765114802458953, 17.34560416271227012, -26.28214589256836575 ) ) ;
#20651=CARTESIAN_POINT ( 'NONE',  ( 25.32158894843077945, 6.480252874148680675, -5.000000000000003553 ) ) ;
#20657=CARTESIAN_POINT ( 'NONE',  ( -31.69836596977474485, -1.611888971326790099, -8.225968294365550548 ) ) ;
#20659=CARTESIAN_POINT ( 'NONE',  ( 29.49705578473263756, -0.08617031093297387867, -10.64064826169365752 ) ) ;
#20663=DIRECTION ( 'NONE',  ( 0.000000000000000000, 0.000000000000000000, -1.000000000000000000 ) ) ;
#20673=CARTESIAN_POINT ( 'NONE',  ( 0.3724352543551862627, 34.47678155200587469, -11.97407239485822039 ) ) ;
#20682=CARTESIAN_POINT ( 'NONE',  ( 10.00001779673401714, 18.34526635362476554, -26.72599099279598889 ) ) ;
#20686=CARTESIAN_POINT ( 'NONE',  ( -16.75542722950669372, 12.74032028316595699, -24.38506794022037383 ) ) ;
#20687=CARTESIAN_POINT ( 'NONE',  ( 14.98890121934614506, -28.67928442654198307, -5.000000000000000000 ) ) ;
#20689=CARTESIAN_POINT ( 'NONE',  ( 14.99547355802778981, -25.99396817878668031, -9.237562226852288561 ) ) ;
#20691=CARTESIAN_POINT ( 'NONE',  ( 13.75556773078374029, 23.42751890104277024, -14.47297052992422550 ) ) ;
#20694=CIRCLE ( 'NONE', #29664, 56.99999999999991473 ) ;
#20695=CARTESIAN_POINT ( 'NONE',  ( -27.46546245186472390, -24.32166980333147066, -8.008947335190420347 ) ) ;
#20696=CARTESIAN_POINT ( 'NONE',  ( 2.964953114717667759, -21.10545243889943734, -23.30365150309269850 ) ) ;
#20697=CARTESIAN_POINT ( 'NONE',  ( 11.64865060427507082, 18.29505130955256575, -23.87876004802710739 ) ) ;
#20698=CARTESIAN_POINT ( 'NONE',  ( 18.69768069937141419, 10.45728937905904665, -22.25138797246191302 ) ) ;
#20702=CARTESIAN_POINT ( 'NONE',  ( -7.186746356396819024, 35.16721044838237020, -9.326795472630500683 ) ) ;
#20707=FACE_OUTER_BOUND ( 'NONE', #26866, .T. ) ;
#20709=CARTESIAN_POINT ( 'NONE',  ( -20.68187284593733111, 1.006734202109016429, -27.45854716128443229 ) ) ;
#20711=CARTESIAN_POINT ( 'NONE',  ( 19.87733292414454667, -5.354748204895443564, -28.50879837906193970 ) ) ;
#20729=CARTESIAN_POINT ( 'NONE',  ( 15.39201892520244641, 13.81047332064365740, -27.12305683531639389 ) ) ;
#20730=CARTESIAN_POINT ( 'NONE',  ( 12.14007034441317856, 31.71921406358307038, -8.558348499896236916 ) ) ;
#20732=CARTESIAN_POINT ( 'NONE',  ( -19.68060073398973842, 9.708938446362566310, -20.11576684351307520 ) ) ;
#20735=CARTESIAN_POINT ( 'NONE',  ( 11.00987194897382970, -19.94983946540193998, -21.59411760730909080 ) ) ;
#20736=CARTESIAN_POINT ( 'NONE',  ( 16.77267017469755217, -29.13948811618736912, -5.000000000000003553 ) ) ;
#20738=CARTESIAN_POINT ( 'NONE',  ( -11.30484249362164384, 18.04208246058641052, -25.01387445287749145 ) ) ;
#20741=CARTESIAN_POINT ( 'NONE',  ( 10.95693405366107953, -22.07055394455351305, -17.55030168376832123 ) ) ;
#20748=CARTESIAN_POINT ( 'NONE',  ( -8.456281551504293503, 23.21296397863146410, -20.00008365536006494 ) ) ;
#20753=CARTESIAN_POINT ( 'NONE',  ( 23.28981712441201779, 0.6280063682916672274, -20.55124257728155257 ) ) ;
#20758=CARTESIAN_POINT ( 'NONE',  ( -23.30969975423458962, 0.5725924327717566431, -20.54455488908562799 ) ) ;
#20761=CARTESIAN_POINT ( 'NONE',  ( 32.55711526567240810, -3.964017815489828678, -9.499260478695129351 ) ) ;
#20774=CARTESIAN_POINT ( 'NONE',  ( 8.026644466976325276, 35.55948074244522417, -8.017818322552109578 ) ) ;
#20777=CARTESIAN_POINT ( 'NONE',  ( 12.01726265205634725, -17.15496393756174953, -26.62634840083233101 ) ) ;
#20782=CARTESIAN_POINT ( 'NONE',  ( 15.33163471202798789, 26.81437899606220299, -6.414921594359186408 ) ) ;
#20784=CARTESIAN_POINT ( 'NONE',  ( -11.37750526317191735, 17.29471388271799981, -27.47106155913822434 ) ) ;
#20787=CARTESIAN_POINT ( 'NONE',  ( 11.39223802988129997, 17.97370404759189810, -25.02557645429753919 ) ) ;
#20789=CARTESIAN_POINT ( 'NONE',  ( 31.15403848181932744, -18.43678299216485073, -10.17193552462277850 ) ) ;
#20791=CARTESIAN_POINT ( 'NONE',  ( -15.00988142436982997, 27.11442454588856421, -7.804806528538684063 ) ) ;
#20793=CARTESIAN_POINT ( 'NONE',  ( -17.26829665777506762, -27.06560434691794015, -5.929067903965382413 ) ) ;
#20797=CARTESIAN_POINT ( 'NONE',  ( -34.77897381664745069, -11.95873854617616239, -8.005595432382110133 ) ) ;
#20798=CARTESIAN_POINT ( 'NONE',  ( -14.68417942092947825, -26.35066116812440740, -7.360212364853471634 ) ) ;
#20801=CARTESIAN_POINT ( 'NONE',  ( 20.42176732625024016, 3.104454087777909432, -27.57334092644989099 ) ) ;
#20805=CARTESIAN_POINT ( 'NONE',  ( -27.19884774959017193, 0.1546446106993354663, -14.46771215221622597 ) ) ;
#20807=CARTESIAN_POINT ( 'NONE',  ( 31.32859553683839238, -0.9615075054642621133, -7.789356384682906587 ) ) ;
#20810=CARTESIAN_POINT ( 'NONE',  ( -20.21274638685197900, 3.602405235153209873, -28.78677028190584863 ) ) ;
#20817=EDGE_CURVE ( 'NONE', #17093, #26001, #411, .T. ) ;
#20822=CARTESIAN_POINT ( 'NONE',  ( -25.50981415929211948, 6.214348039242530319, -5.957670977875550555 ) ) ;
#20825=CARTESIAN_POINT ( 'NONE',  ( 20.78379507624259759, -21.64473465098445359, -14.89368447040524401 ) ) ;
#20829=CARTESIAN_POINT ( 'NONE',  ( 11.21809837322889258, 18.66389468805340357, -23.81189286561465934 ) ) ;
#20832=CARTESIAN_POINT ( 'NONE',  ( -16.52695952976914739, 21.08173666875514130, -10.27124637523843909 ) ) ;
#20835=CARTESIAN_POINT ( 'NONE',  ( 15.24827013184445335, 26.35192645322203475, -7.828065716477629721 ) ) ;
#20839=CARTESIAN_POINT ( 'NONE',  ( -12.59192885307270160, 21.14500111850274777, -18.43868266935661637 ) ) ;
#20842=CARTESIAN_POINT ( 'NONE',  ( -14.64184591927359058, -25.46469159694181172, -10.65210004618737472 ) ) ;
#20846=CARTESIAN_POINT ( 'NONE',  ( -30.88206088769906188, -17.38511845617157547, -11.06633628945596826 ) ) ;
#20847=CARTESIAN_POINT ( 'NONE',  ( -6.708033934598859993, -24.40127542935700333, -10.82077489312179708 ) ) ;
#20849=CARTESIAN_POINT ( 'NONE',  ( 12.15869668810743853, 16.64054837370678896, -28.13968978295428514 ) ) ;
#20851=CARTESIAN_POINT ( 'NONE',  ( 24.66102986608180103, 7.389241230280822137, -5.479742525773724893 ) ) ;
#20857=CARTESIAN_POINT ( 'NONE',  ( -30.88014466036690564, -0.7593947357035598644, -8.724960917509704927 ) ) ;
#20858=CARTESIAN_POINT ( 'NONE',  ( 20.61252707005384721, 0.8134334096382831447, -28.07566294656438544 ) ) ;
#20862=CARTESIAN_POINT ( 'NONE',  ( 31.47283671532267846, -25.12609584734865464, -5.000000000000006217 ) ) ;
#20867=DIRECTION ( 'NONE',  ( 0.000000000000000000, 0.000000000000000000, 1.000000000000000000 ) ) ;
#20871=CARTESIAN_POINT ( 'NONE',  ( 0.2990765050996653796, 27.93411067714205487, -17.59605008320459874 ) ) ;
#20872=DIRECTION ( 'NONE',  ( -0.000000000000000000, -0.000000000000000000, -1.000000000000000000 ) ) ;
#20874=DIRECTION ( 'NONE',  ( 0.000000000000000000, 0.000000000000000000, 1.000000000000000000 ) ) ;
#20878=CARTESIAN_POINT ( 'NONE',  ( 14.20869267691362836, 26.79038709246419714, -10.56660588343595464 ) ) ;
#20881=CARTESIAN_POINT ( 'NONE',  ( -16.37425825659163792, 12.35560620482834970, -29.42542551771414594 ) ) ;
#20885=CARTESIAN_POINT ( 'NONE',  ( 9.713596357440627216, -18.43027871082647096, -26.82846153584012683 ) ) ;
#20887=CARTESIAN_POINT ( 'NONE',  ( 15.08986029823985930, 26.17666856099242878, -8.765926281638572348 ) ) ;
#20890=CARTESIAN_POINT ( 'NONE',  ( -29.78193569813405261, -23.30844690436251909, -6.284807164236900334 ) ) ;
#20891=CARTESIAN_POINT ( 'NONE',  ( 1.807847150130388103, -24.69116081338074764, -6.940716909664599754 ) ) ;
#20892=CARTESIAN_POINT ( 'NONE',  ( 11.21279839779214171, 17.40770563166403306, -27.45855351148847845 ) ) ;
#20893=CARTESIAN_POINT ( 'NONE',  ( 17.51797765111094307, 10.67563444151121033, -29.42969723541586191 ) ) ;
#20896=CARTESIAN_POINT ( 'NONE',  ( -4.855647265510516064, 23.93711347774053522, -20.81528965570410250 ) ) ;
#20902=CARTESIAN_POINT ( 'NONE',  ( -29.17550845323054887, 0.2804399698490122605, -10.65921175933714515 ) ) ;
#20903=CARTESIAN_POINT ( 'NONE',  ( 24.07628088510988462, -8.068220623474307018, -19.75074122426856604 ) ) ;
#20904=VERTEX_POINT ( 'NONE', #9532 ) ;
#20917=CARTESIAN_POINT ( 'NONE',  ( 19.53446308848797841, 15.92845161367016971, -5.964120103321279842 ) ) ;
#20918=CARTESIAN_POINT ( 'NONE',  ( 11.37375446201378359, 32.31738641217482666, -8.978749375577956826 ) ) ;
#20920=CARTESIAN_POINT ( 'NONE',  ( -18.99707236034979019, 8.589053938987861514, -25.49571320823188003 ) ) ;
#20924=CARTESIAN_POINT ( 'NONE',  ( 15.24497472440922863, -25.75736537240847568, -10.15205319649687077 ) ) ;
#20925=DIRECTION ( 'NONE',  ( 1.000000000000000000, 0.000000000000000000, 0.000000000000000000 ) ) ;
#20926=CARTESIAN_POINT ( 'NONE',  ( 30.41237130417911771, 3.314011747244131723, -13.58461195433497437 ) ) ;
#20927=CARTESIAN_POINT ( 'NONE',  ( -15.22675634102432873, 26.42529409424080455, -7.827145395733679401 ) ) ;
#20928=CARTESIAN_POINT ( 'NONE',  ( -13.12770624849639844, -15.75833046460326692, -29.27147291310542698 ) ) ;
#20929=CARTESIAN_POINT ( 'NONE',  ( 13.49652603687809815, -25.99346187903743299, -7.838242035372235073 ) ) ;
#20935=CARTESIAN_POINT ( 'NONE',  ( -11.63680257515883554, 32.30205350153836008, -8.540093277045761155 ) ) ;
#20941=CARTESIAN_POINT ( 'NONE',  ( 30.10059063360280263, 0.1020349076090372453, -8.768825504575827878 ) ) ;
#20947=CARTESIAN_POINT ( 'NONE',  ( -21.27402184835637300, 0.7928451952627717514, -25.01640619516613384 ) ) ;
#20950=CARTESIAN_POINT ( 'NONE',  ( 20.38971234282849565, -2.225416161360934897, -29.29214770260603373 ) ) ;
#20959=VERTEX_POINT ( 'NONE', #14174 ) ;
#20965=CARTESIAN_POINT ( 'NONE',  ( 4.836963073857364570, 24.95738821058018075, -19.74021435415385639 ) ) ;
#20969=CARTESIAN_POINT ( 'NONE',  ( 18.49299501565283776, -27.00900116835392950, -7.282676274710347286 ) ) ;
#20975=CARTESIAN_POINT ( 'NONE',  ( 15.37925838865456996, 26.91354363167639363, -5.000000000000000000 ) ) ;
#20977=CARTESIAN_POINT ( 'NONE',  ( -11.43474607271607724, 17.01453699462772207, -29.99999999999999645 ) ) ;
#20980=CARTESIAN_POINT ( 'NONE',  ( 12.47124741220967969, 20.38495263699950044, -19.51041991144671428 ) ) ;
#20982=CARTESIAN_POINT ( 'NONE',  ( 27.40575770944601075, -17.37578260266968044, -13.80665597063403460 ) ) ;
#20984=CARTESIAN_POINT ( 'NONE',  ( -14.84116226840152564, 28.49513596198176657, -5.928569375116603091 ) ) ;
#20986=CARTESIAN_POINT ( 'NONE',  ( -16.19293341369543171, -24.29526116618816189, -13.31600924498339822 ) ) ;
#20991=CARTESIAN_POINT ( 'NONE',  ( -19.95518743367748726, -6.895742946619512814, -26.33169168298753604 ) ) ;
#20992=CARTESIAN_POINT ( 'NONE',  ( -14.64167027567601487, -25.91586225274019029, -9.242477963831079890 ) ) ;
#20995=CARTESIAN_POINT ( 'NONE',  ( 20.26233914688108229, 3.111977874782128062, -30.00000000000000000 ) ) ;
#20997=COLOUR_RGB ( '', 0.31764706, 0.68627451, 0.89019608) ;
#21000=CARTESIAN_POINT ( 'NONE',  ( -24.59124188716270609, 0.3669073574842401930, -18.44339233438290293 ) ) ;
#21002=CARTESIAN_POINT ( 'NONE',  ( 32.12080372859628596, -1.419867088699604984, -5.466234668651527073 ) ) ;
#21006=CARTESIAN_POINT ( 'NONE',  ( -27.98824911009742422, 2.633740639151773255, -8.327080751032047701 ) ) ;
#21009=CIRCLE ( 'NONE', #34632, 17.99999999999990052 ) ;
#21017=CARTESIAN_POINT ( 'NONE',  ( -25.42975317007962488, 6.206975593436134808, -6.919413500419955732 ) ) ;
#21018=CARTESIAN_POINT ( 'NONE',  ( 15.41558956984165363, 26.78481017248027740, 0.000000000000000000 ) ) ;
#21020=CARTESIAN_POINT ( 'NONE',  ( 26.28907122124725149, -25.68141371849936405, -5.873759093919935559 ) ) ;
#21022=CARTESIAN_POINT ( 'NONE',  ( 14.86242357273094683, 26.45546649154326246, -9.214439520639988501 ) ) ;
#21026=CARTESIAN_POINT ( 'NONE',  ( -16.27617705945219839, 20.65743945337694853, -11.73023920987073510 ) ) ;
#21029=CARTESIAN_POINT ( 'NONE',  ( 14.04032970691909732, 23.91029121590017681, -13.51430497135585895 ) ) ;
#21032=EDGE_LOOP ( 'NONE', ( #3882, #37315 ) ) ;
#21033=CARTESIAN_POINT ( 'NONE',  ( -15.35513899590904430, 26.99708482749830907, -5.473155708056963498 ) ) ;
#21035=CARTESIAN_POINT ( 'NONE',  ( -9.836635315125095147, -18.54107557745045654, -26.21993274389535244 ) ) ;
#21038=CARTESIAN_POINT ( 'NONE',  ( -17.55945971783640758, -10.59693620792911872, -30.00000000000001421 ) ) ;
#21039=CARTESIAN_POINT ( 'NONE',  ( -9.876522206958991745, -22.96841405707892037, -15.64990654850994822 ) ) ;
#21041=CARTESIAN_POINT ( 'NONE',  ( 12.18916105282683304, 16.70401724222313788, -27.52870704815159186 ) ) ;
#21044=CARTESIAN_POINT ( 'NONE',  ( 20.57897257680733460, 5.989271796650077029, -23.20797897217266126 ) ) ;
#21049=CARTESIAN_POINT ( 'NONE',  ( -21.42004826045867816, -0.5745119313267001981, -24.86738022874436638 ) ) ;
#21051=CARTESIAN_POINT ( 'NONE',  ( 20.69644567353984499, 0.8041823441500935976, -27.44559075125846093 ) ) ;
#21060=LINE ( 'NONE', #2576, #12608 ) ;
#21065=CARTESIAN_POINT ( 'NONE',  ( 1.544216759713194165, 37.43288271813057833, -8.405430002237888942 ) ) ;
#21073=CARTESIAN_POINT ( 'NONE',  ( 9.553997640115609258, 18.14112040201965925, -29.99999999999999645 ) ) ;
#21076=CARTESIAN_POINT ( 'NONE',  ( -18.56352605694899083, 15.93433109089512101, -11.84711699134787111 ) ) ;
#21079=CARTESIAN_POINT ( 'NONE',  ( 10.53369465903642244, -19.57651849404395961, -22.73532858526640510 ) ) ;
#21081=CARTESIAN_POINT ( 'NONE',  ( 11.16181463136529040, 17.77262720094327975, -26.22243848669149813 ) ) ;
#21083=CARTESIAN_POINT ( 'NONE',  ( 15.29245034862073460, 32.56469986092002955, -13.99876745781544685 ) ) ;
#21087=CARTESIAN_POINT ( 'NONE',  ( -28.62642820236494501, -22.44600169765076814, -9.303848538514403188 ) ) ;
#21088=CARTESIAN_POINT ( 'NONE',  ( -2.525287455661448632, -24.41780038572089850, -9.392889257882757192 ) ) ;
#21089=CARTESIAN_POINT ( 'NONE',  ( 12.15359677241966629, 19.10405381618496889, -21.66180759330809380 ) ) ;
#21091=CARTESIAN_POINT ( 'NONE',  ( 17.94274596522729937, 10.05102289979594232, -28.30046506151757768 ) ) ;
#21093=CARTESIAN_POINT ( 'NONE',  ( -4.680396452074460534, 32.75778677526109561, -12.91952194480230176 ) ) ;
#21099=CARTESIAN_POINT ( 'NONE',  ( -30.36706297773999097, 0.4086613843392599699, -6.417692154602818277 ) ) ;
#21100=CARTESIAN_POINT ( 'NONE',  ( 31.93250169833669716, -9.587213356856551627, -12.05150297994976327 ) ) ;
#21116=CARTESIAN_POINT ( 'NONE',  ( 29.26826387686844910, -23.91120845623157010, -5.438285388144263877 ) ) ;
#21117=CARTESIAN_POINT ( 'NONE',  ( 19.95486563595593310, 14.86767224104078977, -7.423818949657161603 ) ) ;
#21118=CARTESIAN_POINT ( 'NONE',  ( 12.41906572600498926, 32.58765353250298347, -4.999999999999998224 ) ) ;
#21120=CARTESIAN_POINT ( 'NONE',  ( -21.60396578388440858, 10.50237655917392310, -11.87878979233392762 ) ) ;
#21123=CARTESIAN_POINT ( 'NONE',  ( 9.902073939236615274, -18.51143114917217503, -26.21360673141550635 ) ) ;
#21125=CARTESIAN_POINT ( 'NONE',  ( 16.24796006241085422, 15.88921519459651144, -30.00000000000001421 ) ) ;
#21126=CARTESIAN_POINT ( 'NONE',  ( -12.91698160810270934, 21.67206672448811133, -17.43500531611570636 ) ) ;
#21127=CARTESIAN_POINT ( 'NONE',  ( -24.70057832354312666, -26.06393885949841760, -7.180590994032729490 ) ) ;
#21128=CARTESIAN_POINT ( 'NONE',  ( 13.69821889811312410, -26.30560278297641830, -5.474065301971783981 ) ) ;
#21132=CARTESIAN_POINT ( 'NONE',  ( -6.249731466780908740, 20.89879465126994518, -24.45472809205353926 ) ) ;
#21140=CARTESIAN_POINT ( 'NONE',  ( 30.28856303283004081, 0.06353136651604823770, -8.298345987469021523 ) ) ;
#21141=CARTESIAN_POINT ( 'NONE',  ( -37.48557158514985588, -11.24999999999982414, 3.000000000000000000 ) ) ;
#21144=CARTESIAN_POINT ( 'NONE',  ( -29.35000585794652395, 0.07926546081450050463, -10.65361827406238149 ) ) ;
#21147=CARTESIAN_POINT ( 'NONE',  ( 21.47608197099559391, -2.388604051638352654, -24.67957022850504956 ) ) ;
#21160=CARTESIAN_POINT ( 'NONE',  ( 8.119369784788442956, 36.07111323917224865, -6.725600398549506309 ) ) ;
#21167=CARTESIAN_POINT ( 'NONE',  ( 12.46065444517352283, -16.66684880058570073, -27.23723484178347221 ) ) ;
#21172=CARTESIAN_POINT ( 'NONE',  ( 12.09851136747228217, 19.96279823048476132, -20.53435459044266054 ) ) ;
#21174=CARTESIAN_POINT ( 'NONE',  ( -15.42498320908520704, 26.75103934920171511, -5.000000000000002665 ) ) ;
#21176=CARTESIAN_POINT ( 'NONE',  ( 9.458291886585664443, -18.18766449894053849, -30.00000000000000000 ) ) ;
#21178=CARTESIAN_POINT ( 'NONE',  ( 15.07386490424905467, 25.79242186437713613, -9.240524828524506518 ) ) ;
#21180=CARTESIAN_POINT ( 'NONE',  ( 22.16801406757617343, -13.11526815166102544, -19.62611364897102106 ) ) ;
#21182=CARTESIAN_POINT ( 'NONE',  ( -14.80950393188541092, 28.42383370304063916, -6.390113609832926755 ) ) ;
#21184=CARTESIAN_POINT ( 'NONE',  ( -11.41242022595238126, -17.75887984712721845, -26.06507157920607654 ) ) ;
#21187=CARTESIAN_POINT ( 'NONE',  ( -25.85792922089648371, -9.778323470226343517, -17.66350960614173715 ) ) ;
#21188=CARTESIAN_POINT ( 'NONE',  ( -15.05356374896470584, -26.34688506717603929, -7.828843382777417759 ) ) ;
#21191=CARTESIAN_POINT ( 'NONE',  ( 28.97456723585821692, 1.148426348366920591, -9.256809715960919505 ) ) ;
#21197=CARTESIAN_POINT ( 'NONE',  ( -30.97418125221157226, -0.1138930278413790714, -4.999999999999999112 ) ) ;
#21199=CARTESIAN_POINT ( 'NONE',  ( 30.43325519101775356, -1.251503160527801528, -10.55494845371857693 ) ) ;
#21202=CARTESIAN_POINT ( 'NONE',  ( -24.96329531792162726, 3.513752566392065901, -14.68029723533687303 ) ) ;
#21211=CARTESIAN_POINT ( 'NONE',  ( -24.18815070014865398, 8.032309469253892331, -5.962252224280692126 ) ) ;
#21214=CARTESIAN_POINT ( 'NONE',  ( 20.14663775004962076, -19.75195631921120665, -16.78371938112692519 ) ) ;
#21216=CARTESIAN_POINT ( 'NONE',  ( 10.89766637450477837, 17.61927834571792317, -27.43414935101323948 ) ) ;
#21220=CARTESIAN_POINT ( 'NONE',  ( -16.92840057844002644, 21.76311522583030822, -6.905117785391271745 ) ) ;
#21224=CARTESIAN_POINT ( 'NONE',  ( 11.00857322187251164, 17.29338995577434446, -29.34887577826749805 ) ) ;
#21228=CARTESIAN_POINT ( 'NONE',  ( -12.32989360994015549, 20.57215784758508548, -19.48341777572011324 ) ) ;
#21230=CARTESIAN_POINT ( 'NONE',  ( -15.50788136758524693, -26.74767648567673817, -5.474109841062610116 ) ) ;
#21233=CARTESIAN_POINT ( 'NONE',  ( -18.08564274236685776, -10.18792848139066543, -27.70420942370164141 ) ) ;
#21234=CARTESIAN_POINT ( 'NONE',  ( -7.966395251936380539, -19.90518285585014979, -24.10536815931465426 ) ) ;
#21236=CARTESIAN_POINT ( 'NONE',  ( 12.11158980248019645, 16.54297856518634902, -29.37115136132677762 ) ) ;
#21237=ORIENTED_EDGE ( 'NONE', *, *, #13340, .T. ) ;
#21238=CARTESIAN_POINT ( 'NONE',  ( 20.85536741361552160, 6.013920567586717780, -22.11640438643503614 ) ) ;
#21245=CARTESIAN_POINT ( 'NONE',  ( -30.25467497739411726, -0.7069905369280371499, -10.12455798544348440 ) ) ;
#21246=CARTESIAN_POINT ( 'NONE',  ( 30.63389016003661780, -0.1680630686027007048, -7.820899855639765086 ) ) ;
#21247=CARTESIAN_POINT ( 'NONE',  ( -19.48557158514985588, -11.25000000000002309, 3.000000000000000000 ) ) ;
#21249=CARTESIAN_POINT ( 'NONE',  ( 30.41237130417911771, 3.314011747244134387, -4.999999999999999112 ) ) ;
#21260=CARTESIAN_POINT ( 'NONE',  ( 3.871220829879935099, 38.02450267464935507, -5.436529868897947537 ) ) ;
#21267=CARTESIAN_POINT ( 'NONE',  ( 13.18225496512505757, 24.59173741764900356, -14.35579410304919534 ) ) ;
#21270=CARTESIAN_POINT ( 'NONE',  ( -16.06070315713033025, 13.11638197811575246, -26.58602791737893156 ) ) ;
#21271=CARTESIAN_POINT ( 'NONE',  ( -34.47241746879593904, 3.460351812918829761, 3.000000000000000000 ) ) ;
#21273=CARTESIAN_POINT ( 'NONE',  ( 14.96192828012108578, -25.98634713340315017, -9.238541611499263340 ) ) ;
#21274=CARTESIAN_POINT ( 'NONE',  ( -20.76418541913865923, -26.08974834292795109, -9.464979353182689792 ) ) ;
#21276=CARTESIAN_POINT ( 'NONE',  ( 15.09217338382007689, 26.16895268490867821, -8.766269268417817173 ) ) ;
#21281=AXIS2_PLACEMENT_3D ( 'NONE', #16247, #19897, #22726 ) ;
#21283=CARTESIAN_POINT ( 'NONE',  ( -22.05305370367605278, -18.37986245703921284, -16.69510183025791505 ) ) ;
#21284=CARTESIAN_POINT ( 'NONE',  ( -0.3897205959626178773, -24.77793770357540737, -5.000000000000000888 ) ) ;
#21285=CARTESIAN_POINT ( 'NONE',  ( 13.70661370344850560, 22.39768893898365221, -15.48108906342483415 ) ) ;
#21286=CARTESIAN_POINT ( 'NONE',  ( 22.20551005480023576, 11.09721735243621588, -5.966899065133762114 ) ) ;
#21288=CARTESIAN_POINT ( 'NONE',  ( -3.735156488784892481, 26.39161017904735829, -18.66586346394144158 ) ) ;
#21292=CARTESIAN_POINT ( 'NONE',  ( -34.41928798828883629, -5.508411629658334974, -5.895573557013064736 ) ) ;
#21299=CARTESIAN_POINT ( 'NONE',  ( -23.18519655538999658, 0.9190088410037334787, -20.58602323490189789 ) ) ;
#21300=CARTESIAN_POINT ( 'NONE',  ( 33.79199353566443875, -13.57530639058761679, -9.302689660099131785 ) ) ;
#21313=CARTESIAN_POINT ( 'NONE',  ( -1.746686391856493215, 21.93407269432965379, -24.23685970402688383 ) ) ;
#21318=CARTESIAN_POINT ( 'NONE',  ( 27.74479198965729410, -21.38649675605601885, -11.08839524368410601 ) ) ;
#21319=CARTESIAN_POINT ( 'NONE',  ( 20.01142798620482921, 14.91867193257671431, -6.451173775806654298 ) ) ;
#21320=CARTESIAN_POINT ( 'NONE',  ( 11.04322220929187104, 28.65258582978126256, -13.13952990371131513 ) ) ;
#21321=ORIENTED_EDGE ( 'NONE', *, *, #23505, .F. ) ;
#21323=CARTESIAN_POINT ( 'NONE',  ( -18.43203766348224804, 9.199961657135451887, -27.73406356219650704 ) ) ;
#21325=CARTESIAN_POINT ( 'NONE',  ( 12.04973099137657755, -21.47510576933752091, -18.43454808460629124 ) ) ;
#21328=CARTESIAN_POINT ( 'NONE',  ( -11.87729697930262951, 19.39812291060849603, -21.61417898203982801 ) ) ;
#21329=CARTESIAN_POINT ( 'NONE',  ( -13.82671766433831095, -15.58877518772614046, -27.14361040387732160 ) ) ;
#21330=CARTESIAN_POINT ( 'NONE',  ( 8.649194241449905007, -18.71206457532732514, -28.12513526114011952 ) ) ;
#21334=CARTESIAN_POINT ( 'NONE',  ( -9.013010211479819844, 27.20962005112951942, -15.91364778940325486 ) ) ;
#21343=CARTESIAN_POINT ( 'NONE',  ( 23.31464182441019872, 0.5588091542327003891, -20.54288570421724458 ) ) ;
#21348=CARTESIAN_POINT ( 'NONE',  ( -30.47171451085012706, 0.001944469067151908051, -7.827869195058648977 ) ) ;
#21351=CARTESIAN_POINT ( 'NONE',  ( 27.02919598657182831, -4.767359354157993501, -16.93437983263991953 ) ) ;
#21363=CARTESIAN_POINT ( 'NONE',  ( 5.245106710023661023, 26.98899556905067598, -17.69490459739507671 ) ) ;
#21366=CARTESIAN_POINT ( 'NONE',  ( 11.24817812657392224, -17.21924521237894368, -28.63632236487146798 ) ) ;
#21372=CARTESIAN_POINT ( 'NONE',  ( -11.09715496686145819, 17.48622750951172833, -27.44966945835485816 ) ) ;
#21374=CARTESIAN_POINT ( 'NONE',  ( 9.447256496083108246, -18.24336034194182687, -28.70984161428601666 ) ) ;
#21378=CARTESIAN_POINT ( 'NONE',  ( -10.24004248254194316, 18.41327472192288539, -26.12338179500006419 ) ) ;
#21380=CARTESIAN_POINT ( 'NONE',  ( -19.26074050860073328, -27.02685104100921620, -7.267539198847054571 ) ) ;
#21383=CARTESIAN_POINT ( 'NONE',  ( -30.96917735819973672, -10.61658571351321356, -12.94788124637345206 ) ) ;
#21384=CARTESIAN_POINT ( 'NONE',  ( -11.65776438499378109, -21.50447217315263870, -18.47646201114688225 ) ) ;
#21387=CARTESIAN_POINT ( 'NONE',  ( 26.98308923628663791, 0.4609988587420678074, -14.49164037743313926 ) ) ;
#21392=CARTESIAN_POINT ( 'NONE',  ( -21.72644794604407537, 0.6368340560596529309, -23.84291411478136880 ) ) ;
#21394=CARTESIAN_POINT ( 'NONE',  ( 31.73450339093934858, -1.000272218596043761, -5.933748666415237238 ) ) ;
#21399=CARTESIAN_POINT ( 'NONE',  ( -27.01695987841192093, 3.517937595036570997, -9.299659907420654292 ) ) ;
#21405=DIRECTION ( 'NONE',  ( -0.000000000000000000, -0.000000000000000000, -1.000000000000000000 ) ) ;
#21408=CARTESIAN_POINT ( 'NONE',  ( -23.81473431349828829, 6.976256285597340678, -11.82319584038477522 ) ) ;
#21412=CARTESIAN_POINT ( 'NONE',  ( 14.45205179786681882, -15.04654671938721400, -27.10327764158452268 ) ) ;
#21414=CARTESIAN_POINT ( 'NONE',  ( 10.80899027733819295, 17.41890095272876593, -30.00000000000000000 ) ) ;
#21417=CARTESIAN_POINT ( 'NONE',  ( -15.42122190845770646, 23.49383705188275329, -10.69673651877608478 ) ) ;
#21420=CARTESIAN_POINT ( 'NONE',  ( 15.18681916921612363, 26.24042416626922503, -8.298040651035869075 ) ) ;
#21425=CARTESIAN_POINT ( 'NONE',  ( -15.31970618788670180, 27.02672079109983727, -5.943192127738577746 ) ) ;
#21427=CARTESIAN_POINT ( 'NONE',  ( -11.69740102143367544, -20.95835256283988102, -19.47752585436962036 ) ) ;
#21429=CARTESIAN_POINT ( 'NONE',  ( -34.01753683000946893, -17.82260201088918450, -5.856192742791406225 ) ) ;
#21430=CARTESIAN_POINT ( 'NONE',  ( -13.89005016234717971, -26.28256486574421658, -6.419270497917506368 ) ) ;
#21432=CARTESIAN_POINT ( 'NONE',  ( 15.50276458342831987, 23.27946725895370861, -10.70176112796715095 ) ) ;
#21434=CARTESIAN_POINT ( 'NONE',  ( 23.64686652105454812, 7.232955847004403971, -11.82926767496736353 ) ) ;
#21438=CARTESIAN_POINT ( 'NONE',  ( -20.03448507352192465, -26.57026294638366437, -8.593633122198326646 ) ) ;
#21440=CARTESIAN_POINT ( 'NONE',  ( -31.98245490244095635, -1.244365697959704420, -5.000000000000000000 ) ) ;
#21442=CARTESIAN_POINT ( 'NONE',  ( 27.79148596755621625, 0.1202762638927254851, -13.50639119845660119 ) ) ;
#21448=CARTESIAN_POINT ( 'NONE',  ( 35.36940577612500647, -20.42053594592276866, -4.999999999999997335 ) ) ;
#21449=CARTESIAN_POINT ( 'NONE',  ( 19.48557158514975285, -11.24999999999995737, 10.00000000000000000 ) ) ;
#21451=CARTESIAN_POINT ( 'NONE',  ( -15.48853126089653642, -26.74269726827072446, -4.999999999999999112 ) ) ;
#21454=CARTESIAN_POINT ( 'NONE',  ( 3.763558953900551618, 36.71453398273495594, -8.854024335422799652 ) ) ;
#21463=CARTESIAN_POINT ( 'NONE',  ( 14.75730607214175905, 27.52521798300531586, -8.251418156868062681 ) ) ;
#21466=CARTESIAN_POINT ( 'NONE',  ( -15.47687725686822802, 14.82734777190539077, -23.20797657644519418 ) ) ;
#21470=CARTESIAN_POINT ( 'NONE',  ( 9.970553079590814605, -18.81210375092922149, -25.01410075462041149 ) ) ;
#21471=CARTESIAN_POINT ( 'NONE',  ( -19.52232064119460375, -24.60346519530635589, -12.21144919225334213 ) ) ;
#21473=CARTESIAN_POINT ( 'NONE',  ( 10.97317656914242967, 17.31587133052951089, -29.34811157007365523 ) ) ;
#21476=CARTESIAN_POINT ( 'NONE',  ( -14.53998467467461353, -25.44454797919701505, -10.65503318047344194 ) ) ;
#21478=CARTESIAN_POINT ( 'NONE',  ( -16.88793822083986740, -14.03095869258871531, -24.29931205907291769 ) ) ;
#21479=CARTESIAN_POINT ( 'NONE',  ( 1.255466122108702232, -20.65231545638951616, -27.17923991438529185 ) ) ;
#21480=CARTESIAN_POINT ( 'NONE',  ( 14.97130663709144294, 24.72598064263621609, -10.66823142197542928 ) ) ;
#21481=CARTESIAN_POINT ( 'NONE',  ( 18.10664311642079483, 11.05995638511404167, -23.33310058690642919 ) ) ;
#21484=CARTESIAN_POINT ( 'NONE',  ( -3.705086238427029777, 21.62874139591992773, -24.30186519092085362 ) ) ;
#21486=CARTESIAN_POINT ( 'NONE',  ( -34.30668518109128939, -6.458525508014972161, -7.647112954010694352 ) ) ;
#21492=CARTESIAN_POINT ( 'NONE',  ( -20.66892949074973984, 1.176045066688247598, -27.46922783559482895 ) ) ;
#21493=CARTESIAN_POINT ( 'NONE',  ( 33.95993763334963234, -12.46657790436312752, -9.313543929707535085 ) ) ;
#21494=AXIS2_PLACEMENT_3D ( 'NONE', #25205, #37603, #9770 ) ;
#21503=CARTESIAN_POINT ( 'NONE',  ( -2.962397377419403899, 36.59740967881665341, -9.288886632304988566 ) ) ;
#21509=CARTESIAN_POINT ( 'NONE',  ( 27.03181137051826255, -20.83723433176508166, -11.99698614993629064 ) ) ;
#21511=CARTESIAN_POINT ( 'NONE',  ( 16.48441032495264835, 12.78878735330096994, -25.47995477096423755 ) ) ;
#21512=CARTESIAN_POINT ( 'NONE',  ( 8.265145098949810532, 19.28472743380562804, -26.57823981897835708 ) ) ;
#21514=CARTESIAN_POINT ( 'NONE',  ( -21.33856562183509098, 11.52826686442322845, -10.38518463479564957 ) ) ;
#21516=CARTESIAN_POINT ( 'NONE',  ( 12.00181538804464232, -21.47850077996891471, -18.44043584019166104 ) ) ;
#21518=CARTESIAN_POINT ( 'NONE',  ( 19.54664213359407654, -11.28525909758385914, -19.69475445967423610 ) ) ;
#21519=CARTESIAN_POINT ( 'NONE',  ( -12.11165721293594544, 19.94706872364197281, -20.53702604530188935 ) ) ;
#21522=CARTESIAN_POINT ( 'NONE',  ( -14.83625493676444052, -17.72904731969334691, -22.21157065729462232 ) ) ;
#21523=CARTESIAN_POINT ( 'NONE',  ( 12.69900848833330187, -25.52681193209280153, -9.268119605047994369 ) ) ;
#21526=CARTESIAN_POINT ( 'NONE',  ( -8.291105163447188175, 27.72608485885197638, -15.86983220121024729 ) ) ;
#21532=CARTESIAN_POINT ( 'NONE',  ( 23.30637526650272662, 0.5818651227441539175, -20.54567832033172792 ) ) ;
#21538=CARTESIAN_POINT ( 'NONE',  ( -22.21240959074407684, 0.6992048922518714349, -22.73936558975926658 ) ) ;
#21541=CARTESIAN_POINT ( 'NONE',  ( 22.77169554655636219, -3.983247555766573189, -22.21157357009845512 ) ) ;
#21558=CARTESIAN_POINT ( 'NONE',  ( 4.496862015843431593, 20.00989232716073118, -29.23636761809433082 ) ) ;
#21561=CARTESIAN_POINT ( 'NONE',  ( 15.53547054105565373, -24.29315558060116231, -13.36240988604506263 ) ) ;
#21562=FACE_OUTER_BOUND ( 'NONE', #28702, .T. ) ;
#21566=CARTESIAN_POINT ( 'NONE',  ( -15.03387384203356270, 25.91884056606313536, -9.238937710698264638 ) ) ;
#21569=CARTESIAN_POINT ( 'NONE',  ( 10.44557952003627221, -19.60207686399620286, -22.74606572134008431 ) ) ;
#21571=VERTEX_POINT ( 'NONE', #34616 ) ;
#21573=CARTESIAN_POINT ( 'NONE',  ( -10.38118103384230828, 18.73610608265249766, -24.88814054586562818 ) ) ;
#21574=CARTESIAN_POINT ( 'NONE',  ( -14.44439269762431977, -21.86739633494050139, -17.20223798650874869 ) ) ;
#21578=CARTESIAN_POINT ( 'NONE',  ( -19.82898810763364494, -5.533127045182635761, -28.50453774944905661 ) ) ;
#21579=CARTESIAN_POINT ( 'NONE',  ( -15.28548941152575402, -26.69066991962944257, -5.000000000000000888 ) ) ;
#21581=EDGE_LOOP ( 'NONE', ( #1282, #5941, #39309, #28731 ) ) ;
#21582=CARTESIAN_POINT ( 'NONE',  ( 30.64962079249725946, 0.2186612821100236970, -5.000000000000000000 ) ) ;
#21586=CARTESIAN_POINT ( 'NONE',  ( -30.50745882448537927, -0.03539364285743687444, -7.826725409455514537 ) ) ;
#21588=CARTESIAN_POINT ( 'NONE',  ( 32.12760839428420212, -2.228125769087125896, -8.203263732686945531 ) ) ;
#21589=CIRCLE ( 'NONE', #26781, 17.00000000000000000 ) ;
#21590=CARTESIAN_POINT ( 'NONE',  ( 6.128519550197534471, -19.61146684927020090, -30.00000000000000711 ) ) ;
#21594=CARTESIAN_POINT ( 'NONE',  ( -23.09610976977102936, 3.527081606721067075, -18.74855405513135409 ) ) ;
#21604=CARTESIAN_POINT ( 'NONE',  ( -20.11046056464997633, 6.477547240074802204, -24.32480941670467089 ) ) ;
#21607=CARTESIAN_POINT ( 'NONE',  ( 20.57510288040941049, -22.72408697488640783, -13.98806764414992898 ) ) ;
#21609=CARTESIAN_POINT ( 'NONE',  ( 15.02598156427579568, 26.38482746277715307, -8.756742615304116129 ) ) ;
#21612=CARTESIAN_POINT ( 'NONE',  ( -12.90072778892209904, 17.70939849946352851, -22.91841346334786422 ) ) ;
#21614=VECTOR ( 'NONE', #36867, 1000.000000000000000 ) ;
#21615=CARTESIAN_POINT ( 'NONE',  ( 17.34253826607186255, 27.32041144404028543, -5.000000000000000000 ) ) ;
#21616=CARTESIAN_POINT ( 'NONE',  ( 11.06077487293502593, 17.41132527382090700, -28.07864658204483277 ) ) ;
#21620=CARTESIAN_POINT ( 'NONE',  ( -14.73753967824242572, 25.92079578855301847, -10.16159616314446268 ) ) ;
#21622=CARTESIAN_POINT ( 'NONE',  ( -9.570498547032590508, -18.18000853095062297, -28.70499904869090102 ) ) ;
#21626=CARTESIAN_POINT ( 'NONE',  ( -18.37356219290808568, -9.636757534816835502, -27.70765190437884939 ) ) ;
#21627=CARTESIAN_POINT ( 'NONE',  ( -8.733449382607537004, -18.59056498759259313, -28.73589422697259366 ) ) ;
#21629=CARTESIAN_POINT ( 'NONE',  ( 14.40945247603743340, 22.05875077139578266, -14.55621836163558847 ) ) ;
#21631=CARTESIAN_POINT ( 'NONE',  ( 23.77809889112756991, 5.422375568838193161, -14.77688470156370038 ) ) ;
#21636=CARTESIAN_POINT ( 'NONE',  ( -31.00339467208933542, -1.147717236077904213, -9.169194955842794315 ) ) ;
#21638=CARTESIAN_POINT ( 'NONE',  ( 31.15015558338321711, -0.2976252405140638047, -5.472529613951848226 ) ) ;
#21643=CARTESIAN_POINT ( 'NONE',  ( 20.90924525106828114, -8.502318254486461058, -19.80438750953544513 ) ) ;
#21649=PLANE ( 'NONE',  #24218 ) ;
#21650=CARTESIAN_POINT ( 'NONE',  ( 2.482818899334112928, 24.48995573783189528, -20.72365887979838206 ) ) ;
#21658=CARTESIAN_POINT ( 'NONE',  ( 15.01573743325078070, 27.63731046468882724, -6.866476842728680197 ) ) ;
#21661=CARTESIAN_POINT ( 'NONE',  ( -18.09191307318060993, 16.86591247271400107, -11.82766105011013380 ) ) ;
#21666=CARTESIAN_POINT ( 'NONE',  ( 9.571804183446699810, -18.27277504971789668, -28.07733812879041935 ) ) ;
#21668=CARTESIAN_POINT ( 'NONE',  ( -21.33353929772287216, -26.74474634351298974, -7.673098688866929251 ) ) ;
#21669=CYLINDRICAL_SURFACE ( 'NONE', #32112, 21.00000000000001776 ) ;
#21670=CARTESIAN_POINT ( 'NONE',  ( 12.64671789796098444, 21.06331887642912548, -18.45078820372820871 ) ) ;
#21674=CARTESIAN_POINT ( 'NONE',  ( -14.96192385577551853, -26.11888079852932876, -8.768824939043708966 ) ) ;
#21676=VECTOR ( 'NONE', #22447, 1000.000000000000000 ) ;
#21677=CARTESIAN_POINT ( 'NONE',  ( -29.86115101714491260, -23.36578077687985200, -5.861277548232656898 ) ) ;
#21678=CARTESIAN_POINT ( 'NONE',  ( -2.597410653098545907, -24.79173595445318767, -5.482757586617159618 ) ) ;
#21679=CARTESIAN_POINT ( 'NONE',  ( 11.95174086388698953, 18.65537474512603922, -22.77781173593105279 ) ) ;
#21681=CARTESIAN_POINT ( 'NONE',  ( 22.68038563371576899, 10.11994014617707727, -7.424820902145242485 ) ) ;
#21683=CARTESIAN_POINT ( 'NONE',  ( -3.169894294691394165, 22.54309369389885020, -23.04265340177524735 ) ) ;
#21685=CARTESIAN_POINT ( 'NONE',  ( -24.35958059579095902, -4.502232839367173334, -19.97906599432332087 ) ) ;
#21693=CARTESIAN_POINT ( 'NONE',  ( -29.66265100694612045, 0.8681446443984893735, -7.834569626181125734 ) ) ;
#21694=CARTESIAN_POINT ( 'NONE',  ( 35.42505292462669786, -13.05524145712385042, -5.438507544938067539 ) ) ;
#21704=CARTESIAN_POINT ( 'NONE',  ( -3.065405920905819759, 38.15199578371129263, -5.857520754517073769 ) ) ;
#21708=CARTESIAN_POINT ( 'NONE',  ( 25.46576935384675622, -20.87028045292102263, -12.93180561768287617 ) ) ;
#21709=CARTESIAN_POINT ( 'NONE',  ( 15.86706096491193385, 13.22493649639811508, -27.13960584726105196 ) ) ;
#21710=CARTESIAN_POINT ( 'NONE',  ( 12.57008845403963804, 30.17714168556475229, -9.943509663025896117 ) ) ;
#21713=CARTESIAN_POINT ( 'NONE',  ( -17.79840780512438769, 10.58908824627457257, -26.62318974669575056 ) ) ;
#21715=CARTESIAN_POINT ( 'NONE',  ( 9.643767478264347659, -18.09000205506835712, -29.34533616503313525 ) ) ;
#21717=CARTESIAN_POINT ( 'NONE',  ( 37.49625565938770677, -14.69322820095495530, -14.45070082761205832 ) ) ;
#21719=CARTESIAN_POINT ( 'NONE',  ( -15.27656269013936985, 26.57811910751880191, -7.356432126642811653 ) ) ;
#21720=CARTESIAN_POINT ( 'NONE',  ( -23.88751137688053561, -26.63245304365073807, -5.447315017795344438 ) ) ;
#21721=CARTESIAN_POINT ( 'NONE',  ( 8.584620562788320086, -18.61902014996657684, -29.36583904130536027 ) ) ;
#21724=CARTESIAN_POINT ( 'NONE',  ( -10.38219465376270101, 31.39154972851433101, -11.21545975099760817 ) ) ;
#21729=CARTESIAN_POINT ( 'NONE',  ( 20.48156205581511458, 0.8692611811187750392, -29.34855215404837381 ) ) ;
#21732=EDGE_CURVE ( 'NONE', #12299, #12248, #34162, .T. ) ;
#21734=CARTESIAN_POINT ( 'NONE',  ( -20.52601294777450036, 0.8771626251181813272, -28.70764666120362918 ) ) ;
#21737=CARTESIAN_POINT ( 'NONE',  ( 25.28008582448413222, -5.224672493644258786, -18.90502067835477717 ) ) ;
#21752=CARTESIAN_POINT ( 'NONE',  ( 5.158612383331919737, 20.07816763940033411, -27.79035459442517109 ) ) ;
#21755=CARTESIAN_POINT ( 'NONE',  ( 18.18730782112094246, -26.61009966856806130, -8.649289542032247979 ) ) ;
#21761=CARTESIAN_POINT ( 'NONE',  ( -14.64327399112337780, 24.66794574669921047, -11.60795671540694940 ) ) ;
#21765=CARTESIAN_POINT ( 'NONE',  ( 9.421039322076820710, -18.20697522973744498, -29.34992098691236251 ) ) ;
#21769=CARTESIAN_POINT ( 'NONE',  ( -13.74168852163965582, 30.17666712228406922, -7.268198090464257355 ) ) ;
#21770=CARTESIAN_POINT ( 'NONE',  ( -19.54254085204202696, -25.96847084744576151, -9.956545142502918111 ) ) ;
#21773=CARTESIAN_POINT ( 'NONE',  ( -35.11119181084233531, -9.814895828461905225, -7.164001942392926203 ) ) ;
#21774=CARTESIAN_POINT ( 'NONE',  ( -9.700341350330687007, -18.60197822309132576, -26.23289683583976384 ) ) ;
#21777=CARTESIAN_POINT ( 'NONE',  ( 20.47266963615838264, 1.058032431983775723, -29.35195464549815014 ) ) ;
#21782=CARTESIAN_POINT ( 'NONE',  ( -28.93253131167843151, 0.05243184118532782240, -11.59459516453416583 ) ) ;
#21785=CARTESIAN_POINT ( 'NONE',  ( 26.55368438709993129, -0.9046161187539608628, -16.29675340907314407 ) ) ;
#21789=CARTESIAN_POINT ( 'NONE',  ( -24.43781183141654623, 4.343050687655961362, -14.72646766136039176 ) ) ;
#21801=CARTESIAN_POINT ( 'NONE',  ( 15.48853125999101898, -26.74269726803731828, -5.000000000000000000 ) ) ;
#21802=CARTESIAN_POINT ( 'NONE',  ( -19.65651305555018169, 6.423002548754848995, -27.12312071538742231 ) ) ;
#21805=CARTESIAN_POINT ( 'NONE',  ( 18.65140588264522137, -20.59310479824253548, -16.86763276178779591 ) ) ;
#21807=CARTESIAN_POINT ( 'NONE',  ( 10.86259508579260746, 17.64226652144433771, -27.43142463228216599 ) ) ;
#21809=CARTESIAN_POINT ( 'NONE',  ( -14.99023650920256756, 21.79341618737742792, -13.61763280836055934 ) ) ;
#21810=EDGE_CURVE ( 'NONE', #19243, #6388, #24993, .T. ) ;
#21813=CARTESIAN_POINT ( 'NONE',  ( 14.75519950962563698, 25.34459079533402104, -10.65436177232459869 ) ) ;
#21817=CARTESIAN_POINT ( 'NONE',  ( -13.91244456763262249, 24.21709252099823928, -13.48676834890144249 ) ) ;
#21819=CARTESIAN_POINT ( 'NONE',  ( -15.12295902014546733, -26.02312468727843253, -9.231359056296803089 ) ) ;
#21823=CARTESIAN_POINT ( 'NONE',  ( -34.77349899548257639, -15.60207130184392987, -6.280198675005461695 ) ) ;
#21824=CARTESIAN_POINT ( 'NONE',  ( -11.07034157884144854, -24.96936304302928988, -10.24950191894629370 ) ) ;
#21826=CARTESIAN_POINT ( 'NONE',  ( 12.38972167065434782, 16.33584955698245977, -29.37623187657347401 ) ) ;
#21828=CARTESIAN_POINT ( 'NONE',  ( 19.85421419770838014, 5.208915335517238177, -28.81948969002354488 ) ) ;
#21834=CARTESIAN_POINT ( 'NONE',  ( -23.55945276895399232, -0.1373144991472548537, -20.44794942058729603 ) ) ;
#21836=CARTESIAN_POINT ( 'NONE',  ( 26.00273584551220196, 0.08967249519437395233, -16.41428873911882746 ) ) ;
#21840=CARTESIAN_POINT ( 'NONE',  ( -37.62663912510979003, -8.659558992827880886, -5.000000000000002665 ) ) ;
#21845=AXIS2_PLACEMENT_3D ( 'NONE', #28822, #29625, #35321 ) ;
#21846=DIRECTION ( 'NONE',  ( -0.000000000000000000, -0.000000000000000000, 1.000000000000000000 ) ) ;
#21848=CARTESIAN_POINT ( 'NONE',  ( 1.512454924012853974, 21.38568066047234950, -25.58676729699224239 ) ) ;
#21857=CARTESIAN_POINT ( 'NONE',  ( 12.69411822000453327, 23.12755374673593423, -16.33488331723920339 ) ) ;
#21860=CARTESIAN_POINT ( 'NONE',  ( -18.70298414372253148, 17.62570364501429410, -6.443206386152125376 ) ) ;
#21863=CARTESIAN_POINT ( 'NONE',  ( 15.17726020569047130, -26.28321538289182513, -8.297710205149746443 ) ) ;
#21864=CARTESIAN_POINT ( 'NONE',  ( -14.51034690954441153, -19.54383024884274533, -20.13759940615653221 ) ) ;
#21865=CARTESIAN_POINT ( 'NONE',  ( 10.98647152928294979, 17.30743895948372568, -30.00000000000000711 ) ) ;
#21866=CARTESIAN_POINT ( 'NONE',  ( 11.05510453204928289, 17.51453838611892522, -27.44640421723807222 ) ) ;
#21869=CARTESIAN_POINT ( 'NONE',  ( -12.58328644382519990, -22.55677566891993280, -16.44928081634269645 ) ) ;
#21871=CARTESIAN_POINT ( 'NONE',  ( -23.88592270937412110, -16.48473916716029919, -16.63925841098920699 ) ) ;
#21872=CARTESIAN_POINT ( 'NONE',  ( -0.3897205959626180993, -24.77793770357540737, -5.482964004482600906 ) ) ;
#21873=CARTESIAN_POINT ( 'NONE',  ( 15.56814849921199695, 26.15651636719908879, -5.946228235075683877 ) ) ;
#21874=CARTESIAN_POINT ( 'NONE',  ( 21.01520796838052618, 9.533611945060952664, -15.93287469514982924 ) ) ;
#21877=CARTESIAN_POINT ( 'NONE',  ( -20.82306015624319073, -2.481982540487905897, -26.57961284343121733 ) ) ;
#21887=CARTESIAN_POINT ( 'NONE',  ( -29.86441318786370047, 0.6479988441763335771, -7.832743955948457071 ) ) ;
#21888=CARTESIAN_POINT ( 'NONE',  ( 33.65435358744935712, -12.34966631407584003, -9.758582659885652433 ) ) ;
#21898=CARTESIAN_POINT ( 'NONE',  ( -3.054091535875387731, 37.95567441806279163, -6.700395517222553998 ) ) ;
#21904=CARTESIAN_POINT ( 'NONE',  ( 13.55441085756498154, 30.31521231272209604, -7.712462757402486879 ) ) ;
#21907=CARTESIAN_POINT ( 'NONE',  ( -20.65769276629826479, 11.18138066491571614, -13.90382682998711417 ) ) ;
#21910=CARTESIAN_POINT ( 'NONE',  ( 15.51551714807790994, -26.62543040642743364, -6.885114030514080774 ) ) ;
#21912=CARTESIAN_POINT ( 'NONE',  ( 15.34541588040626792, 26.76641394790292239, -6.415693964850016862 ) ) ;
#21914=CARTESIAN_POINT ( 'NONE',  ( 26.31271763591406909, -28.25584584496056451, -14.26382729546506667 ) ) ;
#21917=CARTESIAN_POINT ( 'NONE',  ( -14.82594730225876312, 25.65344611243898498, -10.17754751450732265 ) ) ;
#21918=CARTESIAN_POINT ( 'NONE',  ( -26.03722647915365584, -25.89241862741840094, -5.000000000000004441 ) ) ;
#21919=CARTESIAN_POINT ( 'NONE',  ( 8.275334808801511954, -21.38839901459642334, -19.81352468994020910 ) ) ;
#21920=CARTESIAN_POINT ( 'NONE',  ( 14.33783055764683745, 24.35298217862673198, -12.55492370899574972 ) ) ;
#21921=CARTESIAN_POINT ( 'NONE',  ( 24.02681206829297977, -16.26566910256974552, -16.63819982037562184 ) ) ;
#21924=CARTESIAN_POINT ( 'NONE',  ( -10.27371142776379820, 34.65346829918823346, -6.313534688996303323 ) ) ;
#21929=CARTESIAN_POINT ( 'NONE',  ( 30.75739384342617555, 0.004716038886164508614, -6.417043594193787115 ) ) ;
#21934=CARTESIAN_POINT ( 'NONE',  ( -20.52549850993021607, 0.8876484853251380702, -28.70801360605462094 ) ) ;
#21938=CARTESIAN_POINT ( 'NONE',  ( 20.21125490546006276, -3.489748019849370220, -29.99999999999998579 ) ) ;
#21942=EDGE_LOOP ( 'NONE', ( #18254, #23102, #5216, #729, #33359, #32733, #31482, #7829 ) ) ;
#21953=CARTESIAN_POINT ( 'NONE',  ( -19.08133911595188437, 7.519478901772812307, -29.99999999999999645 ) ) ;
#21956=CARTESIAN_POINT ( 'NONE',  ( 18.04900360418865546, 18.86275876442724453, -7.401912832897363792 ) ) ;
#21957=CARTESIAN_POINT ( 'NONE',  ( 9.059065324806985231, 35.31177540401563419, -7.163937956742758573 ) ) ;
#21959=EDGE_CURVE ( 'NONE', #16687, #31932, #7558, .T. ) ;
#21960=CARTESIAN_POINT ( 'NONE',  ( 17.41134420666527660, -26.92035120749303445, -7.305176101613050754 ) ) ;
#21961=DIRECTION ( 'NONE',  ( 0.000000000000000000, 0.000000000000000000, 1.000000000000000000 ) ) ;
#21963=B_SPLINE_CURVE_WITH_KNOTS ( 'NONE', 3,
 ( #37643, #21998, #12454, #3511 ),
 .UNSPECIFIED., .F., .F.,
 ( 4, 4 ),
 ( 0.000000000000000000, 0.1234515740337736034 ),
 .UNSPECIFIED. ) ;
#21965=ORIENTED_EDGE ( 'NONE', *, *, #24369, .F. ) ;
#21966=CARTESIAN_POINT ( 'NONE',  ( -11.23742582611742513, 17.39156283123631752, -27.46051757209724897 ) ) ;
#21969=CARTESIAN_POINT ( 'NONE',  ( 11.80044851807104678, -21.49314593586473876, -18.46258872189030242 ) ) ;
#21973=CARTESIAN_POINT ( 'NONE',  ( -13.92122689940795510, 28.37753238768550190, -9.577933452506133705 ) ) ;
#21974=CARTESIAN_POINT ( 'NONE',  ( -11.08653240243507554, -17.32279251903801409, -28.64327423991444377 ) ) ;
#21977=CARTESIAN_POINT ( 'NONE',  ( -26.20239787803879850, -7.299429199793270762, -17.76499887194331961 ) ) ;
#21978=CARTESIAN_POINT ( 'NONE',  ( -9.394881763177457046, -18.22048488343288142, -29.35045134641008957 ) ) ;
#21981=CARTESIAN_POINT ( 'NONE',  ( 20.67958368883273224, 1.036419229453801050, -27.46041608859013650 ) ) ;
#21985=CARTESIAN_POINT ( 'NONE',  ( -20.52899626704462932, 0.8142514703770860063, -28.70543900254816805 ) ) ;
#21986=EDGE_CURVE ( 'NONE', #29585, #35629, #17551, .T. ) ;
#21988=CARTESIAN_POINT ( 'NONE',  ( 20.88948691698688265, -0.6490584520769514532, -26.71535767925633564 ) ) ;
#21989=CARTESIAN_POINT ( 'NONE',  ( 15.27779781845867468, -13.73655938454271030, -29.99999999999999645 ) ) ;
#21992=CARTESIAN_POINT ( 'NONE',  ( -26.64229111171870912, 4.405581445021985232, -7.868447511081861911 ) ) ;
#21993=EDGE_CURVE ( 'NONE', #12248, #19728, #2106, .T. ) ;
#21998=CARTESIAN_POINT ( 'NONE',  ( -17.14571668001621418, -27.17024302301528849, -4.999999999999999112 ) ) ;
#22001=PRODUCT_DEFINITION_SHAPE ( 'NONE', 'NONE',  #27397 ) ;
#22004=CARTESIAN_POINT ( 'NONE',  ( -19.80772954507643391, 5.710854581715417488, -27.67139024716352225 ) ) ;
#22007=CARTESIAN_POINT ( 'NONE',  ( 19.29622809070872691, -21.30767804701306289, -15.90023521376778604 ) ) ;
#22010=CARTESIAN_POINT ( 'NONE',  ( 15.27493397812733988, 27.00603829493833175, -6.411867504281748786 ) ) ;
#22012=CARTESIAN_POINT ( 'NONE',  ( -12.27438659830399104, 16.41897796854597047, -30.00000000000000000 ) ) ;
#22015=CARTESIAN_POINT ( 'NONE',  ( 11.72000814234884025, 18.87896920474838680, -22.74070836927191053 ) ) ;
#22017=CARTESIAN_POINT ( 'NONE',  ( -14.23945615837876311, -31.58416516429889853, 0.000000000000000000 ) ) ;
#22019=CARTESIAN_POINT ( 'NONE',  ( -14.17779301840820239, 24.76684511783872011, -12.52556781375514738 ) ) ;
#22021=CARTESIAN_POINT ( 'NONE',  ( -15.29280108727264853, -26.19529837291199215, -8.758642717996806937 ) ) ;
#22025=CARTESIAN_POINT ( 'NONE',  ( -33.98065044953765579, -15.22623518443444901, -8.413853775630943943 ) ) ;
#22026=CARTESIAN_POINT ( 'NONE',  ( -13.97107818215439146, -25.64569743057662166, -9.722743490932185040 ) ) ;
#22028=CARTESIAN_POINT ( 'NONE',  ( 16.38359496941714966, 23.11600525820518115, -7.374208509789634824 ) ) ;
#22030=CARTESIAN_POINT ( 'NONE',  ( 25.86526715380574259, 4.645913844102615542, -10.29163244528595200 ) ) ;
#22036=CARTESIAN_POINT ( 'NONE',  ( -30.84242166733599788, -0.3958891573209706860, -7.811368989421731079 ) ) ;
#22038=CARTESIAN_POINT ( 'NONE',  ( 20.61837044269047681, 0.7085719058875546983, -28.07041881223954860 ) ) ;
#22042=CARTESIAN_POINT ( 'NONE',  ( 12.33616729053617966, -27.99489201236593416, -5.000000000000000000 ) ) ;
#22049=CARTESIAN_POINT ( 'NONE',  ( 3.810525450730533947, 37.24451434163790253, -7.981115972861925201 ) ) ;
#22059=CARTESIAN_POINT ( 'NONE',  ( 15.00330998323748055, 28.06465100738194351, -4.999999999999998224 ) ) ;
#22062=CARTESIAN_POINT ( 'NONE',  ( -18.09385140116044965, 18.44421545049425504, -8.373696076410258371 ) ) ;
#22065=CARTESIAN_POINT ( 'NONE',  ( 9.486164890912217373, -18.17313361576023212, -29.34858962865161303 ) ) ;
#22066=CARTESIAN_POINT ( 'NONE',  ( -20.92342021452639855, -26.27463686021861378, -9.014949617875791077 ) ) ;
#22067=CARTESIAN_POINT ( 'NONE',  ( 15.17557291600564362, 26.27770503188184037, -8.298014751482952533 ) ) ;
#22068=CARTESIAN_POINT ( 'NONE',  ( 12.38369262076488475, 20.50029293666852226, -19.49479296581450427 ) ) ;
#22071=CARTESIAN_POINT ( 'NONE',  ( -9.648264831776160122, -18.46096267954140657, -26.83400085027493986 ) ) ;
#22074=CARTESIAN_POINT ( 'NONE',  ( -19.84140702193834827, -14.57578147485350506, -20.72667381623678651 ) ) ;
#22075=CARTESIAN_POINT ( 'NONE',  ( -2.250492809306957387, -22.96836341133687753, -15.94180792882460018 ) ) ;
#22076=CARTESIAN_POINT ( 'NONE',  ( 14.19245098026133967, 22.50397599124407932, -14.52977076431803560 ) ) ;
#22078=CARTESIAN_POINT ( 'NONE',  ( 18.70205627895097678, 9.558498540185201620, -24.40894002729765688 ) ) ;
#22083=CARTESIAN_POINT ( 'NONE',  ( -22.73893131577041871, -2.785302627231514006, -22.32846206850632598 ) ) ;
#22091=CARTESIAN_POINT ( 'NONE',  ( -21.60728915618764390, 1.248469937430795262, -23.91367510233994764 ) ) ;
#22092=CARTESIAN_POINT ( 'NONE',  ( 19.81193986357125425, -7.322314881371388751, -26.31558243123959073 ) ) ;
#22101=CARTESIAN_POINT ( 'NONE',  ( -3.032905758677766794, 37.61468665050777105, -7.549769678190211941 ) ) ;
#22108=CARTESIAN_POINT ( 'NONE',  ( 8.094548601407081989, 18.84590462288236878, -29.28895203708815487 ) ) ;
#22110=CARTESIAN_POINT ( 'NONE',  ( -20.71964873649640282, 12.39161998634679840, -10.88618712900710150 ) ) ;
#22112=CARTESIAN_POINT ( 'NONE',  ( 11.22784262000083899, -20.46096934038583015, -20.53583499620931363 ) ) ;
#22116=CARTESIAN_POINT ( 'NONE',  ( 14.70889546940418136, 25.48292030289299959, -10.64750965446335762 ) ) ;
#22117=CARTESIAN_POINT ( 'NONE',  ( 8.937590682902566641, -20.71651963383554218, -21.24786896499729494 ) ) ;
#22118=DIRECTION ( 'NONE',  ( -0.000000000000000000, -0.000000000000000000, -1.000000000000000000 ) ) ;
#22119=CARTESIAN_POINT ( 'NONE',  ( -26.93779216284742972, -25.25507388614077797, -6.299698065591226026 ) ) ;
#22120=CARTESIAN_POINT ( 'NONE',  ( 8.427633117194249124, -18.99098521131534412, -26.92671562467327107 ) ) ;
#22121=CARTESIAN_POINT ( 'NONE',  ( 11.09252425524408459, 17.23965631597926418, -29.99999999999999289 ) ) ;
#22122=CARTESIAN_POINT ( 'NONE',  ( 17.32296204507781212, -11.70303779259323917, -26.97532818047861269 ) ) ;
#22126=CARTESIAN_POINT ( 'NONE',  ( -8.013417946183661655, 33.96338083945676800, -10.23839836295345229 ) ) ;
#22131=CARTESIAN_POINT ( 'NONE',  ( 30.47427288445410554, -0.0007432638058615850113, -7.827850035976748444 ) ) ;
#22136=CARTESIAN_POINT ( 'NONE',  ( -20.81434011470259193, 0.8451126377779130117, -26.83172302409398924 ) ) ;
#22139=CARTESIAN_POINT ( 'NONE',  ( 34.03611443232053091, -6.103416065348592490, -8.094509381288824912 ) ) ;
#22148=CARTESIAN_POINT ( 'NONE',  ( 1.419287350250943325, 20.45362594422159219, -30.00000000000000711 ) ) ;
#22151=CARTESIAN_POINT ( 'NONE',  ( 16.28467717620302579, 16.38496874790540758, -17.87567372210706296 ) ) ;
#22152=CARTESIAN_POINT ( 'NONE',  ( 5.103355680224397339, 19.86390335519187289, -29.24334217793310842 ) ) ;
#22156=CARTESIAN_POINT ( 'NONE',  ( 14.72827463056593444, -23.14637955489208565, -15.28270852680887693 ) ) ;
#22160=CARTESIAN_POINT ( 'NONE',  ( -14.54212453546162465, 24.94396834142040120, -11.59977209224463479 ) ) ;
#22162=CARTESIAN_POINT ( 'NONE',  ( 9.346475367005044887, -18.24555389153483631, -30.00000000000000000 ) ) ;
#22169=CARTESIAN_POINT ( 'NONE',  ( -14.36450198187400318, 29.42115241676423310, -6.376794364350948818 ) ) ;
#22172=CARTESIAN_POINT ( 'NONE',  ( -33.71982540184990995, -9.379966980860906745, -9.801996931721211226 ) ) ;
#22173=CARTESIAN_POINT ( 'NONE',  ( -15.12720010012756156, -26.36448638230414687, -7.828442106200601991 ) ) ;
#22176=CARTESIAN_POINT ( 'NONE',  ( 25.72413230257677341, 0.5541670876175327498, -16.46445719556119514 ) ) ;
#22180=CARTESIAN_POINT ( 'NONE',  ( -30.92750986253986767, -0.06599190286722655951, -5.000000000000000000 ) ) ;
#22182=CARTESIAN_POINT ( 'NONE',  ( 32.75437695154221274, -2.309567439508531272, -5.462365998068315243 ) ) ;
#22183=CARTESIAN_POINT ( 'NONE',  ( -7.326526595265096198, -19.15832871326084330, -30.00000000000001066 ) ) ;
#22195=CARTESIAN_POINT ( 'NONE',  ( -22.97007816870513608, 9.885904127924739271, -5.482133400955172320 ) ) ;
#22196=CARTESIAN_POINT ( 'NONE',  ( 22.46963405367063160, -26.15767612554902399, -8.532870437220990922 ) ) ;
#22199=CARTESIAN_POINT ( 'NONE',  ( 12.82845314113447444, 21.81843741845949580, -17.41504233143949776 ) ) ;
#22201=CARTESIAN_POINT ( 'NONE',  ( -13.77473007477936306, 20.30411881401572316, -17.57123835615476892 ) ) ;
#22205=CARTESIAN_POINT ( 'NONE',  ( 15.19494511612774090, 26.21339590839900069, -8.298239470938288065 ) ) ;
#22209=CARTESIAN_POINT ( 'NONE',  ( -10.88757786208257805, 17.52439729938563318, -28.06831848310639899 ) ) ;
#22211=CARTESIAN_POINT ( 'NONE',  ( -9.580852559982135475, -18.12344168749379492, -30.00000000000000000 ) ) ;
#22214=CARTESIAN_POINT ( 'NONE',  ( -22.78420442030176929, -11.94118074355967352, -19.63367908279295548 ) ) ;
#22215=CARTESIAN_POINT ( 'NONE',  ( -12.34945208490760216, -23.53982313883594202, -14.53211625936720885 ) ) ;
#22217=CARTESIAN_POINT ( 'NONE',  ( 14.60279944388903495, 20.71121289329725457, -15.60062821346018325 ) ) ;
#22219=CARTESIAN_POINT ( 'NONE',  ( 21.81847007083357326, 4.523505414233293109, -20.94089222306983089 ) ) ;
#22225=CARTESIAN_POINT ( 'NONE',  ( -20.84162644709726209, 0.4883270344463671031, -26.80397353251239423 ) ) ;
#22226=CARTESIAN_POINT ( 'NONE',  ( 31.20266475843156329, -0.3930892854634324141, -5.941229959064580513 ) ) ;
#22231=CARTESIAN_POINT ( 'NONE',  ( -31.47283671532259675, -25.12609584734821411, -5.000000000000010658 ) ) ;
#22239=CARTESIAN_POINT ( 'NONE',  ( 2.971324280269732387, 22.57991813769753264, -23.03519204931057374 ) ) ;
#22247=CARTESIAN_POINT ( 'NONE',  ( 10.56422568374752480, 17.99037428788165371, -26.77787062081501190 ) ) ;
#22251=CARTESIAN_POINT ( 'NONE',  ( -18.26045280058711739, 18.67344520970426913, -5.958434712537178157 ) ) ;
#22252=CARTESIAN_POINT ( 'NONE',  ( 14.98890121934609532, -28.67928442654221044, -5.000000000000000000 ) ) ;
#22255=CARTESIAN_POINT ( 'NONE',  ( 15.45091137245021429, -26.73300375246232008, -5.000000000000000000 ) ) ;
#22257=CARTESIAN_POINT ( 'NONE',  ( 14.29112916160344859, 24.47062756151937180, -12.55066837350503839 ) ) ;
#22259=CARTESIAN_POINT ( 'NONE',  ( 15.28428319961222570, 26.55126983923268114, -7.357174194785967458 ) ) ;
#22262=CARTESIAN_POINT ( 'NONE',  ( -15.39818770356525945, -26.71945962344603487, -5.000000000000000888 ) ) ;
#22265=CARTESIAN_POINT ( 'NONE',  ( -25.96013749710196450, -19.13211056138908361, -13.82494223876936346 ) ) ;
#22266=CARTESIAN_POINT ( 'NONE',  ( -1.948798780195311275, -21.39903356808110146, -22.24353699554251662 ) ) ;
#22267=CARTESIAN_POINT ( 'NONE',  ( 12.51562164745455874, 19.46842532610077825, -20.60745837019819859 ) ) ;
#22269=CARTESIAN_POINT ( 'NONE',  ( 23.39763224849028234, 9.229310415396369649, -4.999999999999999112 ) ) ;
#22274=CARTESIAN_POINT ( 'NONE',  ( -33.86638135467044464, -4.484472903435158919, -6.349560011803310644 ) ) ;
#22282=CARTESIAN_POINT ( 'NONE',  ( -24.79870091042203484, 1.154735779887344771, -17.51345790379463807 ) ) ;
#22284=CARTESIAN_POINT ( 'NONE',  ( 19.60579457783088841, -8.618293326532800336, -25.60564762322205823 ) ) ;
#22290=LINE ( 'NONE', #13145, #261 ) ;
#22295=CARTESIAN_POINT ( 'NONE',  ( -0.4054287150579977683, 20.91504830566051254, -26.96527958665584634 ) ) ;
#22296=FACE_OUTER_BOUND ( 'NONE', #4050, .T. ) ;
#22303=CARTESIAN_POINT ( 'NONE',  ( 11.02804646868720617, 24.24809588149700090, -17.10494504817883055 ) ) ;
#22306=CARTESIAN_POINT ( 'NONE',  ( -20.55655765742755747, 12.29105890200828455, -11.88403847902282529 ) ) ;
#22310=CARTESIAN_POINT ( 'NONE',  ( 12.70345522867710741, -22.55901976966053368, -16.43839307279606032 ) ) ;
#22312=CARTESIAN_POINT ( 'NONE',  ( 10.93327523444657778, 17.34109439532409525, -29.34725070414031478 ) ) ;
#22313=CARTESIAN_POINT ( 'NONE',  ( 7.289639608743135213, -27.06962010326278190, -5.000000000000004441 ) ) ;
#22316=CARTESIAN_POINT ( 'NONE',  ( -17.85134198839684316, -18.89656077001060552, -18.85215370857916639 ) ) ;
#22317=CARTESIAN_POINT ( 'NONE',  ( 6.120099083145483121, -24.74703752395057421, -8.867573918171460789 ) ) ;
#22318=CARTESIAN_POINT ( 'NONE',  ( 14.60292836218529544, 24.77861828538451050, -11.60468508207308069 ) ) ;
#22319=CARTESIAN_POINT ( 'NONE',  ( 17.38935910474636160, -12.52520610644180366, -25.59909104371132216 ) ) ;
#22323=CARTESIAN_POINT ( 'NONE',  ( -8.044889785369548463, 30.10955582739369163, -13.93146741096502872 ) ) ;
#22326=CARTESIAN_POINT ( 'NONE',  ( 25.87031140294526921, 0.3067695561049477715, -16.44274321582222953 ) ) ;
#22330=CARTESIAN_POINT ( 'NONE',  ( -27.11474883183905504, 0.2720220986060000734, -14.47902593302377738 ) ) ;
#22333=CARTESIAN_POINT ( 'NONE',  ( 20.16346151983087509, -4.126571039269510521, -28.54077426291244990 ) ) ;
#22344=CARTESIAN_POINT ( 'NONE',  ( -18.10143317280823894, -9.644849403491171813, -30.00000000000001421 ) ) ;
#22347=CARTESIAN_POINT ( 'NONE',  ( 17.84657098941836040, 18.57841126220657557, -9.344939892030197370 ) ) ;
#22348=CARTESIAN_POINT ( 'NONE',  ( 5.797474147347187134, 25.70591046706581295, -18.75075227247661758 ) ) ;
#22350=CARTESIAN_POINT ( 'NONE',  ( 16.16426081259751513, -26.77215978000938890, -6.871636933944165193 ) ) ;
#22355=CARTESIAN_POINT ( 'NONE',  ( -15.39831948222068192, 26.75390157443277772, -5.946046044839542688 ) ) ;
#22357=CARTESIAN_POINT ( 'NONE',  ( 12.19254079021881587, -22.55338299999295870, -16.47865374781240888 ) ) ;
#22361=CARTESIAN_POINT ( 'NONE',  ( -8.916636640703819339, 18.64685610723298836, -27.95511672575932494 ) ) ;
#22363=CARTESIAN_POINT ( 'NONE',  ( -12.11431924477676425, -16.53859993892360336, -30.00000000000000711 ) ) ;
#22366=CIRCLE ( 'NONE', #15910, 18.00000000000000355 ) ;
#22367=CARTESIAN_POINT ( 'NONE',  ( -24.28665842282865839, -6.776736144980733734, -19.81828135623066345 ) ) ;
#22370=CARTESIAN_POINT ( 'NONE',  ( 29.18931739517128676, 0.2643966938976765602, -10.65876322853514502 ) ) ;
#22374=CARTESIAN_POINT ( 'NONE',  ( -25.87499874312591785, 0.2997861449386328148, -16.44121720947547871 ) ) ;
#22376=CARTESIAN_POINT ( 'NONE',  ( 29.56918532523465259, -1.550794330668424648, -12.39820313618830205 ) ) ;
#22394=CARTESIAN_POINT ( 'NONE',  ( -22.85284608940409257, 9.847895807180515604, -7.423717738255721343 ) ) ;
#22395=CARTESIAN_POINT ( 'NONE',  ( 13.47898897988460121, -15.87835076097369580, -27.16664839183066249 ) ) ;
#22397=CARTESIAN_POINT ( 'NONE',  ( 11.38208074324289854, 18.52518290154176483, -23.83773640263114046 ) ) ;
#22399=CARTESIAN_POINT ( 'NONE',  ( -15.38402806139854384, 25.23968687678138068, -8.776766146092349175 ) ) ;
#22403=CARTESIAN_POINT ( 'NONE',  ( 13.51484764804600935, 22.76996113590243453, -15.45381432112062825 ) ) ;
#22405=CARTESIAN_POINT ( 'NONE',  ( 33.70372332681250782, -18.58847439657466083, -5.435464265174550391 ) ) ;
#22408=CARTESIAN_POINT ( 'NONE',  ( -11.92048302216191047, 20.17252841636972960, -20.49873944758164868 ) ) ;
#22410=CARTESIAN_POINT ( 'NONE',  ( -9.994354138142316657, -18.05759666164655286, -28.05362611333584866 ) ) ;
#22413=CARTESIAN_POINT ( 'NONE',  ( -18.43967439804336550, -8.978407292334221523, -30.00000000000000711 ) ) ;
#22414=CARTESIAN_POINT ( 'NONE',  ( -9.792301971375101388, -19.78694043973939287, -22.82254168301635033 ) ) ;
#22416=CARTESIAN_POINT ( 'NONE',  ( 15.52145767144611099, 22.42669402248078470, -11.67624505304624094 ) ) ;
#22418=CARTESIAN_POINT ( 'NONE',  ( 25.41189056253793410, 4.628821310671148659, -11.75822289690720268 ) ) ;
#22420=CARTESIAN_POINT ( 'NONE',  ( 3.485571585149872753, -11.24999999999998224, 6.000000000000000000 ) ) ;
#22423=CARTESIAN_POINT ( 'NONE',  ( -28.02036111935687757, -0.1831946594191615485, -13.47373158784090563 ) ) ;
#22424=CARTESIAN_POINT ( 'NONE',  ( 23.40003965484141446, 0.3230641209998412200, -20.51045967696057559 ) ) ;
#22431=CARTESIAN_POINT ( 'NONE',  ( -21.88499642459564853, -5.528038495964381127, -30.00000000000000355 ) ) ;
#22437=CARTESIAN_POINT ( 'NONE',  ( 15.41558956984165363, 26.78481017248027740, -5.000000000000000000 ) ) ;
#22438=CARTESIAN_POINT ( 'NONE',  ( 3.093609891035674853, 23.47637780903313853, -21.88905062759406306 ) ) ;
#22443=CARTESIAN_POINT ( 'NONE',  ( 28.46220377038417126, -23.29623700624878779, -8.431205218395554368 ) ) ;
#22447=DIRECTION ( 'NONE',  ( -0.000000000000000000, -0.000000000000000000, 1.000000000000000000 ) ) ;
#22448=CARTESIAN_POINT ( 'NONE',  ( 10.76979477178801936, 18.04852582976164044, -26.18016545178095100 ) ) ;
#22451=CARTESIAN_POINT ( 'NONE',  ( -17.59337500131034915, 19.37719024453491201, -8.848041657323321374 ) ) ;
#22457=CARTESIAN_POINT ( 'NONE',  ( 11.87964959439185897, -21.48688383848312000, -18.45485520218330677 ) ) ;
#22460=CARTESIAN_POINT ( 'NONE',  ( 10.98647152928295156, 17.30743895948372568, -29.34839841643596614 ) ) ;
#22461=ORIENTED_EDGE ( 'NONE', *, *, #32237, .F. ) ;
#22462=CARTESIAN_POINT ( 'NONE',  ( 11.00058940542414554, 17.35166013633943649, -28.70672724212847271 ) ) ;
#22465=CARTESIAN_POINT ( 'NONE',  ( -11.17406680738855584, -20.47027838762622665, -20.54295404136550118 ) ) ;
#22467=CARTESIAN_POINT ( 'NONE',  ( -29.65485267539152048, -20.48675704930219155, -10.17941642897329224 ) ) ;
#22468=CARTESIAN_POINT ( 'NONE',  ( -3.392224512981891316, -20.63403223353535410, -25.47406074567986778 ) ) ;
#22469=CARTESIAN_POINT ( 'NONE',  ( 15.65441761974471113, 25.86232774665390366, -5.946368842702213442 ) ) ;
#22471=CARTESIAN_POINT ( 'NONE',  ( 22.11137694095066308, 11.05602416922195630, -7.426733222396916467 ) ) ;
#22475=CARTESIAN_POINT ( 'NONE',  ( -32.89022462939520608, -4.305485280278338323, -9.038522573761735401 ) ) ;
#22477=ORIENTED_EDGE ( 'NONE', *, *, #35131, .T. ) ;
#22481=CARTESIAN_POINT ( 'NONE',  ( 20.12997315792683395, -8.847206737175625335, -24.25336459654654320 ) ) ;
#22488=CARTESIAN_POINT ( 'NONE',  ( -15.45712587483427924, 26.63597398780867564, -5.000000000000002665 ) ) ;
#22491=CARTESIAN_POINT ( 'NONE',  ( -0.7539017812582486933, 38.52547057370831141, -5.435359319770989295 ) ) ;
#22497=CARTESIAN_POINT ( 'NONE',  ( 13.78612880735749791, 27.70518701290404451, -10.51413500146422564 ) ) ;
#22498=DIRECTION ( 'NONE',  ( -0.000000000000000000, -0.000000000000000000, -1.000000000000000000 ) ) ;
#22500=CARTESIAN_POINT ( 'NONE',  ( -18.80902559120175255, 10.24077132063193041, -22.24714609963263001 ) ) ;
#22503=CARTESIAN_POINT ( 'NONE',  ( 15.47542781151556213, -26.66463022141588368, -6.416210468062471861 ) ) ;
#22505=CARTESIAN_POINT ( 'NONE',  ( 15.20930106813657368, 26.48505469187728423, -7.825161417022220789 ) ) ;
#22506=CARTESIAN_POINT ( 'NONE',  ( -18.07620401364299667, 24.68088026512193167, -13.58461195433497082 ) ) ;
#22510=CARTESIAN_POINT ( 'NONE',  ( -14.62643312820280528, -15.49996111506702512, -25.77096336785993103 ) ) ;
#22511=CARTESIAN_POINT ( 'NONE',  ( 5.856590299683157141, -20.17846598857110507, -25.37062753232054746 ) ) ;
#22512=CARTESIAN_POINT ( 'NONE',  ( 15.10734495844927849, 25.68721481206937085, -9.241857395831049260 ) ) ;
#22513=CARTESIAN_POINT ( 'NONE',  ( 23.08576052398056078, -15.62326469692720110, -17.60933158146236366 ) ) ;
#22517=CARTESIAN_POINT ( 'NONE',  ( -6.983932559990830846, 26.21054456205356331, -17.77984188425750389 ) ) ;
#22521=CARTESIAN_POINT ( 'NONE',  ( 30.22229184125601265, -0.02826660990534823545, -8.765447815367933160 ) ) ;
#22525=CARTESIAN_POINT ( 'NONE',  ( -26.41186682634353389, 0.4197715753672409678, -15.46164128583599329 ) ) ;
#22529=CARTESIAN_POINT ( 'NONE',  ( 33.51572963880570910, -7.992457164366485678, -9.832202616107817761 ) ) ;
#22542=SURFACE_SIDE_STYLE ('',( #20116 ) ) ;
#22547=CARTESIAN_POINT ( 'NONE',  ( 17.71135169000040932, 20.05059954136391553, -5.477262195481070073 ) ) ;
#22549=CARTESIAN_POINT ( 'NONE',  ( 11.56236212135367047, 32.93568925309087803, -7.647066273184269569 ) ) ;
#22551=CARTESIAN_POINT ( 'NONE',  ( 10.21873439408511253, -18.03641402610821842, -27.40419155213225721 ) ) ;
#22553=B_SPLINE_CURVE_WITH_KNOTS ( 'NONE', 3,
 ( #36166, #38808, #23372, #10984, #7922, #29663, #39006, #20736, #11182 ),
 .UNSPECIFIED., .F., .F.,
 ( 4, 1, 1, 1, 1, 1, 4 ),
 ( 0.3034822677883343145, 0.3750000000143087764, 0.4999999999999940048, 0.6249999999856795663, 0.7499999999713649057, 0.8749999999570503562, 1.000000000000000000 ),
 .UNSPECIFIED. ) ;
#22558=CARTESIAN_POINT ( 'NONE',  ( -15.02206552268004458, 25.95591568151323969, -9.238934606167955366 ) ) ;
#22560=CARTESIAN_POINT ( 'NONE',  ( 9.296951271124752836, -18.31947431080797628, -28.71563296508281482 ) ) ;
#22565=CARTESIAN_POINT ( 'NONE',  ( -13.55309326636294109, 29.69719733569533915, -8.626781295736174471 ) ) ;
#22569=AXIS2_PLACEMENT_3D ( 'NONE', #4345, #13279, #19379 ) ;
#22570=CARTESIAN_POINT ( 'NONE',  ( -35.11052852875971553, -8.727991070938342588, -6.744352222248348738 ) ) ;
#22573=CARTESIAN_POINT ( 'NONE',  ( 20.80244950058357034, 0.9809649937616239379, -26.84207219552697410 ) ) ;
#22578=CARTESIAN_POINT ( 'NONE',  ( -29.59593009434644983, 0.04982597378002901617, -10.18041819265831549 ) ) ;
#22582=CARTESIAN_POINT ( 'NONE',  ( 33.36633864933632054, -3.217268494394103673, -5.000000000000000000 ) ) ;
#22597=CARTESIAN_POINT ( 'NONE',  ( -23.58808727774059832, 8.960771098271621327, -5.481298557163171381 ) ) ;
#22598=CARTESIAN_POINT ( 'NONE',  ( 18.77937622075242530, -23.29516096719056861, -14.07484684245071982 ) ) ;
#22602=CARTESIAN_POINT ( 'NONE',  ( 15.32234214663592375, 26.84634284219205824, -6.414409059685876713 ) ) ;
#22605=CARTESIAN_POINT ( 'NONE',  ( -13.03496280190833723, 19.64411286304471815, -19.60530794096396434 ) ) ;
#22608=CARTESIAN_POINT ( 'NONE',  ( 11.92636920872155670, 19.34590550356041305, -21.62300054144612460 ) ) ;
#22610=CARTESIAN_POINT ( 'NONE',  ( 18.81768709236329329, -9.658926806160746281, -26.25942549260763670 ) ) ;
#22614=CARTESIAN_POINT ( 'NONE',  ( -11.24118742064583998, 18.64458347442174713, -23.81550990468068107 ) ) ;
#22616=CARTESIAN_POINT ( 'NONE',  ( -16.68682434244347590, -26.92965747703111390, -6.397897022492878172 ) ) ;
#22619=CARTESIAN_POINT ( 'NONE',  ( -22.46715076204040429, -10.09974697177796088, -20.72078323234527630 ) ) ;
#22620=CARTESIAN_POINT ( 'NONE',  ( -9.971190107407892356, -19.73728639792070538, -22.80224159634297720 ) ) ;
#22622=CARTESIAN_POINT ( 'NONE',  ( 13.88678101316755864, 18.51693486955983659, -19.73415532929779914 ) ) ;
#22624=CARTESIAN_POINT ( 'NONE',  ( 23.90103726830303899, 3.753447309722855785, -16.71722843108891965 ) ) ;
#22628=CARTESIAN_POINT ( 'NONE',  ( -20.73211841591003690, 0.1678577862357426842, -27.40417673715113978 ) ) ;
#22629=CARTESIAN_POINT ( 'NONE',  ( 29.33018326755770744, -0.4255386876862592427, -11.55134619685823516 ) ) ;
#22634=CARTESIAN_POINT ( 'NONE',  ( -13.28992586503615669, -18.25382200079944539, -20.55760979252988463 ) ) ;
#22644=CARTESIAN_POINT ( 'NONE',  ( 15.88542612224667927, -12.95767258840383107, -29.22532221307605838 ) ) ;
#22647=CARTESIAN_POINT ( 'NONE',  ( 13.80587148021421484, 24.46212733322120414, -13.46414252330034778 ) ) ;
#22651=CARTESIAN_POINT ( 'NONE',  ( -14.63038540974646828, 16.30325065141676077, -22.01182681179342637 ) ) ;
#22654=CARTESIAN_POINT ( 'NONE',  ( 15.29084952668607933, -26.49705136638473846, -7.357960102425458615 ) ) ;
#22656=CARTESIAN_POINT ( 'NONE',  ( 11.12160456634172512, 17.61533166272547035, -26.83009323505500987 ) ) ;
#22658=CARTESIAN_POINT ( 'NONE',  ( 13.76332498804387861, 23.40953749546633134, -14.47517996330730305 ) ) ;
#22662=CARTESIAN_POINT ( 'NONE',  ( -12.08249424194362120, 19.98192381863790956, -20.53110637240889602 ) ) ;
#22664=CARTESIAN_POINT ( 'NONE',  ( -9.594949128275974459, -18.35353841803804542, -27.44967104049570850 ) ) ;
#22666=CARTESIAN_POINT ( 'NONE',  ( -18.49734238951277732, -11.93560065676270021, -24.22553531776692992 ) ) ;
#22667=CARTESIAN_POINT ( 'NONE',  ( -3.697151520580219231, -21.53368035006806380, -21.12883000117165366 ) ) ;
#22668=CARTESIAN_POINT ( 'NONE',  ( 15.49389368908896714, 25.54012532978367389, -7.832773519083336744 ) ) ;
#22671=CARTESIAN_POINT ( 'NONE',  ( 18.94224516238102396, 8.015443379958615111, -28.28845633141069627 ) ) ;
#22673=CARTESIAN_POINT ( 'NONE',  ( -15.46713722816187975, -26.73718067935205056, -5.000000000000000000 ) ) ;
#22677=CARTESIAN_POINT ( 'NONE',  ( -23.36115073782027096, -2.173507815852580016, -21.26580309426782733 ) ) ;
#22679=ORIENTED_EDGE ( 'NONE', *, *, #24599, .F. ) ;
#22682=CARTESIAN_POINT ( 'NONE',  ( 34.43848434938189484, -16.34293750617152696, -6.699837301618770447 ) ) ;
#22691=CARTESIAN_POINT ( 'NONE',  ( -28.92287456554050351, 1.976372635573284242, -5.000000000000000000 ) ) ;
#22692=DIRECTION ( 'NONE',  ( -1.000000000000000000, 0.000000000000000000, 0.000000000000000000 ) ) ;
#22694=CARTESIAN_POINT ( 'NONE',  ( -0.4022046384660851182, 20.75372784789253799, -27.70456478907405184 ) ) ;
#22700=CARTESIAN_POINT ( 'NONE',  ( 14.46705284293606120, 29.28167841381910463, -5.921992419550550224 ) ) ;
#22703=CARTESIAN_POINT ( 'NONE',  ( -16.81891822627442323, 11.75299315897373731, -28.85843616979807535 ) ) ;
#22706=CARTESIAN_POINT ( 'NONE',  ( 15.22463038672936086, -26.29468693911994848, -8.295888942704511493 ) ) ;
#22708=CARTESIAN_POINT ( 'NONE',  ( 11.00364732032666382, 17.44887877622111461, -28.07524110270195195 ) ) ;
#22709=CARTESIAN_POINT ( 'NONE',  ( -21.88444403592365362, 6.126538576424530369, -21.50719306941233455 ) ) ;
#22711=CYLINDRICAL_SURFACE ( 'NONE', #33675, 16.00000000000000711 ) ;
#22712=CARTESIAN_POINT ( 'NONE',  ( -15.98951276118712883, -15.93656576511519951, -23.18934444843043607 ) ) ;
#22713=CARTESIAN_POINT ( 'NONE',  ( 5.693958622330683284, -19.87604177814888473, -27.65608055801159892 ) ) ;
#22714=CARTESIAN_POINT ( 'NONE',  ( 15.31836689275630370, 26.11603314008040400, -7.829368276863946541 ) ) ;
#22715=CARTESIAN_POINT ( 'NONE',  ( 18.88587872898141740, 12.68145420873708851, -16.97363421066873812 ) ) ;
#22717=DIRECTION ( 'NONE',  ( 1.000000000000000000, 0.000000000000000000, 0.000000000000000000 ) ) ;
#22720=CARTESIAN_POINT ( 'NONE',  ( -9.379895652603979173, 35.46246444712465973, -5.000000000000002665 ) ) ;
#22724=CARTESIAN_POINT ( 'NONE',  ( 20.81719713451408893, 0.8112600457793633923, -26.82911930713009241 ) ) ;
#22726=DIRECTION ( 'NONE',  ( 1.000000000000000000, 0.000000000000000000, 0.000000000000000000 ) ) ;
#22728=CARTESIAN_POINT ( 'NONE',  ( -22.19870942614620901, 0.7548860820614724521, -22.74607621399518465 ) ) ;
#22729=CARTESIAN_POINT ( 'NONE',  ( -20.49308933001933397, -27.11270025041355680, -6.352872742357712710 ) ) ;
#22731=CARTESIAN_POINT ( 'NONE',  ( 34.06363962356728337, -8.139266223780131426, -8.939444182090305446 ) ) ;
#22743=( NAMED_UNIT ( * ) PLANE_ANGLE_UNIT ( ) SI_UNIT ( $, .RADIAN. ) );
#22744=CARTESIAN_POINT ( 'NONE',  ( 2.406372317666654492, 20.36914331218811824, -30.00000000000001776 ) ) ;
#22747=CARTESIAN_POINT ( 'NONE',  ( 17.71135169000040932, 20.05059954136391553, -5.000000000000002665 ) ) ;
#22748=CARTESIAN_POINT ( 'NONE',  ( 6.687105839631831472, 20.72947162859387404, -24.48960877912796263 ) ) ;
#22752=CARTESIAN_POINT ( 'NONE',  ( 16.20011322261754216, -26.49736879530895806, -8.260367887910364360 ) ) ;
#22757=CARTESIAN_POINT ( 'NONE',  ( -15.37168272651113199, 26.67356397381335142, -6.417197371198677835 ) ) ;
#22760=CARTESIAN_POINT ( 'NONE',  ( 11.13984957941081433, -21.02844965650029962, -19.53953216799471448 ) ) ;
#22766=CARTESIAN_POINT ( 'NONE',  ( -12.12099249900222731, 26.27303737746609613, -14.20430146812667083 ) ) ;
#22770=CARTESIAN_POINT ( 'NONE',  ( -34.38052266744621477, -7.499778090769174455, -8.068316597692506420 ) ) ;
#22773=CARTESIAN_POINT ( 'NONE',  ( 20.52133710794606358, 0.9695505216964825923, -28.71086575011983300 ) ) ;
#22774=CARTESIAN_POINT ( 'NONE',  ( 15.34996087503667361, 26.64851995519817152, -6.887892877121212010 ) ) ;
#22778=CARTESIAN_POINT ( 'NONE',  ( -30.35055362032863613, -0.002292147019176501987, -8.297710457928772598 ) ) ;
#22781=CARTESIAN_POINT ( 'NONE',  ( 24.63269681886077223, -1.423661518239742518, -19.25494299242245688 ) ) ;
#22798=CARTESIAN_POINT ( 'NONE',  ( -19.81925457214680719, 7.205556427748036619, -24.35504295706233790 ) ) ;
#22800=CARTESIAN_POINT ( 'NONE',  ( 20.87224371475484475, -27.19134377947485248, -5.902448757945053970 ) ) ;
#22804=CARTESIAN_POINT ( 'NONE',  ( 11.77217231312305223, 19.50978363648416547, -21.59411333990740545 ) ) ;
#22806=CARTESIAN_POINT ( 'NONE',  ( -14.31861646336927230, 22.24101317123190569, -14.54554263817891702 ) ) ;
#22810=CARTESIAN_POINT ( 'NONE',  ( 12.43267688036053187, 20.43562119112951692, -19.50373040854491080 ) ) ;
#22813=CARTESIAN_POINT ( 'NONE',  ( 22.53426880051877035, -12.42977529295302652, -19.62973737113728490 ) ) ;
#22816=CARTESIAN_POINT ( 'NONE',  ( -14.69713093287458427, 26.03946747147639584, -10.15458874994915028 ) ) ;
#22818=CARTESIAN_POINT ( 'NONE',  ( -13.61946501912157714, -23.12974890171631870, -15.38845843242090261 ) ) ;
#22820=AXIS2_PLACEMENT_3D ( 'NONE', #25151, #6265, #31253 ) ;
#22822=CARTESIAN_POINT ( 'NONE',  ( -29.46499357413496867, -13.19446224756526220, -13.82164065331125968 ) ) ;
#22823=CARTESIAN_POINT ( 'NONE',  ( -14.23983225781402417, -26.43328798539083735, -5.474040432887671948 ) ) ;
#22825=CARTESIAN_POINT ( 'NONE',  ( 16.14888623509959942, 20.94233928415653168, -11.72143342499177088 ) ) ;
#22827=CARTESIAN_POINT ( 'NONE',  ( 20.22268228429073034, 4.508760637809952954, -27.05330256971496539 ) ) ;
#22831=CARTESIAN_POINT ( 'NONE',  ( -20.48845606910846939, 0.6931994281368786259, -30.00000000000000000 ) ) ;
#22832=CARTESIAN_POINT ( 'NONE',  ( 20.54489790006002892, 0.3835546433576813574, -28.69025006841924963 ) ) ;
#22836=CARTESIAN_POINT ( 'NONE',  ( -16.24796006241077961, 15.88921519459651499, -21.50719306941234876 ) ) ;
#22844=CARTESIAN_POINT ( 'NONE',  ( 17.00000000000000000, 22.50000000000000711, 6.000000000000000000 ) ) ;
#22848=CARTESIAN_POINT ( 'NONE',  ( 19.20779205614405072, -16.68223394817295713, -19.73749630327306903 ) ) ;
#22851=CARTESIAN_POINT ( 'NONE',  ( 10.95309464140887812, 18.88199699059095948, -23.77075622942746591 ) ) ;
#22854=CARTESIAN_POINT ( 'NONE',  ( -17.77135203137562058, 19.64225148421929390, -6.915705780155396276 ) ) ;
#22857=CARTESIAN_POINT ( 'NONE',  ( 14.71950235153890141, -25.64848556417364378, -10.18105174685851999 ) ) ;
#22859=CARTESIAN_POINT ( 'NONE',  ( 15.30169432489863013, 26.49078902709227989, -7.357960067667439930 ) ) ;
#22861=CARTESIAN_POINT ( 'NONE',  ( 12.39027692975310124, 20.49132159761027339, -19.49634355596792901 ) ) ;
#22863=CARTESIAN_POINT ( 'NONE',  ( -10.95909218333906487, 17.37826635768778516, -28.70499877695077373 ) ) ;
#22865=CARTESIAN_POINT ( 'NONE',  ( -12.61201992331770150, -22.55708276399396794, -16.44710463512250342 ) ) ;
#22868=CARTESIAN_POINT ( 'NONE',  ( -30.92005800807112337, -19.98835077949903294, -9.284583649112713388 ) ) ;
#22869=CARTESIAN_POINT ( 'NONE',  ( -4.809173904559163937, -24.92317228705597287, -5.480779845647450799 ) ) ;
#22870=CARTESIAN_POINT ( 'NONE',  ( 11.64932880570667351, 17.76966214386914800, -25.05926785085788211 ) ) ;
#22872=CARTESIAN_POINT ( 'NONE',  ( 23.08742108726735864, 9.144738169211333201, -8.888958855014557514 ) ) ;
#22874=CARTESIAN_POINT ( 'NONE',  ( -14.89115357024799380, -26.59122515138228948, -5.000000000000000000 ) ) ;
#22877=CARTESIAN_POINT ( 'NONE',  ( -28.78671411640772959, -1.326716728304855542, -13.36536875498820720 ) ) ;
#22879=EDGE_LOOP ( 'NONE', ( #36032, #3191 ) ) ;
#22882=CARTESIAN_POINT ( 'NONE',  ( 34.61427093075294437, -16.43137713082842666, -5.857256890622249301 ) ) ;
#22885=ADVANCED_FACE ( 'NONE', ( #30984 ), #5992, .F. ) ;
#22894=CARTESIAN_POINT ( 'NONE',  ( -1.688293718737135851, 33.40510209930049257, -12.89208270232461828 ) ) ;
#22902=CARTESIAN_POINT ( 'NONE',  ( 9.714866619683970583, 18.51369873714040537, -26.70036842142175004 ) ) ;
#22903=CARTESIAN_POINT ( 'NONE',  ( 30.90412082983250741, -0.04211290444289944590, -5.000000000000000000 ) ) ;
#22905=CARTESIAN_POINT ( 'NONE',  ( -18.33793368410551494, 13.06784656731418437, -17.99966567637481063 ) ) ;
#22909=CARTESIAN_POINT ( 'NONE',  ( 15.53709981414127483, -26.75515487142352100, -5.000000000000000888 ) ) ;
#22911=CARTESIAN_POINT ( 'NONE',  ( 14.51165130258184988, 25.03008843810978235, -11.59459722426760386 ) ) ;
#22913=CARTESIAN_POINT ( 'NONE',  ( -1.775381057445013511E-14, 40.84107189184581443, -14.51648065752882566 ) ) ;
#22916=CARTESIAN_POINT ( 'NONE',  ( -23.57342501307383387, -22.18880773095553138, -12.97801393859235297 ) ) ;
#22917=CARTESIAN_POINT ( 'NONE',  ( 7.182736407388268240, -19.60433374307056908, -26.43616374447599426 ) ) ;
#22918=CARTESIAN_POINT ( 'NONE',  ( 14.90956390896501915, 25.40097293458214622, -10.18423201954005641 ) ) ;
#22919=CARTESIAN_POINT ( 'NONE',  ( 18.41239260963195790, 13.48770510890848051, -16.96331977760756970 ) ) ;
#22926=CARTESIAN_POINT ( 'NONE',  ( -5.279954849186515808, 19.80786611602342973, -29.24590087848358877 ) ) ;
#22928=CARTESIAN_POINT ( 'NONE',  ( -11.07691353229041731, -20.48794067953776477, -20.55402119402114991 ) ) ;
#22932=CARTESIAN_POINT ( 'NONE',  ( 27.77418311698831488, 0.1426534356837458328, -13.50886777650709902 ) ) ;
#22936=CARTESIAN_POINT ( 'NONE',  ( -30.51319350132663288, 0.08894917402604617107, -7.358348470158322385 ) ) ;
#22938=CARTESIAN_POINT ( 'NONE',  ( 32.69488556240459332, -8.773221015582116422, -11.16016912004820050 ) ) ;
#22940=ORIENTED_EDGE ( 'NONE', *, *, #18338, .F. ) ;
#22953=CARTESIAN_POINT ( 'NONE',  ( 15.17029220080370600, 14.77339687257036260, -24.28810107756022063 ) ) ;
#22954=CARTESIAN_POINT ( 'NONE',  ( 9.102363436486372805, 31.45286188096421043, -12.09631145245175077 ) ) ;
#22959=CARTESIAN_POINT ( 'NONE',  ( 16.10155988989870934, -26.68239398247207461, -7.337369887910988098 ) ) ;
#22963=CARTESIAN_POINT ( 'NONE',  ( -12.66689476310357598, 21.03365424557304664, -18.45460298430356616 ) ) ;
#22966=CARTESIAN_POINT ( 'NONE',  ( 14.88849274807932765, -26.59100623965352739, -5.000000000000000888 ) ) ;
#22971=CARTESIAN_POINT ( 'NONE',  ( -8.376537992280214340, 19.04457702326376278, -27.24859099131081663 ) ) ;
#22972=CARTESIAN_POINT ( 'NONE',  ( -16.05099858185807449, -21.51520586029840842, -17.05908743202043709 ) ) ;
#22974=CIRCLE ( 'NONE', #9359, 59.99999999999998579 ) ;
#22975=CARTESIAN_POINT ( 'NONE',  ( -21.19038336318232751, -5.228579731333282687, -24.44094102819527947 ) ) ;
#22978=CARTESIAN_POINT ( 'NONE',  ( 30.39593018562074178, 0.08170413101267633149, -7.828442670039330586 ) ) ;
#22979=CARTESIAN_POINT ( 'NONE',  ( 12.13489577590003776, 19.91918274404604361, -20.54176213831676634 ) ) ;
#22982=CARTESIAN_POINT ( 'NONE',  ( -26.51672392814666779, 0.2580214034863175243, -15.44851676060052270 ) ) ;
#22985=CARTESIAN_POINT ( 'NONE',  ( 33.76045296747373925, -4.171667482292196638, -6.352430751017280386 ) ) ;
#22989=ORIENTED_EDGE ( 'NONE', *, *, #26093, .F. ) ;
#22998=B_SPLINE_SURFACE_WITH_KNOTS ( 'NONE', 3, 3, ( 
 ( #30800, #33854, #24299, #40129 ),
 ( #5606, #36301, #3163, #12305 ),
 ( #12501, #33661, #8663, #27544 ),
 ( #27149, #18015, #15554, #5411 ),
 ( #17823, #24694, #39929, #2964 ),
 ( #21249, #18211, #15351, #36893 ),
 ( #9258, #30603, #8463, #18608 ),
 ( #8862, #2374, #27740, #14759 ),
 ( #2571, #14956, #27344, #36494 ),
 ( #37091, #30993, #21643, #9063 ),
 ( #21448, #24099, #116, #34046 ),
 ( #20862, #38077, #37877, #10250 ),
 ( #9462, #9665, #34441, #13289 ),
 ( #3555, #34243, #31580, #35040 ),
 ( #25684, #15749, #16349, #6398 ),
 ( #22042, #513, #18804, #709 ),
 ( #10052, #6592, #12696, #19193 ),
 ( #18997, #34836, #15952, #31387 ),
 ( #24893, #28138, #28732, #28332 ),
 ( #31786, #19390, #7193, #315 ),
 ( #12897, #1114, #25289, #3950 ),
 ( #911, #19592, #22634, #13087 ),
 ( #37685, #31982, #37287, #3747 ),
 ( #22231, #9853, #31191, #25477 ),
 ( #3356, #25090, #34635, #37487 ),
 ( #6788, #4148, #16554, #28936 ),
 ( #21840, #16151, #28535, #22431 ),
 ( #6984, #4353, #8210, #23452 ),
 ( #17571, #38892, #29144, #26698 ),
 ( #11068, #16963, #17373, #26084 ),
 ( #13492, #10863, #36048, #19800 ),
 ( #23251, #38484, #4762, #35235 ),
 ( #23041, #20614, #22836, #7393 ),
 ( #29745, #32605, #35842, #32405 ),
 ( #38690, #8003, #20208, #1314 ),
 ( #10659, #1724, #5163, #14100 ),
 ( #33013, #29943, #25884, #35649 ),
 ( #7600, #35445, #13696, #20006 ),
 ( #38283, #20412, #4559, #32808 ),
 ( #10453, #32194, #29343, #7805 ),
 ( #14304, #1514, #13904, #16759 ),
 ( #26295, #17169, #1928, #29545 ),
 ( #26497, #4966, #23652, #39085 ),
 ( #11263, #33806, #23850, #17967 ) ),
 .UNSPECIFIED., .T., .F., .F.,
 ( 4, 1, 1, 1, 2, 1, 1, 1, 1, 1, 1, 1, 2, 1, 1, 1, 2, 1, 1, 1, 1, 1, 1, 1, 2, 1, 1, 1, 2, 1, 1, 1, 1, 1, 1, 1, 4 ),
 ( 4, 4 ),
 ( 0.000000000000000000, 0.03553882639362128393, 0.07107765278724256786, 0.1066164791808638657, 0.1421553055744851357, 0.1660525590443411859, 0.1899498125141971805, 0.2138470659840532306, 0.2377443194539092253, 0.2616415729237652754, 0.2855388263936212701, 0.3094360798634773202, 0.3333333333333333703, 0.3688721597269547514, 0.4044109861205760215, 0.4399498125141973470, 0.4754886389078186171, 0.4993858923776745562, 0.5232831458475305508, 0.5471803993173864900, 0.5710776527872425401, 0.5949749062570985902, 0.6188721597269547514, 0.6427694131968104685, 0.6666666666666665186, 0.7022054930602876777, 0.7377443194539090587, 0.7732831458475302178, 0.8088219722411513768, 0.8327192257110074269, 0.8566164791808634771, 0.8805137326507195272, 0.9044109861205756884, 0.9283082395904318496, 0.9522054930602878997, 0.9761027465301439499, 1.000000000000000000 ),
 ( 0.000000000000000000, 1.000000000000000000 ),
 .UNSPECIFIED. ) ;
#23002=CARTESIAN_POINT ( 'NONE',  ( -23.58808727774059832, 8.960771098271621327, -5.000000000000000000 ) ) ;
#23003=CARTESIAN_POINT ( 'NONE',  ( 21.98490994300607682, -27.05380718176246901, -5.895602069099679099 ) ) ;
#23007=CARTESIAN_POINT ( 'NONE',  ( 10.84452725066743106, 17.39679239189240434, -29.34533630210047406 ) ) ;
#23010=CARTESIAN_POINT ( 'NONE',  ( -11.99665585415270996, 16.62659876986841567, -30.00000000000000000 ) ) ;
#23013=CARTESIAN_POINT ( 'NONE',  ( 11.04912124349541713, 17.32038412190906840, -28.70874619594562915 ) ) ;
#23015=CARTESIAN_POINT ( 'NONE',  ( 17.94885553750267349, -9.904091770223047320, -30.00000000000002842 ) ) ;
#23018=CARTESIAN_POINT ( 'NONE',  ( -10.93774750043060706, 17.74170758838544160, -26.81279356920407864 ) ) ;
#23021=CARTESIAN_POINT ( 'NONE',  ( -10.04686839703753876, -18.12954247328852020, -27.41699321995579908 ) ) ;
#23025=CARTESIAN_POINT ( 'NONE',  ( -35.02447263591297855, -13.24401549867776318, -7.135927747732872639 ) ) ;
#23026=CARTESIAN_POINT ( 'NONE',  ( -9.169462346764058580, -18.33493501355543742, -29.35491832476872176 ) ) ;
#23028=CARTESIAN_POINT ( 'NONE',  ( 15.06161168841436471, 19.05444440493321423, -16.70087182429124084 ) ) ;
#23030=CARTESIAN_POINT ( 'NONE',  ( 27.43674297377669546, 3.779828424379618301, -5.000000000000001776 ) ) ;
#23034=CARTESIAN_POINT ( 'NONE',  ( -24.64392587737382456, 0.2590282008007734893, -18.42865202136458436 ) ) ;
#23036=CARTESIAN_POINT ( 'NONE',  ( 21.79677046812914654, 0.2436873253541234352, -23.79487705795048313 ) ) ;
#23039=CARTESIAN_POINT ( 'NONE',  ( -23.05051288410620103, 1.290431267577835772, -20.62872711280308025 ) ) ;
#23041=CARTESIAN_POINT ( 'NONE',  ( -19.79815887584811307, 19.84782313723621883, -4.999999999999999112 ) ) ;
#23044=AXIS2_PLACEMENT_3D ( 'NONE', #39594, #30057, #27009 ) ;
#23047=EDGE_CURVE ( 'NONE', #8550, #1290, #34995, .T. ) ;
#23055=CARTESIAN_POINT ( 'NONE',  ( 25.40476810523085760, -22.14310417253436469, -12.02608197892994468 ) ) ;
#23058=CARTESIAN_POINT ( 'NONE',  ( 15.10103005678714894, 27.38430384138463225, -6.871694316642929401 ) ) ;
#23059=CARTESIAN_POINT ( 'NONE',  ( 0.000000000000000000, 22.50000000000000355, 3.000000000000000000 ) ) ;
#23061=CARTESIAN_POINT ( 'NONE',  ( -14.44435570328332652, 14.60131355992008473, -28.82039636960078255 ) ) ;
#23063=CARTESIAN_POINT ( 'NONE',  ( 15.27748152860279518, -26.61456374246583678, -6.417151305163597996 ) ) ;
#23065=CARTESIAN_POINT ( 'NONE',  ( 15.42339932183901752, 26.75673767418847859, -5.000000000000002665 ) ) ;
#23067=CARTESIAN_POINT ( 'NONE',  ( 11.68277618612572866, 18.91466778193324672, -22.73465507004121733 ) ) ;
#23070=CARTESIAN_POINT ( 'NONE',  ( -13.73783782086621308, 23.46750919750577680, -14.46876710495131313 ) ) ;
#23073=CARTESIAN_POINT ( 'NONE',  ( -12.64202328258549990, -22.55724117488063030, -16.44518350383058447 ) ) ;
#23078=CARTESIAN_POINT ( 'NONE',  ( -25.88132202143377469, -15.63261420755070930, -15.67704684687844185 ) ) ;
#23079=CARTESIAN_POINT ( 'NONE',  ( -9.295420884976664411, -25.43675055676933638, -4.999999999999999112 ) ) ;
#23080=CARTESIAN_POINT ( 'NONE',  ( 11.85474644856143378, 17.60367872427052305, -25.08547864272203398 ) ) ;
#23082=CARTESIAN_POINT ( 'NONE',  ( 23.30655953786771661, 8.157976315886919849, -10.85338692621293077 ) ) ;
#23086=ADVANCED_BREP_SHAPE_REPRESENTATION ( '', ( #9362, #24238 ), #9333 ) ;
#23087=CARTESIAN_POINT ( 'NONE',  ( -32.18856600309058535, -1.666818702012493381, -6.386702722256275777 ) ) ;
#23092=CARTESIAN_POINT ( 'NONE',  ( 31.34477257452704535, -13.70488752507857910, -11.99102932043097169 ) ) ;
#23098=CARTESIAN_POINT ( 'NONE',  ( -15.42743469815759028, 26.74224822490523579, -5.000000000000002665 ) ) ;
#23102=ORIENTED_EDGE ( 'NONE', *, *, #7842, .T. ) ;
#23103=CARTESIAN_POINT ( 'NONE',  ( -0.7219791468970899739, 36.56720658881546626, -9.725050104156155228 ) ) ;
#23110=CARTESIAN_POINT ( 'NONE',  ( 9.501231361094543360, 18.85103192176102738, -26.04902248843100665 ) ) ;
#23113=CARTESIAN_POINT ( 'NONE',  ( -17.34395368315986730, 11.20622719433779757, -27.17580777125886726 ) ) ;
#23116=CARTESIAN_POINT ( 'NONE',  ( 9.514046198846664026, -18.15855281542499000, -30.00000000000000000 ) ) ;
#23118=CARTESIAN_POINT ( 'NONE',  ( 11.65547513713623573, 18.94099047327305740, -22.72982294686783789 ) ) ;
#23119=CARTESIAN_POINT ( 'NONE',  ( -16.84920187454418539, 29.09530251867925443, -5.000000000000000000 ) ) ;
#23121=CARTESIAN_POINT ( 'NONE',  ( -14.94827155352230186, -14.02787326271796609, -30.00000000000001421 ) ) ;
#23122=CARTESIAN_POINT ( 'NONE',  ( 7.004305706416510624, -19.31551653162770776, -29.39181977775634991 ) ) ;
#23123=CARTESIAN_POINT ( 'NONE',  ( 14.41205314296764683, 24.16671282165543388, -12.56218448904276741 ) ) ;
#23124=CARTESIAN_POINT ( 'NONE',  ( 20.57095190365273396, 13.97674357447790250, -4.999999999999997335 ) ) ;
#23130=CARTESIAN_POINT ( 'NONE',  ( -6.337285794301795505, 36.78338214817075880, -7.138834133703192641 ) ) ;
#23132=CARTESIAN_POINT ( 'NONE',  ( -14.47023594716632999, -25.43102382604878642, -10.65652329803860532 ) ) ;
#23141=CARTESIAN_POINT ( 'NONE',  ( -20.69120578336301008, 0.8799204947885410633, -27.45047952108874512 ) ) ;
#23143=CARTESIAN_POINT ( 'NONE',  ( 33.35964565017460615, -8.962426252800922200, -10.25865101404451352 ) ) ;
#23146=B_SPLINE_CURVE_WITH_KNOTS ( 'NONE', 3,
 ( #10168, #3664, #16059, #28447, #819, #13200, #34951, #31698, #25594, #7105, #22744, #22148, #19109, #35147, #19501, #19707, #4264, #31895, #37602, #37790, #31302, #3469, #37395, #25799, #6900, #4058, #16463, #1024, #25003, #7301, #623, #28049, #32099, #16262, #34354, #13405, #9571, #227, #12612, #21953, #6503, #18909, #15864, #13004, #9768, #25392, #28250, #427, #34750, #12807, #25204, #6700, #34549, #31501, #9964, #22344, #13806, #16874, #7913, #26199, #29850, #26804, #35957, #29253 ),
 .UNSPECIFIED., .F., .F.,
 ( 4, 2, 2, 2, 2, 2, 2, 2, 2, 2, 2, 2, 2, 2, 2, 2, 2, 2, 2, 2, 2, 2, 2, 2, 2, 2, 2, 2, 2, 2, 2, 4 ),
 ( 0.06544620927018722500, 0.06740620535651276057, 0.06838620339967552142, 0.06936620144283828227, 0.07328619361548933953, 0.07524618970181487509, 0.07622618774497763594, 0.07720618578814039679, 0.08112617796079146792, 0.08210617600395422877, 0.08308617404711698962, 0.08504617013344251131, 0.08896616230609356857, 0.08994616034925632941, 0.09092615839241909026, 0.09288615447874459807, 0.09484615056507009201, 0.09582614860823285285, 0.09680614665139561370, 0.1007261388240466016, 0.1026861349103721094, 0.1036661329535348564, 0.1046461309966976172, 0.1085661231693486051, 0.1105261192556741129, 0.1124861153419996207, 0.1164061075146506086, 0.1183661036009761164, 0.1203260996873016242, 0.1222860957736271181, 0.1242460918599526259, 0.1281660840326036277 ),
 .UNSPECIFIED. ) ;
#23156=CARTESIAN_POINT ( 'NONE',  ( 15.66611865990399188, 14.17652996785340314, -24.32473454633646170 ) ) ;
#23158=CARTESIAN_POINT ( 'NONE',  ( 7.918914183234117665, 24.62754220467781607, -18.88895522463596066 ) ) ;
#23163=CARTESIAN_POINT ( 'NONE',  ( 14.62307350666250727, -24.21852764430928318, -13.43612557937942142 ) ) ;
#23168=CARTESIAN_POINT ( 'NONE',  ( -11.02828492200578658, 17.43271654862448372, -28.07671141248061275 ) ) ;
#23170=CARTESIAN_POINT ( 'NONE',  ( 14.73837995999511641, -26.18078596994419271, -8.300944784147242572 ) ) ;
#23175=CARTESIAN_POINT ( 'NONE',  ( -13.28590053108947799, 29.03689826311631350, -9.996870771847651937 ) ) ;
#23179=CARTESIAN_POINT ( 'NONE',  ( -20.12188542190007468, -4.958127744699047490, -27.81140718703422010 ) ) ;
#23182=CARTESIAN_POINT ( 'NONE',  ( 30.64998978746207570, 0.1153925296135153711, -6.417209882492363349 ) ) ;
#23189=CARTESIAN_POINT ( 'NONE',  ( -20.48235837767022716, 0.8503560580662928858, -29.34820720422862550 ) ) ;
#23191=ORIENTED_EDGE ( 'NONE', *, *, #33006, .F. ) ;
#23192=CARTESIAN_POINT ( 'NONE',  ( 30.96795480659843847, -2.880468441431110360, -11.37706435339893041 ) ) ;
#23208=ADVANCED_FACE ( 'NONE', ( #26632 ), #33146, .T. ) ;
#23209=CARTESIAN_POINT ( 'NONE',  ( 3.650831912126976331, 27.51027965810262543, -17.63966039508103023 ) ) ;
#23212=CARTESIAN_POINT ( 'NONE',  ( -22.21927468398150296, 10.75596765700722024, -7.916699199386848740 ) ) ;
#23213=CARTESIAN_POINT ( 'NONE',  ( 14.40695447559362918, -17.97978767915237341, -22.25716284559454650 ) ) ;
#23218=CARTESIAN_POINT ( 'NONE',  ( 15.25445287089756441, 26.65416740092992498, -7.354337790751865889 ) ) ;
#23221=CARTESIAN_POINT ( 'NONE',  ( -12.79219479534856774, 19.13966889506235347, -20.65395721553354846 ) ) ;
#23225=CARTESIAN_POINT ( 'NONE',  ( 11.03950910960345766, 17.27365618835783678, -29.34954168035285704 ) ) ;
#23227=CARTESIAN_POINT ( 'NONE',  ( 23.87817301747191934, -12.24222096213839706, -18.61666795014612674 ) ) ;
#23230=CARTESIAN_POINT ( 'NONE',  ( -10.93239227196862906, 17.93597283121687269, -26.19762304272490638 ) ) ;
#23232=CARTESIAN_POINT ( 'NONE',  ( -15.80249673657252529, -25.67169305692603842, -10.58215573314341462 ) ) ;
#23234=DIRECTION ( 'NONE',  ( -1.000000000000000000, 2.602085213965210642E-15, 0.000000000000000000 ) ) ;
#23237=CARTESIAN_POINT ( 'NONE',  ( -18.92370352201584538, -8.520676925239653698, -27.71828468939111545 ) ) ;
#23238=CARTESIAN_POINT ( 'NONE',  ( -12.50179810955727966, -23.06732317427903922, -15.48378489298444549 ) ) ;
#23240=CARTESIAN_POINT ( 'NONE',  ( 17.21933148029187421, 21.00599287609430732, -6.908854110444175411 ) ) ;
#23242=CARTESIAN_POINT ( 'NONE',  ( 22.98885138662875960, 3.755270039684655892, -18.76986221281831391 ) ) ;
#23246=CARTESIAN_POINT ( 'NONE',  ( -30.99742014632522569, -0.1379718400911539578, -4.999999999999999112 ) ) ;
#23247=CARTESIAN_POINT ( 'NONE',  ( 26.83762895626454537, -0.2330588716970352914, -15.38901361913504928 ) ) ;
#23250=CARTESIAN_POINT ( 'NONE',  ( -28.19786622711188784, 2.629271227132516486, -7.374041015958935574 ) ) ;
#23251=CARTESIAN_POINT ( 'NONE',  ( -23.06249103411543544, 13.31513540672989926, -4.999999999999996447 ) ) ;
#23262=CARTESIAN_POINT ( 'NONE',  ( -22.33022999260465724, 5.911010040927092035, -17.87267886299877162 ) ) ;
#23265=CARTESIAN_POINT ( 'NONE',  ( 20.87822957844602456, -19.29698014627262737, -16.74541713236688167 ) ) ;
#23268=CARTESIAN_POINT ( 'NONE',  ( 14.16267402188527313, 24.80506001027335472, -12.52237342293435240 ) ) ;
#23269=ORIENTED_EDGE ( 'NONE', *, *, #32917, .F. ) ;
#23270=CARTESIAN_POINT ( 'NONE',  ( -17.22179567822546176, 20.49768920708832454, -8.352296547685462258 ) ) ;
#23272=CARTESIAN_POINT ( 'NONE',  ( 11.85325580602118301, -21.48896600845587557, -18.45743837482206828 ) ) ;
#23274=CARTESIAN_POINT ( 'NONE',  ( 14.85248842483373188, 25.57170511055247175, -10.18105171841187584 ) ) ;
#23276=CARTESIAN_POINT ( 'NONE',  ( 12.12763111783735503, 19.92791405175542607, -20.54027923519833010 ) ) ;
#23278=CARTESIAN_POINT ( 'NONE',  ( -10.99314221940617564, 17.45576443972036529, -28.07461421731269979 ) ) ;
#23280=CARTESIAN_POINT ( 'NONE',  ( -14.86193584663134892, -25.83070395712688949, -9.709670777925021312 ) ) ;
#23285=CARTESIAN_POINT ( 'NONE',  ( -26.84768961812649835, -16.21779228968876652, -14.72956622491983758 ) ) ;
#23286=CARTESIAN_POINT ( 'NONE',  ( -5.926965089342771442, -22.63169345552070055, -16.85668200393126526 ) ) ;
#23287=CARTESIAN_POINT ( 'NONE',  ( 11.69146759026597238, 16.83997637742415776, -29.36300835845053570 ) ) ;
#23290=CARTESIAN_POINT ( 'NONE',  ( 23.35054822394877760, 9.216580574185069707, -6.449451739544402429 ) ) ;
#23295=CARTESIAN_POINT ( 'NONE',  ( -27.79641046810536054, -1.962788507153767847, -15.20952948633108193 ) ) ;
#23302=CARTESIAN_POINT ( 'NONE',  ( 34.10630787157268884, -17.48172648250967143, -6.276852260651874182 ) ) ;
#23312=ORIENTED_EDGE ( 'NONE', *, *, #19398, .F. ) ;
#23313=CARTESIAN_POINT ( 'NONE',  ( 1.051372576265723557, 25.72197380671092048, -19.63089720651151282 ) ) ;
#23320=CARTESIAN_POINT ( 'NONE',  ( 12.11678078314277762, 23.99614306916164708, -16.23412490227547522 ) ) ;
#23322=ORIENTED_EDGE ( 'NONE', *, *, #24930, .F. ) ;
#23323=CARTESIAN_POINT ( 'NONE',  ( -20.20456973212974106, 14.66708349146731827, -5.482234822857553702 ) ) ;
#23326=CARTESIAN_POINT ( 'NONE',  ( 13.74681413364860383, -24.12214955346338741, -13.51035512735945154 ) ) ;
#23328=CARTESIAN_POINT ( 'NONE',  ( 15.27289138331547669, 26.59085539454768821, -7.356080397504305424 ) ) ;
#23329=CARTESIAN_POINT ( 'NONE',  ( -19.54664213359414404, -11.28525909758381651, -19.69475445967427163 ) ) ;
#23332=CARTESIAN_POINT ( 'NONE',  ( -22.15736500781834906, -20.84727699870213868, -14.83950653091789817 ) ) ;
#23333=CARTESIAN_POINT ( 'NONE',  ( 4.192399910511806382, -20.06660217949758618, -29.41646740880849364 ) ) ;
#23334=CARTESIAN_POINT ( 'NONE',  ( 11.85241674728229988, 18.75149653998677124, -22.76202379300414691 ) ) ;
#23336=CARTESIAN_POINT ( 'NONE',  ( 17.07516244282002660, 12.28144768211119953, -24.39718017846627518 ) ) ;
#23339=CARTESIAN_POINT ( 'NONE',  ( -7.410464713192979502, 36.46669482336120183, -6.720204936114559935 ) ) ;
#23348=CARTESIAN_POINT ( 'NONE',  ( -22.70365180105937242, 0.7008854888786294479, -21.62861051218136055 ) ) ;
#23349=ORIENTED_EDGE ( 'NONE', *, *, #32271, .T. ) ;
#23350=CARTESIAN_POINT ( 'NONE',  ( 35.11092860954450856, -11.76153023245262297, -7.147189329740518460 ) ) ;
#23365=CARTESIAN_POINT ( 'NONE',  ( 18.42725648993722842, 16.20988549689709757, -11.84062711183378092 ) ) ;
#23366=CARTESIAN_POINT ( 'NONE',  ( 6.331554793186663588, 19.58397683058095140, -28.53572403070387864 ) ) ;
#23371=CARTESIAN_POINT ( 'NONE',  ( 15.36935833352434777, -25.93966974496969513, -9.682725942216546144 ) ) ;
#23372=CARTESIAN_POINT ( 'NONE',  ( 37.19292564617598629, -15.51005328467150512, -4.999999999999994671 ) ) ;
#23375=VERTEX_POINT ( 'NONE', #21141 ) ;
#23376=CARTESIAN_POINT ( 'NONE',  ( -11.68537700245894762, 18.91218677661948888, -22.73505939135654330 ) ) ;
#23378=CARTESIAN_POINT ( 'NONE',  ( 11.39961882692148087, -22.05299179249424313, -17.51387407834204168 ) ) ;
#23382=CARTESIAN_POINT ( 'NONE',  ( -7.682719301950634794, 20.99212371924112119, -23.35384790439877278 ) ) ;
#23386=CARTESIAN_POINT ( 'NONE',  ( -32.20191614452445350, -5.996939808026042762, -11.23890058235647160 ) ) ;
#23389=CARTESIAN_POINT ( 'NONE',  ( 20.80995787673824893, 0.8960491595669888287, -26.83562114098080187 ) ) ;
#23394=CARTESIAN_POINT ( 'NONE',  ( -30.63049699552009031, -0.03312779925433120137, -7.357393045505457252 ) ) ;
#23397=CARTESIAN_POINT ( 'NONE',  ( 26.43890877042912990, -2.343727469559957033, -17.12617500785380997 ) ) ;
#23399=ORIENTED_EDGE ( 'NONE', *, *, #21959, .F. ) ;
#23409=CARTESIAN_POINT ( 'NONE',  ( 4.110008236141186266, 30.79763600885550190, -14.76321218211128716 ) ) ;
#23416=CARTESIAN_POINT ( 'NONE',  ( 19.84635048062218488, -25.97363186618970943, -9.943601658171525415 ) ) ;
#23420=CARTESIAN_POINT ( 'NONE',  ( 11.22254838620092343, 18.10604511926858962, -25.00253263116462321 ) ) ;
#23422=CARTESIAN_POINT ( 'NONE',  ( -11.31188296672360671, 17.14851204919853345, -28.71951328966818906 ) ) ;
#23425=CARTESIAN_POINT ( 'NONE',  ( 12.17448594789072303, 19.87244906308695036, -20.54873440190374012 ) ) ;
#23427=CARTESIAN_POINT ( 'NONE',  ( 17.33150493693412031, -10.96591108411289639, -29.21252997676894481 ) ) ;
#23430=CARTESIAN_POINT ( 'NONE',  ( -10.72859233046692395, 17.88194238571141170, -26.79320594746885931 ) ) ;
#23431=LINE ( 'NONE', #36234, #3037 ) ;
#23432=CARTESIAN_POINT ( 'NONE',  ( -11.02901866483229121, -18.34862447518570505, -24.88864236400666030 ) ) ;
#23435=CARTESIAN_POINT ( 'NONE',  ( -27.44899772917025871, -12.30322565212499342, -15.69884287347142404 ) ) ;
#23436=CARTESIAN_POINT ( 'NONE',  ( -10.23778664914769720, -19.66181284788236994, -22.77101389171386003 ) ) ;
#23438=CARTESIAN_POINT ( 'NONE',  ( 15.53819178773900589, 18.26476869418323190, -16.75515271693409147 ) ) ;
#23440=CARTESIAN_POINT ( 'NONE',  ( 28.94531653062197307, 1.996249385887188810, -5.947783999245325859 ) ) ;
#23445=CARTESIAN_POINT ( 'NONE',  ( -21.75755899457715259, 0.4677864005904093236, -23.82221529625467227 ) ) ;
#23446=CARTESIAN_POINT ( 'NONE',  ( 20.49706908807578287, 0.3883427504116045981, -29.33974050869597150 ) ) ;
#23451=CARTESIAN_POINT ( 'NONE',  ( -20.74887948658896164, 1.506378959947736629, -26.88035768992763508 ) ) ;
#23452=CARTESIAN_POINT ( 'NONE',  ( -22.45323650136969462, -2.382502413133420038, -30.00000000000000000 ) ) ;
#23460=CARTESIAN_POINT ( 'NONE',  ( -24.28833252230154827, 5.197361523840480224, -13.76725034441404460 ) ) ;
#23463=CARTESIAN_POINT ( 'NONE',  ( 20.76506965807099192, -18.05532636877229180, -17.69242679302543664 ) ) ;
#23466=CARTESIAN_POINT ( 'NONE',  ( 12.72381738783331251, 21.98735769358159686, -17.39217821953997145 ) ) ;
#23469=CARTESIAN_POINT ( 'NONE',  ( -16.79589040972348002, 21.53745278782425032, -8.341412201671980498 ) ) ;
#23471=CARTESIAN_POINT ( 'NONE',  ( 10.76785045493358339, -20.00693649655310580, -21.62580521813471535 ) ) ;
#23473=CARTESIAN_POINT ( 'NONE',  ( 12.93818047135676785, 21.63701063370047706, -17.43940108704190450 ) ) ;
#23477=CARTESIAN_POINT ( 'NONE',  ( -10.94041201910780359, 17.33660477453622306, -29.34740466869044440 ) ) ;
#23479=CARTESIAN_POINT ( 'NONE',  ( -15.48655661866953892, -26.71642918275651368, -5.945876010756700580 ) ) ;
#23481=CARTESIAN_POINT ( 'NONE',  ( -32.15735702992046896, -20.77263526992292242, -6.277248360418026252 ) ) ;
#23482=CARTESIAN_POINT ( 'NONE',  ( -6.821084136371410089, -20.84928387019777318, -22.02595131697182751 ) ) ;
#23483=CARTESIAN_POINT ( 'NONE',  ( 15.86158329389953536, 24.87666108630855177, -6.892499796494895747 ) ) ;
#23485=CARTESIAN_POINT ( 'NONE',  ( 22.72982457100355802, 9.046144286754186581, -10.86715459307012033 ) ) ;
#23488=CARTESIAN_POINT ( 'NONE',  ( -15.41367234785094809, -26.72342555440733136, -4.999999999999999112 ) ) ;
#23492=CARTESIAN_POINT ( 'NONE',  ( -20.89685344739347173, -1.175242339315835105, -26.67474265850594506 ) ) ;
#23497=CARTESIAN_POINT ( 'NONE',  ( 29.24088705168217572, -13.85790213908317980, -13.81488898234178642 ) ) ;
#23505=EDGE_CURVE ( 'NONE', #5646, #7027, #33500, .T. ) ;
#23506=CARTESIAN_POINT ( 'NONE',  ( 1.510082208727901110, 36.50975218198507832, -9.726556050585005053 ) ) ;
#23514=CARTESIAN_POINT ( 'NONE',  ( 10.91375165427755789, 19.61687978590818204, -22.60510580339686015 ) ) ;
#23519=CARTESIAN_POINT ( 'NONE',  ( -19.51546397819036827, 15.47399000601905250, -8.398378205727166090 ) ) ;
#23522=CARTESIAN_POINT ( 'NONE',  ( 15.40300567925599395, -26.59730094924787380, -6.887548287194356966 ) ) ;
#23524=CARTESIAN_POINT ( 'NONE',  ( 15.28201387016975232, 26.55918798812530923, -7.356955115318605465 ) ) ;
#23527=CARTESIAN_POINT ( 'NONE',  ( -15.37464264532748004, -13.57371270378507866, -29.23195595578610195 ) ) ;
#23529=CARTESIAN_POINT ( 'NONE',  ( 2.755021161861860080, -20.38581168850896930, -28.85590101152765286 ) ) ;
#23530=CARTESIAN_POINT ( 'NONE',  ( 12.08865418433290806, 19.17331245234230508, -21.65079422309015911 ) ) ;
#23531=CARTESIAN_POINT ( 'NONE',  ( 20.38739101816897659, 13.83500035239263859, -8.405622461330182205 ) ) ;
#23532=CARTESIAN_POINT ( 'NONE',  ( -3.485571585149855434, -11.25000000000002132, 0.000000000000000000 ) ) ;
#23535=CARTESIAN_POINT ( 'NONE',  ( -6.207178120114770437, 35.88840053175069755, -8.874516004040346573 ) ) ;
#23545=EDGE_LOOP ( 'NONE', ( #24061, #6451, #14798, #34008 ) ) ;
#23546=CARTESIAN_POINT ( 'NONE',  ( -30.47170454527866923, 0.4016671284418431020, -5.474069987333029630 ) ) ;
#23548=CARTESIAN_POINT ( 'NONE',  ( 33.42056292424250330, -10.04652305323077144, -10.23864384795611926 ) ) ;
#23565=CARTESIAN_POINT ( 'NONE',  ( 14.79081071437772010, 14.21365739191439737, -29.41171982604052815 ) ) ;
#23567=CARTESIAN_POINT ( 'NONE',  ( 13.12592325053682174, 31.71798720882053502, -4.999999999999997335 ) ) ;
#23568=ORIENTED_EDGE ( 'NONE', *, *, #31640, .T. ) ;
#23571=AXIS2_PLACEMENT_3D ( 'NONE', #28709, #7576, #887 ) ;
#23572=CARTESIAN_POINT ( 'NONE',  ( 12.28942040934312985, -21.45707787718824733, -18.40523778129498567 ) ) ;
#23575=CARTESIAN_POINT ( 'NONE',  ( -15.17240177202555529, 26.28854900485869450, -8.297591635734974602 ) ) ;
#23578=CARTESIAN_POINT ( 'NONE',  ( 8.917746432365776244, -18.50716487789387088, -28.72979828505872746 ) ) ;
#23582=CARTESIAN_POINT ( 'NONE',  ( -8.544825274508923485, 21.36057392928206511, -22.27686155045734751 ) ) ;
#23587=CARTESIAN_POINT ( 'NONE',  ( -22.05567186454189255, -3.361187274895892418, -23.39584885048158114 ) ) ;
#23590=CARTESIAN_POINT ( 'NONE',  ( 28.29240262143307660, 0.1985313112800510538, -12.55298984254547534 ) ) ;
#23595=CARTESIAN_POINT ( 'NONE',  ( -28.87100298341330529, 0.1244608980665242309, -11.59986624588286652 ) ) ;
#23598=CARTESIAN_POINT ( 'NONE',  ( 34.31080765618935402, -5.232520982112594865, -5.000000000000004441 ) ) ;
#23604=DIRECTION ( 'NONE',  ( -0.000000000000000000, -0.000000000000000000, 1.000000000000000000 ) ) ;
#23612=CARTESIAN_POINT ( 'NONE',  ( 5.775113167322606600, 35.08353508384845298, -10.20345263113499890 ) ) ;
#23616=CARTESIAN_POINT ( 'NONE',  ( 19.79884881832018806, -27.24719281008185590, -5.000000000000007994 ) ) ;
#23621=CARTESIAN_POINT ( 'NONE',  ( 11.81796877063049855, 19.46134122272024669, -21.60282401223847515 ) ) ;
#23623=CARTESIAN_POINT ( 'NONE',  ( -14.50388987035031896, 23.93725455160438997, -12.57114492812263329 ) ) ;
#23626=CARTESIAN_POINT ( 'NONE',  ( 15.28593968016526539, 26.22478663915245889, -7.828761890089739772 ) ) ;
#23628=CARTESIAN_POINT ( 'NONE',  ( 32.51966212229606867, -20.60195123665384287, -5.435513030541969215 ) ) ;
#23630=CARTESIAN_POINT ( 'NONE',  ( -11.17525274941712965, 18.69957113221303757, -23.80519623910948823 ) ) ;
#23632=CARTESIAN_POINT ( 'NONE',  ( -10.57413422691279159, -17.73442412422751246, -28.02013674793951026 ) ) ;
#23636=CARTESIAN_POINT ( 'NONE',  ( -35.49576857290053766, -12.23958519446773785, -5.439352978075872258 ) ) ;
#23637=CARTESIAN_POINT ( 'NONE',  ( -12.84450433006265690, -23.57826165373034399, -14.50520116907959434 ) ) ;
#23639=CARTESIAN_POINT ( 'NONE',  ( 20.36878409817081703, 2.417852450439661460, -29.99999999999999289 ) ) ;
#23644=CARTESIAN_POINT ( 'NONE',  ( -23.38024468256067578, 0.3787364488140903540, -20.51809825364033202 ) ) ;
#23645=CARTESIAN_POINT ( 'NONE',  ( 21.35776115567573896, 0.1272554325118729346, -24.94344375846707607 ) ) ;
#23650=CARTESIAN_POINT ( 'NONE',  ( -22.28349864444602701, 2.069094159404865518, -21.78945192521086938 ) ) ;
#23652=CARTESIAN_POINT ( 'NONE',  ( 11.10756861982301125, 19.59949212537556562, -20.90349153980999475 ) ) ;
#23660=CARTESIAN_POINT ( 'NONE',  ( -26.20904522235016287, 5.310845850833655568, -5.000000000000001776 ) ) ;
#23664=CARTESIAN_POINT ( 'NONE',  ( 26.21722217325281079, -25.61866019997112076, -6.304309572116824967 ) ) ;
#23667=CARTESIAN_POINT ( 'NONE',  ( 14.90256438169874365, 26.33380216902334325, -9.220340838230743685 ) ) ;
#23669=VERTEX_POINT ( 'NONE', #25975 ) ;
#23670=CARTESIAN_POINT ( 'NONE',  ( -16.99205359343081057, 21.87216257061389157, -5.000000000000000888 ) ) ;
#23673=CARTESIAN_POINT ( 'NONE',  ( 10.99973294177321215, 17.29901363094238675, -29.34868498375898227 ) ) ;
#23677=CARTESIAN_POINT ( 'NONE',  ( -10.95797138140908089, 17.47870688081035340, -28.07251611394456603 ) ) ;
#23679=CARTESIAN_POINT ( 'NONE',  ( -15.50788136758524871, -26.74767648567673817, -5.000000000000000888 ) ) ;
#23682=CARTESIAN_POINT ( 'NONE',  ( -32.89506354292129231, -17.22296157212681322, -8.845019317189917629 ) ) ;
#23683=CARTESIAN_POINT ( 'NONE',  ( -9.128838725168229473, -25.12525415319764477, -8.353599142830312019 ) ) ;
#23684=CARTESIAN_POINT ( 'NONE',  ( 11.87583182831933293, 17.23919556405288844, -26.29577713834995834 ) ) ;
#23686=CARTESIAN_POINT ( 'NONE',  ( 23.88329450473187165, 7.269808345019653117, -10.83961925935574122 ) ) ;
#23692=CARTESIAN_POINT ( 'NONE',  ( -31.99486564968922409, -1.644587291267736617, -7.306215044918229040 ) ) ;
#23694=CARTESIAN_POINT ( 'NONE',  ( 20.69502533546467049, 0.8251162403339853402, -27.44695267912525694 ) ) ;
#23707=CARTESIAN_POINT ( 'NONE',  ( 0.4114189264675339741, 38.49512827994399800, -5.000000000000003553 ) ) ;
#23716=CARTESIAN_POINT ( 'NONE',  ( 11.15866139110228161, 21.00416962748823480, -20.35793133617824680 ) ) ;
#23720=CARTESIAN_POINT ( 'NONE',  ( -17.86741215881691858, 13.84986514057024287, -17.98417663591535032 ) ) ;
#23723=CARTESIAN_POINT ( 'NONE',  ( 9.723126879071481099, -18.42578174174817462, -26.82764559573607599 ) ) ;
#23725=CARTESIAN_POINT ( 'NONE',  ( 10.96431188987212479, 17.32148673788787718, -29.34792031095122056 ) ) ;
#23728=CARTESIAN_POINT ( 'NONE',  ( -15.95643642716439814, -14.97217458464374218, -24.37019123110221130 ) ) ;
#23729=CARTESIAN_POINT ( 'NONE',  ( 2.749517794474013233, -20.36689819698734993, -29.42597746536911885 ) ) ;
#23730=CARTESIAN_POINT ( 'NONE',  ( 14.43692155601393523, 24.10478420696655633, -12.56460344322019118 ) ) ;
#23731=CARTESIAN_POINT ( 'NONE',  ( 19.13270401218881389, 10.69174942926454364, -20.12447810330580822 ) ) ;
#23734=CARTESIAN_POINT ( 'NONE',  ( -5.927024997082391167, 29.01444388681059294, -15.76666309069987904 ) ) ;
#23743=CARTESIAN_POINT ( 'NONE',  ( -24.46827507224332976, 0.6227895819650135500, -18.47284972081245158 ) ) ;
#23745=CARTESIAN_POINT ( 'NONE',  ( 30.96083639235021678, -10.32297208420813384, -12.95559803073687277 ) ) ;
#23761=CARTESIAN_POINT ( 'NONE',  ( 17.77173691806767764, 16.90998488025378421, -12.82112725625904659 ) ) ;
#23762=CARTESIAN_POINT ( 'NONE',  ( 13.08272806821811685, 31.59167807745777523, -6.349128532506149725 ) ) ;
#23766=CARTESIAN_POINT ( 'NONE',  ( 15.50750456237632235, -26.45556754333551552, -7.819482178144383511 ) ) ;
#23770=CARTESIAN_POINT ( 'NONE',  ( -15.39383690649032488, 26.76996700796825479, -5.945875866430524681 ) ) ;
#23773=CARTESIAN_POINT ( 'NONE',  ( 14.00981168397869325, -26.01563153178782528, -8.306567882437748906 ) ) ;
#23778=CARTESIAN_POINT ( 'NONE',  ( -11.25898764560963272, 28.46192956650065753, -13.15053914888870956 ) ) ;
#23783=ORIENTED_EDGE ( 'NONE', *, *, #355, .T. ) ;
#23784=CARTESIAN_POINT ( 'NONE',  ( 20.69061391627001711, 0.8884056894011840289, -27.45102547293791417 ) ) ;
#23790=CARTESIAN_POINT ( 'NONE',  ( -25.84690816252402357, 0.3462692498223990945, -16.44622743198997483 ) ) ;
#23793=CARTESIAN_POINT ( 'NONE',  ( 23.46557895267442362, -3.401122285006365153, -21.14145122161913548 ) ) ;
#23799=DIRECTION ( 'NONE',  ( 0.000000000000000000, 0.000000000000000000, 1.000000000000000000 ) ) ;
#23809=CARTESIAN_POINT ( 'NONE',  ( 3.962059598754420708, 20.50340585479708011, -27.03137393839747560 ) ) ;
#23812=CARTESIAN_POINT ( 'NONE',  ( 12.39337453381797616, -17.63539129962619967, -24.72786391051304378 ) ) ;
#23815=FACE_BOUND ( 'NONE', #12304, .T. ) ;
#23817=CARTESIAN_POINT ( 'NONE',  ( 10.91660561822348896, 17.40535124426578761, -28.70322919763274783 ) ) ;
#23819=CARTESIAN_POINT ( 'NONE',  ( -11.77357070864453092, 18.18633671150151443, -23.89743119366780633 ) ) ;
#23822=CARTESIAN_POINT ( 'NONE',  ( 14.57902638507616366, 24.84342498027717383, -11.60275616826175948 ) ) ;
#23824=CARTESIAN_POINT ( 'NONE',  ( 31.14704341106911656, -19.74704749676938675, -9.282700252451727252 ) ) ;
#23826=CARTESIAN_POINT ( 'NONE',  ( -14.95020005163037702, 26.98781491602204952, -8.271018971934079644 ) ) ;
#23828=CARTESIAN_POINT ( 'NONE',  ( -18.24387349984239037, -27.08452756295628205, -6.833357348710000778 ) ) ;
#23834=CARTESIAN_POINT ( 'NONE',  ( -19.25070363287986197, -7.311498989063264453, -28.46895897768014905 ) ) ;
#23835=CARTESIAN_POINT ( 'NONE',  ( -9.241419177041928279, -18.43513586380258573, -28.09520835628508095 ) ) ;
#23838=CARTESIAN_POINT ( 'NONE',  ( 27.69967049059682296, 2.038585896039051271, -10.70918416779063165 ) ) ;
#23844=CARTESIAN_POINT ( 'NONE',  ( -20.48527248842334458, 0.7769947089114559446, -29.34686795096567380 ) ) ;
#23845=CARTESIAN_POINT ( 'NONE',  ( 32.07997776912482379, -1.415336196370684529, -5.928950972838648248 ) ) ;
#23849=CARTESIAN_POINT ( 'NONE',  ( -25.95428780700007820, 2.674197598944707099, -13.64957008435976960 ) ) ;
#23850=CARTESIAN_POINT ( 'NONE',  ( 12.05832241004688399, 18.99596958976722760, -21.04195414767209726 ) ) ;
#23859=CARTESIAN_POINT ( 'NONE',  ( -19.97087465710904652, 5.004486353843795143, -28.23393442912554008 ) ) ;
#23862=CARTESIAN_POINT ( 'NONE',  ( 22.07789268346514433, -22.99653480363242153, -13.02319493230320724 ) ) ;
#23866=CARTESIAN_POINT ( 'NONE',  ( 14.11939125880675938, 24.91404824547022301, -12.51327720378664310 ) ) ;
#23870=CARTESIAN_POINT ( 'NONE',  ( -13.97090665946301336, 15.18147329247454280, -27.63196484367346883 ) ) ;
#23873=CARTESIAN_POINT ( 'NONE',  ( 15.38381738949339272, 26.63070857578979300, -6.417047948954210490 ) ) ;
#23875=CARTESIAN_POINT ( 'NONE',  ( 11.89393184209720111, 19.38028970819424757, -21.61737904418153988 ) ) ;
#23877=CARTESIAN_POINT ( 'NONE',  ( -13.15316605911461245, 22.33945200540117426, -16.43108139302208315 ) ) ;
#23879=CARTESIAN_POINT ( 'NONE',  ( -13.09026340579413628, -23.09710496079592446, -15.44275337101657186 ) ) ;
#23881=CARTESIAN_POINT ( 'NONE',  ( -32.00223536558479509, -16.75185194936180011, -10.17489710537347669 ) ) ;
#23882=CARTESIAN_POINT ( 'NONE',  ( -8.966847780561042924, -24.82021992796463294, -9.807061091129195773 ) ) ;
#23884=CARTESIAN_POINT ( 'NONE',  ( 12.15445636706326482, 17.84729731487952265, -23.95206648447458164 ) ) ;
#23886=CARTESIAN_POINT ( 'NONE',  ( 24.51742203815395982, 7.367698884986912056, -7.410464452778436240 ) ) ;
#23890=ORIENTED_EDGE ( 'NONE', *, *, #9638, .F. ) ;
#23891=CARTESIAN_POINT ( 'NONE',  ( -23.66820407423360351, -0.4863796308273267699, -20.40241117499521906 ) ) ;
#23893=CARTESIAN_POINT ( 'NONE',  ( 30.78377185402874971, -0.09069996828062186489, -6.886088703951912748 ) ) ;
#23898=AXIS2_PLACEMENT_3D ( 'NONE', #3113, #15700, #15509 ) ;
#23900=CYLINDRICAL_SURFACE ( 'NONE', #4366, 15.99999999999999645 ) ;
#23906=CARTESIAN_POINT ( 'NONE',  ( 0.4103210871597268716, 38.34576889810298894, -6.276193439666084117 ) ) ;
#23916=CARTESIAN_POINT ( 'NONE',  ( 9.842964772816607422, 17.98588232539188425, -29.32391334795786975 ) ) ;
#23920=CARTESIAN_POINT ( 'NONE',  ( -16.78989029355724583, 13.95002842669032006, -21.11808514744672749 ) ) ;
#23924=CARTESIAN_POINT ( 'NONE',  ( 15.20883357874183517, -26.29087852017448057, -8.296495227514824933 ) ) ;
#23926=CARTESIAN_POINT ( 'NONE',  ( 13.48758456246937065, 22.82324740036665744, -15.44989232396192236 ) ) ;
#23927=CARTESIAN_POINT ( 'NONE',  ( 12.12035967098243283, 19.93664080562797025, -20.53879709934572162 ) ) ;
#23929=CARTESIAN_POINT ( 'NONE',  ( -32.33143948542088708, 1.358872982498823268, -5.000000000000000888 ) ) ;
#23931=CARTESIAN_POINT ( 'NONE',  ( -27.24402026484078476, -22.73710829990762861, -10.20726825364095269 ) ) ;
#23932=CARTESIAN_POINT ( 'NONE',  ( 4.543046482400002972, -20.88912539285810155, -23.23170238819161426 ) ) ;
#23933=CARTESIAN_POINT ( 'NONE',  ( 12.80356091706831556, 20.83509046290971156, -18.47796576163459648 ) ) ;
#23934=CARTESIAN_POINT ( 'NONE',  ( 19.82717930584050947, 11.06638669728694602, -16.98486891981015390 ) ) ;
#23937=CARTESIAN_POINT ( 'NONE',  ( -6.355925524898499823, 36.92694055957776555, -6.714009213630858675 ) ) ;
#23946=CARTESIAN_POINT ( 'NONE',  ( -30.47170454527866923, 0.4016671284418433796, -4.999999999999999112 ) ) ;
#23947=CARTESIAN_POINT ( 'NONE',  ( 28.06320634686874627, -9.371851771698166189, -15.76881348996817067 ) ) ;
#23952=CARTESIAN_POINT ( 'NONE',  ( -35.48557158514988430, -11.25000000000002309, 10.00000000000000000 ) ) ;
#23964=CARTESIAN_POINT ( 'NONE',  ( 16.84224471403853229, 14.37780181299635984, -20.04792273672603997 ) ) ;
#23965=CARTESIAN_POINT ( 'NONE',  ( 9.502174681210730611, 24.54420635781409388, -17.97437483132709701 ) ) ;
#23967=CARTESIAN_POINT ( 'NONE',  ( -21.48623309969284989, 11.60342812567675885, -9.394375087043044914 ) ) ;
#23970=CARTESIAN_POINT ( 'NONE',  ( 10.09390139374666262, -18.42364844336855256, -26.19501470389041842 ) ) ;
#23972=CARTESIAN_POINT ( 'NONE',  ( 27.08779848459123585, 7.221796966026763798, -5.000000000000007105 ) ) ;
#23973=CARTESIAN_POINT ( 'NONE',  ( -12.92966971681751431, 21.65081211195085942, -17.43791612333144414 ) ) ;
#23975=CARTESIAN_POINT ( 'NONE',  ( -20.88456819748228810, -23.43278618219788711, -13.06947050431665858 ) ) ;
#23976=CARTESIAN_POINT ( 'NONE',  ( 13.62892564869307854, -25.43202621200122948, -10.20098705052232724 ) ) ;
#23981=CARTESIAN_POINT ( 'NONE',  ( -7.677290147211061289, 19.01944725762398392, -29.99999999999998934 ) ) ;
#23986=CARTESIAN_POINT ( 'NONE',  ( 28.27163672435500530, 0.2247573307824139721, -12.55420016491700608 ) ) ;
#23991=CARTESIAN_POINT ( 'NONE',  ( -22.21514529423838979, 0.6880714958666251935, -22.73802149961197472 ) ) ;
#23994=CARTESIAN_POINT ( 'NONE',  ( 33.42451262833972692, -5.048360147377955798, -8.566326254722081757 ) ) ;
#23999=CARTESIAN_POINT ( 'NONE',  ( 0.000000000000000000, 22.50000000000000355, 6.000000000000000000 ) ) ;
#24008=CARTESIAN_POINT ( 'NONE',  ( 6.458614852237183790, 33.04048157560279009, -12.02760640721125363 ) ) ;
#24012=CARTESIAN_POINT ( 'NONE',  ( 18.56734095888186786, -27.10473135465256433, -6.828420776304507278 ) ) ;
#24017=CARTESIAN_POINT ( 'NONE',  ( 12.86711912072691177, 21.75488451896397279, -17.42369386892843863 ) ) ;
#24019=CARTESIAN_POINT ( 'NONE',  ( -13.99681549934592084, 22.91249579894840949, -14.50524598184051150 ) ) ;
#24024=CARTESIAN_POINT ( 'NONE',  ( 15.22753785222040435, 26.10542462839032041, -8.299041287613635021 ) ) ;
#24026=CARTESIAN_POINT ( 'NONE',  ( 29.11864404320880340, -18.46465774631702672, -11.97498759040503913 ) ) ;
#24028=CARTESIAN_POINT ( 'NONE',  ( -11.54653377988851304, 19.74306190993011256, -21.55203727238154343 ) ) ;
#24029=FACE_OUTER_BOUND ( 'NONE', #29501, .T. ) ;
#24030=CARTESIAN_POINT ( 'NONE',  ( -11.33884614197604890, -19.32953085267849502, -22.62991861938991889 ) ) ;
#24033=CARTESIAN_POINT ( 'NONE',  ( -19.17275462598830060, -7.282501898908932958, -29.22487285613485852 ) ) ;
#24035=CARTESIAN_POINT ( 'NONE',  ( -14.56418105446348932, -25.61681370524265589, -10.18385066514556669 ) ) ;
#24038=CARTESIAN_POINT ( 'NONE',  ( 26.85566260921343584, 2.066112236289315174, -12.63869616061161061 ) ) ;
#24045=CARTESIAN_POINT ( 'NONE',  ( -20.48447659325206516, 0.7979435291051002466, -30.00000000000000000 ) ) ;
#24047=EDGE_CURVE ( 'NONE', #19728, #23375, #5110, .T. ) ;
#24048=CARTESIAN_POINT ( 'NONE',  ( 31.18558700419108831, -0.9481828064721339322, -8.253045886946059895 ) ) ;
#24051=CARTESIAN_POINT ( 'NONE',  ( -27.66981915501925826, 3.518264008085504546, -5.475398431093116081 ) ) ;
#24061=ORIENTED_EDGE ( 'NONE', *, *, #13311, .T. ) ;
#24062=CARTESIAN_POINT ( 'NONE',  ( -26.09954572027081454, 5.304898449170225128, -6.914248030060270445 ) ) ;
#24065=CARTESIAN_POINT ( 'NONE',  ( 24.71631120996009656, -24.23736600738799396, -10.25405846535409538 ) ) ;
#24067=CARTESIAN_POINT ( 'NONE',  ( 34.47241746879583957, 3.460351812918713854, 3.000000000000000000 ) ) ;
#24068=CARTESIAN_POINT ( 'NONE',  ( 10.70229295774111478, 17.48483442551455269, -29.34227022712989452 ) ) ;
#24071=CARTESIAN_POINT ( 'NONE',  ( -16.07951411908364392, 20.32485814370012633, -12.71120202138577504 ) ) ;
#24073=CARTESIAN_POINT ( 'NONE',  ( -36.48557158514989140, -11.24999999999987743, 10.00000000000000000 ) ) ;
#24074=CARTESIAN_POINT ( 'NONE',  ( 12.40954600831128296, 20.46600775631657854, -19.49970488155097215 ) ) ;
#24078=CARTESIAN_POINT ( 'NONE',  ( -11.40498260276712017, 18.50559946058070082, -23.84136616158568600 ) ) ;
#24080=CARTESIAN_POINT ( 'NONE',  ( -10.28329067726930113, -19.14409761816654054, -23.84654465020906500 ) ) ;
#24083=CARTESIAN_POINT ( 'NONE',  ( -25.36562297843122238, -14.28257506075462047, -16.62385786568234636 ) ) ;
#24084=CARTESIAN_POINT ( 'NONE',  ( -7.791008596474476633, -19.63400282832837362, -25.23920589239619261 ) ) ;
#24086=CARTESIAN_POINT ( 'NONE',  ( 11.84859450830439442, 16.77681853612139662, -28.74023605449830399 ) ) ;
#24088=CARTESIAN_POINT ( 'NONE',  ( 19.48206314129080141, 6.618909439000534967, -28.26876915201039964 ) ) ;
#24094=CARTESIAN_POINT ( 'NONE',  ( -20.64734822606397913, -0.1544862121781659936, -28.02694178585644735 ) ) ;
#24095=CARTESIAN_POINT ( 'NONE',  ( 29.95060329414361533, -0.1183784304507303486, -9.698056910375742135 ) ) ;
#24099=CARTESIAN_POINT ( 'NONE',  ( 35.36940577612500647, -20.42053594592275800, -14.51648065752882566 ) ) ;
#24106=CARTESIAN_POINT ( 'NONE',  ( 1.465318874961157203, 35.37165157456092857, -11.06833281905744570 ) ) ;
#24114=CARTESIAN_POINT ( 'NONE',  ( 14.38792334706498899, 28.09311145835767221, -8.686077744534234313 ) ) ;
#24117=CARTESIAN_POINT ( 'NONE',  ( -18.91572163234467041, 16.32661989365160338, -9.372685314759676700 ) ) ;
#24121=CARTESIAN_POINT ( 'NONE',  ( 15.30940322879717286, -26.50162545292337057, -7.357895834298116888 ) ) ;
#24123=CARTESIAN_POINT ( 'NONE',  ( 14.92592191758538434, 25.82844783702134350, -9.707335997509764169 ) ) ;
#24127=CARTESIAN_POINT ( 'NONE',  ( -16.46786645114412551, -12.86135933887615579, -27.00130938684783999 ) ) ;
#24128=CARTESIAN_POINT ( 'NONE',  ( 3.891635163620496662, -24.39404397995950546, -9.874836895460536113 ) ) ;
#24129=CARTESIAN_POINT ( 'NONE',  ( 11.28285220518144172, 17.35954613783441758, -27.46386206762080207 ) ) ;
#24130=CARTESIAN_POINT ( 'NONE',  ( 20.72356761093054089, 11.55030529434603181, -12.89082050402462976 ) ) ;
#24132=CARTESIAN_POINT ( 'NONE',  ( -4.317981579255198987, 25.11931188802156711, -19.71681041348662333 ) ) ;
#24138=ADVANCED_FACE ( 'NONE', ( #30841, #24542 ), #3007, .T. ) ;
#24140=CARTESIAN_POINT ( 'NONE',  ( -25.13567556507226897, 0.5201041552294234371, -17.45255897844877069 ) ) ;
#24141=CARTESIAN_POINT ( 'NONE',  ( 20.44673976918552327, -6.181689145942012686, -25.69967426495654905 ) ) ;
#24145=DIRECTION ( 'NONE',  ( -1.000000000000000000, 0.000000000000000000, 0.000000000000000000 ) ) ;
#24157=CARTESIAN_POINT ( 'NONE',  ( 26.90452307301082158, -22.05113920026022356, -11.10173837139930697 ) ) ;
#24158=CARTESIAN_POINT ( 'NONE',  ( 17.72686569301070492, 14.07852954895453479, -17.97737483715281570 ) ) ;
#24159=CARTESIAN_POINT ( 'NONE',  ( 7.566615708652627781, 19.25748430301096192, -27.88712974580454329 ) ) ;
#24161=CARTESIAN_POINT ( 'NONE',  ( -19.21278935434771995, 9.517384517114377829, -22.24295473033291515 ) ) ;
#24167=CARTESIAN_POINT ( 'NONE',  ( 14.83614609751987423, -25.15722166327546105, -11.56489435687942802 ) ) ;
#24170=CARTESIAN_POINT ( 'NONE',  ( -14.27227629280091215, 24.52115250329153540, -12.54634419364836262 ) ) ;
#24171=CARTESIAN_POINT ( 'NONE',  ( -17.64560943446032937, -21.02421742741433164, -16.93458103129471226 ) ) ;
#24172=CARTESIAN_POINT ( 'NONE',  ( 13.69821889811312410, -26.30560278297641830, -5.000000000000000000 ) ) ;
#24177=CARTESIAN_POINT ( 'NONE',  ( -7.081591661052614839, 19.23835092891137322, -29.27181413004323929 ) ) ;
#24183=CARTESIAN_POINT ( 'NONE',  ( 29.75086405456110938, 0.1002501869623030895, -9.710278012872217701 ) ) ;
#24187=CARTESIAN_POINT ( 'NONE',  ( -25.85423149439973400, 0.3339084734886691441, -16.44513718936062929 ) ) ;
#24191=CARTESIAN_POINT ( 'NONE',  ( 25.82646452138326154, -3.017894876147785510, -18.05725647810044521 ) ) ;
#24204=CARTESIAN_POINT ( 'NONE',  ( 7.399002019425528154, 32.59854033243159677, -12.04523620305728393 ) ) ;
#24210=CARTESIAN_POINT ( 'NONE',  ( 12.31336357260648562, -16.48320293064839959, -28.59255635963331699 ) ) ;
#24212=FACE_BOUND ( 'NONE', #32795, .T. ) ;
#24215=CARTESIAN_POINT ( 'NONE',  ( 15.26368502715787656, 26.62251295125168582, -7.355208640532818976 ) ) ;
#24217=CARTESIAN_POINT ( 'NONE',  ( -12.79441350932495780, 20.84820608835214983, -18.47654784684910112 ) ) ;
#24218=AXIS2_PLACEMENT_3D ( 'NONE', #37496, #5612, #34053 ) ;
#24220=CARTESIAN_POINT ( 'NONE',  ( 10.48966746473434064, -19.58931170878575756, -22.74071033439049572 ) ) ;
#24222=CARTESIAN_POINT ( 'NONE',  ( 14.07857810331197257, 23.82131834651897861, -13.51868220414109700 ) ) ;
#24224=CARTESIAN_POINT ( 'NONE',  ( 26.47194016310583820, -16.78111321318651861, -14.73213283222064796 ) ) ;
#24226=CARTESIAN_POINT ( 'NONE',  ( -13.82211424505259778, 24.42565547601927634, -13.46747677272994004 ) ) ;
#24228=CARTESIAN_POINT ( 'NONE',  ( -14.47914568234718224, -23.13007937158521088, -15.30831667679490415 ) ) ;
#24229=CARTESIAN_POINT ( 'NONE',  ( -16.84920187510344647, 29.09530251743286300, -5.000000000000000000 ) ) ;
#24232=CARTESIAN_POINT ( 'NONE',  ( -32.70405218813849757, -11.20998461038165495, -11.11490927511992410 ) ) ;
#24233=CARTESIAN_POINT ( 'NONE',  ( -15.12763912169749858, -26.45704430479512936, -7.358536573642846967 ) ) ;
#24236=CARTESIAN_POINT ( 'NONE',  ( 20.62929968266412928, 3.093903264742920101, -26.39664856447400965 ) ) ;
#24238=AXIS2_PLACEMENT_3D ( 'NONE', #4469, #10767, #25593 ) ;
#24241=CARTESIAN_POINT ( 'NONE',  ( -26.55369869109904357, 0.2031603616629021614, -15.44166204089604832 ) ) ;
#24244=CARTESIAN_POINT ( 'NONE',  ( 21.82419164594113070, 0.07435039598037769537, -23.77433660182619946 ) ) ;
#24249=CARTESIAN_POINT ( 'NONE',  ( -27.21597387510395194, 2.648795058466725916, -10.72652230008515772 ) ) ;
#24259=CARTESIAN_POINT ( 'NONE',  ( -24.20609638677606412, 8.035638068618503382, -5.480463713371170442 ) ) ;
#24262=CARTESIAN_POINT ( 'NONE',  ( 25.11666564602450791, -26.04266884310358421, -6.744201284302634214 ) ) ;
#24266=CARTESIAN_POINT ( 'NONE',  ( 15.34186426957387184, 27.04214388478009923, -5.472936367007620539 ) ) ;
#24270=CARTESIAN_POINT ( 'NONE',  ( -13.90277657046047288, 15.06583648262319031, -29.40017519746768926 ) ) ;
#24273=CARTESIAN_POINT ( 'NONE',  ( 11.09010279485205963, 17.49098561682555442, -27.44912391568058041 ) ) ;
#24277=CARTESIAN_POINT ( 'NONE',  ( -10.90492496769149433, 17.35893878472046126, -29.99999999999998934 ) ) ;
#24279=CARTESIAN_POINT ( 'NONE',  ( -10.24267276777706215, -19.15822127202351055, -23.85172878415961506 ) ) ;
#24281=CARTESIAN_POINT ( 'NONE',  ( -26.74262847843787938, -14.00387254376185453, -15.68192966552173928 ) ) ;
#24283=CARTESIAN_POINT ( 'NONE',  ( -9.368301651731773205, -22.13363141439098314, -17.67998840172026576 ) ) ;
#24285=CARTESIAN_POINT ( 'NONE',  ( 14.37559196849546161, 21.13036632534599235, -15.57174267854623473 ) ) ;
#24287=CARTESIAN_POINT ( 'NONE',  ( 22.56375456310565042, 6.182170930846935697, -16.85945526150993956 ) ) ;
#24292=CARTESIAN_POINT ( 'NONE',  ( -21.92138948956064581, -0.6339311634017230634, -23.68985892038928398 ) ) ;
#24293=ADVANCED_FACE ( 'NONE', ( #10704 ), #13136, .T. ) ;
#24295=CARTESIAN_POINT ( 'NONE',  ( 20.48413544616686011, 0.8063757131868728445, -30.00000000000000000 ) ) ;
#24299=CARTESIAN_POINT ( 'NONE',  ( 12.05832241004688399, 18.99596958976722760, -21.04195414767209726 ) ) ;
#24306=DIRECTION ( 'NONE',  ( 1.000000000000000000, 0.000000000000000000, 0.000000000000000000 ) ) ;
#24307=CARTESIAN_POINT ( 'NONE',  ( 3.860467995676855502, 37.87601681638416551, -6.280638966725057948 ) ) ;
#24317=CARTESIAN_POINT ( 'NONE',  ( 14.90467518106525269, 28.31725849260483585, -4.999999999999998224 ) ) ;
#24320=CARTESIAN_POINT ( 'NONE',  ( -17.38933059521489710, 14.62580955216105849, -17.95874418599646560 ) ) ;
#24323=CARTESIAN_POINT ( 'NONE',  ( 13.02171807787146385, -23.09221996238842323, -15.44989160518525928 ) ) ;
#24324=CARTESIAN_POINT ( 'NONE',  ( -13.76749719093327329, -17.52493337752909142, -23.41495867390861818 ) ) ;
#24325=DIRECTION ( 'NONE',  ( 1.000000000000000000, 0.000000000000000000, 0.000000000000000000 ) ) ;
#24326=CARTESIAN_POINT ( 'NONE',  ( 11.45955615606448319, 18.45868997252334864, -23.85003837067463550 ) ) ;
#24327=ORIENTED_EDGE ( 'NONE', *, *, #30446, .T. ) ;
#24332=CARTESIAN_POINT ( 'NONE',  ( -23.53733200146751869, -18.44805065072479877, -15.72207550959232947 ) ) ;
#24333=CARTESIAN_POINT ( 'NONE',  ( -0.2650373451695003379, -20.49916026595607121, -30.00000000000000711 ) ) ;
#24334=CARTESIAN_POINT ( 'NONE',  ( 14.92415143525127341, 24.85911683587750787, -10.66521362572363785 ) ) ;
#24335=CARTESIAN_POINT ( 'NONE',  ( 22.21982769557913784, 11.10346373912405049, -4.999999999999997335 ) ) ;
#24337=CARTESIAN_POINT ( 'NONE',  ( -4.208561989267932901, 37.92874393496560970, -5.858868913340946172 ) ) ;
#24339=CARTESIAN_POINT ( 'NONE',  ( -33.77851027019138286, -5.369403031741126320, -8.110867528180607522 ) ) ;
#24345=CARTESIAN_POINT ( 'NONE',  ( -21.68533774883767862, 0.8527267334164467805, -23.86863619998306518 ) ) ;
#24346=CARTESIAN_POINT ( 'NONE',  ( 34.54137992947591584, -13.89200096410145768, -7.989112350646218275 ) ) ;
#24355=VECTOR ( 'NONE', #33396, 1000.000000000000000 ) ;
#24357=ORIENTED_EDGE ( 'NONE', *, *, #8197, .F. ) ;
#24361=CARTESIAN_POINT ( 'NONE',  ( 30.18422347142476880, -23.20414393450525736, -5.000000000000001776 ) ) ;
#24362=CARTESIAN_POINT ( 'NONE',  ( 19.54635772746084399, 15.94078878846792335, -5.481359321442739407 ) ) ;
#24363=CARTESIAN_POINT ( 'NONE',  ( 7.501377273760488684, 19.07882637373012713, -29.27881224950820283 ) ) ;
#24365=CARTESIAN_POINT ( 'NONE',  ( -21.95856242959800042, 10.64870207983313577, -9.886801507649353837 ) ) ;
#24367=CARTESIAN_POINT ( 'NONE',  ( 15.05947082473196197, -25.87448528531247760, -9.699063484119998080 ) ) ;
#24369=EDGE_CURVE ( 'NONE', #32508, #20904, #20694, .T. ) ;
#24370=CARTESIAN_POINT ( 'NONE',  ( 23.06249103411542478, 13.31513540672987972, -4.999999999999992006 ) ) ;
#24372=CARTESIAN_POINT ( 'NONE',  ( -11.01071465375284752, 17.44424455191658296, -28.07566285216567081 ) ) ;
#24373=CARTESIAN_POINT ( 'NONE',  ( -15.32667431977992578, -18.29772241814856670, -21.07163874326107589 ) ) ;
#24374=CARTESIAN_POINT ( 'NONE',  ( 8.268557591513960858, -18.75831942629880444, -30.00000000000000000 ) ) ;
#24378=CARTESIAN_POINT ( 'NONE',  ( -8.856483827409315168, 29.59330869415324372, -13.96223684641979901 ) ) ;
#24380=DIRECTION ( 'NONE',  ( -1.000000000000000000, 0.000000000000000000, 0.000000000000000000 ) ) ;
#24386=CARTESIAN_POINT ( 'NONE',  ( 23.93473260754475618, 0.4999434715730360357, -19.49809802192611841 ) ) ;
#24390=CARTESIAN_POINT ( 'NONE',  ( -30.85287573504917802, -0.02542951706361920583, -5.946081676602823940 ) ) ;
#24393=CARTESIAN_POINT ( 'NONE',  ( 32.36939943392307129, -4.852295849567697772, -10.37643807136409890 ) ) ;
#24396=ADVANCED_FACE ( 'NONE', ( #39734 ), #23900, .F. ) ;
#24405=CARTESIAN_POINT ( 'NONE',  ( 3.293556582578045067, 20.32739358238259442, -28.46901180915632779 ) ) ;
#24411=CARTESIAN_POINT ( 'NONE',  ( 12.13886791120663489, -18.39813430154476492, -23.60940752486453675 ) ) ;
#24417=CARTESIAN_POINT ( 'NONE',  ( -11.14607843802444087, 17.59829798962171310, -26.83237680307435369 ) ) ;
#24419=CARTESIAN_POINT ( 'NONE',  ( 14.64890392409851572, -25.63402876358651383, -10.18232085067979220 ) ) ;
#24425=CARTESIAN_POINT ( 'NONE',  ( -13.39899704888391518, 25.36066129426254534, -13.38256906110033029 ) ) ;
#24427=CARTESIAN_POINT ( 'NONE',  ( -11.14796620122417536, -17.40538162519350252, -27.98683963314264034 ) ) ;
#24430=CARTESIAN_POINT ( 'NONE',  ( -34.29392370955937963, -11.77843072186552220, -8.881902778450617930 ) ) ;
#24431=CARTESIAN_POINT ( 'NONE',  ( -14.04164913135559978, -25.01591397610629031, -11.60796646869975390 ) ) ;
#24434=CARTESIAN_POINT ( 'NONE',  ( 21.24802458993929832, 0.9742268056361320649, -25.03556984149153308 ) ) ;
#24438=CARTESIAN_POINT ( 'NONE',  ( -28.97168722745774261, 0.006711083214636500045, -11.59031396894388699 ) ) ;
#24440=CARTESIAN_POINT ( 'NONE',  ( 24.20991175986098654, -0.1716401066519940843, -19.40784505169473206 ) ) ;
#24445=CARTESIAN_POINT ( 'NONE',  ( -20.46803965419261218, 2.897456671940229711, -27.56527374437133204 ) ) ;
#24454=CARTESIAN_POINT ( 'NONE',  ( -19.71604245095232955, 5.704143033173037836, -28.82764346654152732 ) ) ;
#24457=CARTESIAN_POINT ( 'NONE',  ( 22.12641700133371359, -25.78554156883743431, -9.427553252327385280 ) ) ;
#24460=CARTESIAN_POINT ( 'NONE',  ( 13.65407654052588526, 23.65245025108414367, -14.44949798609442126 ) ) ;
#24464=CARTESIAN_POINT ( 'NONE',  ( -16.20952767024093077, 24.08095879529154004, -5.947967261773682957 ) ) ;
#24467=CARTESIAN_POINT ( 'NONE',  ( 11.09448639774211287, 17.48802892231923778, -27.44946313874878996 ) ) ;
#24472=CARTESIAN_POINT ( 'NONE',  ( -12.87226721047317035, 21.74635154274772120, -17.42485855766595648 ) ) ;
#24474=CARTESIAN_POINT ( 'NONE',  ( -12.44633464221259622, -22.01977715156473536, -17.41908692410127912 ) ) ;
#24477=CARTESIAN_POINT ( 'NONE',  ( -32.42739033151597283, -18.25660761601222148, -8.842418814747594169 ) ) ;
#24478=CARTESIAN_POINT ( 'NONE',  ( -11.50551555847164664, -25.70084177611234466, -6.898850981578088515 ) ) ;
#24480=CARTESIAN_POINT ( 'NONE',  ( 16.11351922548164950, 24.44051152376729519, -5.474194937227850666 ) ) ;
#24482=CARTESIAN_POINT ( 'NONE',  ( 20.28232154407063348, 6.728145097213812598, -23.24529083297425558 ) ) ;
#24487=CARTESIAN_POINT ( 'NONE',  ( -21.88088975564236449, -0.2942360282749391653, -23.72980161136129240 ) ) ;
#24488=CARTESIAN_POINT ( 'NONE',  ( 25.24508218390874603, 0.3179225735388317431, -17.43064974027972980 ) ) ;
#24502=CARTESIAN_POINT ( 'NONE',  ( 3.060806728840579805, 29.89625055151331168, -15.70096931457847234 ) ) ;
#24509=DIRECTION ( 'NONE',  ( 0.000000000000000000, 0.000000000000000000, 1.000000000000000000 ) ) ;
#24510=CARTESIAN_POINT ( 'NONE',  ( 13.56443329977971857, 24.98013321944925735, -13.41769806874402171 ) ) ;
#24513=CARTESIAN_POINT ( 'NONE',  ( -16.42692940787602751, 16.16190383186714996, -17.88839106487290209 ) ) ;
#24517=CARTESIAN_POINT ( 'NONE',  ( 13.03491049794189216, -23.09316184486432277, -15.44851748533687008 ) ) ;
#24518=CARTESIAN_POINT ( 'NONE',  ( -16.05099854162948603, -21.51520587089331471, -17.05908743538380890 ) ) ;
#24519=FACE_OUTER_BOUND ( 'NONE', #10965, .T. ) ;
#24520=CARTESIAN_POINT ( 'NONE',  ( 14.52648563089041645, 24.98748751028934834, -11.59782509437098419 ) ) ;
#24526=CIRCLE ( 'NONE', #20618, 22.50000000000000355 ) ;
#24529=CARTESIAN_POINT ( 'NONE',  ( -29.02322137993849438, -24.14915179229603837, -5.438517818996884579 ) ) ;
#24530=CARTESIAN_POINT ( 'NONE',  ( -0.2994915553838167210, -21.65328977690111145, -21.17874425746205702 ) ) ;
#24531=CARTESIAN_POINT ( 'NONE',  ( 13.49234167325138145, 21.73580331833325019, -16.48722854393279391 ) ) ;
#24532=CARTESIAN_POINT ( 'NONE',  ( 20.40580192547206551, 12.55472529160778983, -11.88336945610312689 ) ) ;
#24535=CARTESIAN_POINT ( 'NONE',  ( -5.286117828675410024, 37.24231109432135867, -7.131154415093411636 ) ) ;
#24538=CARTESIAN_POINT ( 'NONE',  ( -28.89557855833852074, -5.358265633141725992, -14.97716460387147919 ) ) ;
#24542=FACE_OUTER_BOUND ( 'NONE', #22879, .T. ) ;
#24545=CARTESIAN_POINT ( 'NONE',  ( -29.58401177971029838, 0.6647329222074543909, -8.776217634601312767 ) ) ;
#24547=CARTESIAN_POINT ( 'NONE',  ( 34.31971835247910718, -13.79709225594373834, -8.423480077211841888 ) ) ;
#24558=CARTESIAN_POINT ( 'NONE',  ( -4.066748194678229567, 36.38340522611666472, -9.294197595149157110 ) ) ;
#24559=CARTESIAN_POINT ( 'NONE',  ( -20.23296131041716706, 28.12381335138030636, 0.000000000000000000 ) ) ;
#24563=CARTESIAN_POINT ( 'NONE',  ( 16.64356867624101000, -11.98442300389733717, -30.00000000000002487 ) ) ;
#24565=CARTESIAN_POINT ( 'NONE',  ( 19.45606358795933843, 15.84753467433722562, -7.419582043610376765 ) ) ;
#24566=CARTESIAN_POINT ( 'NONE',  ( 13.33950791723536611, 29.76583335417164733, -9.070794986034909968 ) ) ;
#24568=CARTESIAN_POINT ( 'NONE',  ( -20.17546868353657885, 9.912285996584582648, -18.01224743220988955 ) ) ;
#24571=CARTESIAN_POINT ( 'NONE',  ( 13.18019970074355385, -23.10295469650971256, -15.43347796454282062 ) ) ;
#24573=CARTESIAN_POINT ( 'NONE',  ( -16.77267017469753085, -29.13948811618693924, -13.79123840944732748 ) ) ;
#24574=CARTESIAN_POINT ( 'NONE',  ( -14.72251014768929167, 25.44185296451583866, -10.65018569441744134 ) ) ;
#24575=CARTESIAN_POINT ( 'NONE',  ( -18.83446081530439642, -22.42967529457653342, -14.99109861493270834 ) ) ;
#24576=CARTESIAN_POINT ( 'NONE',  ( 11.67685997438431045, -23.90497018467267765, -13.60458191810863049 ) ) ;
#24580=CARTESIAN_POINT ( 'NONE',  ( -8.116341641279710473, 24.50416309976997908, -18.90493885958451159 ) ) ;
#24587=CARTESIAN_POINT ( 'NONE',  ( 28.31319793978629917, 0.1723095648249480527, -12.55177946987335424 ) ) ;
#24589=DIRECTION ( 'NONE',  ( 1.000000000000000000, 0.000000000000000000, 0.000000000000000000 ) ) ;
#24593=CARTESIAN_POINT ( 'NONE',  ( -30.74133289564772298, 0.02125651492519025493, -6.417068207764520693 ) ) ;
#24596=CARTESIAN_POINT ( 'NONE',  ( 33.05307263222019287, -5.890996608547069080, -9.885471256058895761 ) ) ;
#24599=EDGE_CURVE ( 'NONE', #34935, #13116, #15426, .T. ) ;
#24609=CARTESIAN_POINT ( 'NONE',  ( 6.272699779124576658, 32.10004986042342523, -12.94969384604119433 ) ) ;
#24612=CARTESIAN_POINT ( 'NONE',  ( 17.27603859610683301, -25.39141712192287059, -11.41356120857962431 ) ) ;
#24618=CARTESIAN_POINT ( 'NONE',  ( -15.30065312247323028, 26.49437699940635937, -7.357947398261144301 ) ) ;
#24620=CARTESIAN_POINT ( 'NONE',  ( 13.92138958099786450, -24.59342578875250140, -12.55492369404029951 ) ) ;
#24624=CARTESIAN_POINT ( 'NONE',  ( -9.436104724621630524, 18.21145219648997227, -29.31522508094131751 ) ) ;
#24625=CARTESIAN_POINT ( 'NONE',  ( -20.57926088536441966, -27.21289976561331514, -4.999999999999997335 ) ) ;
#24626=CARTESIAN_POINT ( 'NONE',  ( -19.48557158514985588, -11.25000000000002309, 0.000000000000000000 ) ) ;
#24628=CARTESIAN_POINT ( 'NONE',  ( -28.18824097937255146, -7.837830145184667252, -15.82023872818571064 ) ) ;
#24629=CARTESIAN_POINT ( 'NONE',  ( -12.49708442935645358, -22.55589311136183284, -16.45579901909083276 ) ) ;
#24632=CARTESIAN_POINT ( 'NONE',  ( 20.47800464711415813, 1.727324350805305109, -28.73678694931549060 ) ) ;
#24636=CARTESIAN_POINT ( 'NONE',  ( -23.33365362593783487, 0.5068941057029301422, -20.53583360551006010 ) ) ;
#24638=CARTESIAN_POINT ( 'NONE',  ( 32.13235714270949472, -1.817784623349015360, -7.301148604131005193 ) ) ;
#24640=CARTESIAN_POINT ( 'NONE',  ( 4.811402195336492049, -19.97410447909037146, -30.00000000000001066 ) ) ;
#24644=CARTESIAN_POINT ( 'NONE',  ( -22.20364817425843285, 3.543267544546572889, -20.85647020598273471 ) ) ;
#24655=CARTESIAN_POINT ( 'NONE',  ( -23.77417876032645694, 7.953466752255449634, -9.369785356547680522 ) ) ;
#24658=CARTESIAN_POINT ( 'NONE',  ( 24.21359695930263101, -26.57684320323437532, -5.446510658207939670 ) ) ;
#24660=CARTESIAN_POINT ( 'NONE',  ( 12.51893876027292940, 21.25235172184055443, -18.42282389506313223 ) ) ;
#24662=CARTESIAN_POINT ( 'NONE',  ( -12.44972444764569453, 16.77980448052251106, -26.34956027326842687 ) ) ;
#24667=CARTESIAN_POINT ( 'NONE',  ( 11.91014968976024235, 19.36310277583015349, -21.62019219126923275 ) ) ;
#24669=CARTESIAN_POINT ( 'NONE',  ( -16.00000000000000000, 22.50000000000000355, 6.000000000000000000 ) ) ;
#24672=CARTESIAN_POINT ( 'NONE',  ( -15.30029427371034600, 27.09079015021717396, -5.942535154850186352 ) ) ;
#24674=CARTESIAN_POINT ( 'NONE',  ( -15.38607054502407756, -26.33262433206096986, -8.289753305509513837 ) ) ;
#24676=CARTESIAN_POINT ( 'NONE',  ( -31.78065895063095780, -15.41279462978935832, -11.07266024125810056 ) ) ;
#24677=CARTESIAN_POINT ( 'NONE',  ( -9.122435668794345531, -19.14094883146207593, -25.10522684686861439 ) ) ;
#24679=CARTESIAN_POINT ( 'NONE',  ( 13.13796970620712656, 19.50823006588858632, -19.62116264178829184 ) ) ;
#24681=CARTESIAN_POINT ( 'NONE',  ( 26.68456133973351641, 4.675186248811364464, -5.953666022845518491 ) ) ;
#24686=CARTESIAN_POINT ( 'NONE',  ( -20.55327584008562170, -0.1442271758602391429, -28.67149428179880744 ) ) ;
#24687=CARTESIAN_POINT ( 'NONE',  ( 29.17685817419758365, -0.2385013389979390996, -11.56797761538647329 ) ) ;
#24694=CARTESIAN_POINT ( 'NONE',  ( 27.08779848459123585, 7.221796966026769127, -13.42901749168596304 ) ) ;
#24701=CARTESIAN_POINT ( 'NONE',  ( 2.721668488675992759, 37.91170157744703317, -7.120364383801717878 ) ) ;
#24704=DIRECTION ( 'NONE',  ( 1.000000000000000000, 0.000000000000000000, 0.000000000000000000 ) ) ;
#24708=CARTESIAN_POINT ( 'NONE',  ( 10.18918489279338147, 17.95568076346413733, -28.02701222315408813 ) ) ;
#24711=CARTESIAN_POINT ( 'NONE',  ( -17.77270048994293106, 18.00536303972542029, -10.82195543332399978 ) ) ;
#24714=CARTESIAN_POINT ( 'NONE',  ( 9.504747149499191750, -18.16341882422712573, -29.34820719226206975 ) ) ;
#24716=CARTESIAN_POINT ( 'NONE',  ( -14.22557620116472421, -18.08049471867423819, -22.27683892693457679 ) ) ;
#24718=CARTESIAN_POINT ( 'NONE',  ( 14.01964074023701379, 23.95961702490197709, -13.51097757283367429 ) ) ;
#24721=CARTESIAN_POINT ( 'NONE',  ( -13.60973832552192775, -24.10531655226265357, -13.51781039733256229 ) ) ;
#24723=CARTESIAN_POINT ( 'NONE',  ( -15.77773026942784185, -13.10308996503666101, -29.22635037987518913 ) ) ;
#24724=CARTESIAN_POINT ( 'NONE',  ( -0.3788947411688599609, -24.40711055506037397, -9.394763118258644852 ) ) ;
#24725=CARTESIAN_POINT ( 'NONE',  ( 15.34816150809986013, 25.71129999911718755, -8.302060856640464337 ) ) ;
#24726=CARTESIAN_POINT ( 'NONE',  ( 19.07176576169624838, 8.856411245019137013, -24.40134652798608172 ) ) ;
#24729=CARTESIAN_POINT ( 'NONE',  ( -4.949370363199405709, 34.62182401653869590, -11.09161847530103984 ) ) ;
#24731=CARTESIAN_POINT ( 'NONE',  ( -20.04600691274970714, -4.289688609580842638, -30.00000000000000000 ) ) ;
#24736=CARTESIAN_POINT ( 'NONE',  ( -20.49737880956387670, 1.361707026421257183, -28.72413233336064664 ) ) ;
#24738=CARTESIAN_POINT ( 'NONE',  ( 29.79256524754709901, -11.96324064677705401, -13.83857493703202657 ) ) ;
#24747=CARTESIAN_POINT ( 'NONE',  ( -18.00000000000000000, 22.50000000000001066, 3.000000000000000000 ) ) ;
#24749=CARTESIAN_POINT ( 'NONE',  ( -2.264496061979761166, 20.62872948969808817, -27.72085884865996164 ) ) ;
#24754=CARTESIAN_POINT ( 'NONE',  ( 27.47508384939705550, -22.51065662569030223, -10.20476834957493395 ) ) ;
#24755=CARTESIAN_POINT ( 'NONE',  ( 19.54882725460437598, 14.50357661510694385, -10.87434924481359921 ) ) ;
#24756=CARTESIAN_POINT ( 'NONE',  ( 10.77366068177361491, 25.64106453496501103, -16.05906032174032916 ) ) ;
#24758=CARTESIAN_POINT ( 'NONE',  ( -20.68145323613758180, 13.65869002226675910, -6.453259564398977410 ) ) ;
#24760=CARTESIAN_POINT ( 'NONE',  ( 11.27261089013053308, -20.45316121506556684, -20.52991339251368075 ) ) ;
#24765=CARTESIAN_POINT ( 'NONE',  ( 17.81784622497951176, -13.85677843414110555, -30.00000000000001421 ) ) ;
#24768=CARTESIAN_POINT ( 'NONE',  ( -11.86970878780117467, 19.40623504760773699, -21.61272265936945658 ) ) ;
#24770=CARTESIAN_POINT ( 'NONE',  ( -19.68546449317618752, -22.09548208296689609, -14.94786901843714588 ) ) ;
#24771=CARTESIAN_POINT ( 'NONE',  ( 10.56601941806194667, -25.32872364259939246, -8.337176484249591013 ) ) ;
#24774=CARTESIAN_POINT ( 'NONE',  ( -10.00978049950840365, 33.59848884444493677, -8.937983356255100986 ) ) ;
#24779=CARTESIAN_POINT ( 'NONE',  ( 20.52560773323338950, 0.8855934539933489891, -28.70794251307378531 ) ) ;
#24784=CARTESIAN_POINT ( 'NONE',  ( -25.18774962667799855, 0.4227707108053092577, -17.44299664577632214 ) ) ;
#24788=CARTESIAN_POINT ( 'NONE',  ( 33.33943358355180919, -6.927885457322644491, -9.856513271172966384 ) ) ;
#24790=AXIS2_PLACEMENT_3D ( 'NONE', #40112, #37473, #3341 ) ;
#24805=CARTESIAN_POINT ( 'NONE',  ( 9.133087869482302779, 35.68701272469542829, -4.999999999999999112 ) ) ;
#24808=CARTESIAN_POINT ( 'NONE',  ( 11.58194518081183944, -17.66261609970828061, -26.04779429940238700 ) ) ;
#24814=CARTESIAN_POINT ( 'NONE',  ( -11.84249978353584964, 18.76146840030286711, -22.76060117347688561 ) ) ;
#24817=CARTESIAN_POINT ( 'NONE',  ( 14.73164756419078536, -25.80301381421831763, -9.711130863355320386 ) ) ;
#24818=CARTESIAN_POINT ( 'NONE',  ( 2.485571585149743523, -11.24999999999995737, 10.00000000000000000 ) ) ;
#24821=CARTESIAN_POINT ( 'NONE',  ( -14.26477007067611247, 27.22168516859696297, -10.08655638140778343 ) ) ;
#24822=CARTESIAN_POINT ( 'NONE',  ( -19.86157376375091488, -26.35897367172421468, -9.048130445010871270 ) ) ;
#24825=CARTESIAN_POINT ( 'NONE',  ( -34.75757652648396601, -9.699577992749013333, -8.031966576075948439 ) ) ;
#24827=CARTESIAN_POINT ( 'NONE',  ( -9.318012453479679991, -18.39830250787939292, -28.09118640345915452 ) ) ;
#24831=CARTESIAN_POINT ( 'NONE',  ( 30.66646233963074053, 0.1658458930697631339, -5.946129198316283393 ) ) ;
#24835=CARTESIAN_POINT ( 'NONE',  ( -30.37298050052526577, -0.02580378418990478956, -8.296495627326031297 ) ) ;
#24837=CARTESIAN_POINT ( 'NONE',  ( 20.74370561925601564, -0.3015135946092845076, -27.37350676080033196 ) ) ;
#24839=CARTESIAN_POINT ( 'NONE',  ( -6.026386652613112460, -19.60672597950843965, -29.99999999999999289 ) ) ;
#24843=CARTESIAN_POINT ( 'NONE',  ( -20.27261486981255700, 4.299876162282100012, -27.04395481629711995 ) ) ;
#24847=DIRECTION ( 'NONE',  ( 1.000000000000000000, 0.000000000000000000, 0.000000000000000000 ) ) ;
#24853=CARTESIAN_POINT ( 'NONE',  ( -19.73431017332725901, 6.432349763256766551, -26.55950874972816678 ) ) ;
#24856=CARTESIAN_POINT ( 'NONE',  ( 15.61542113695269762, -16.24202176434524958, -23.22363185398829089 ) ) ;
#24858=CARTESIAN_POINT ( 'NONE',  ( 15.32268921037612586, 27.10638078547256669, -4.999999999999999112 ) ) ;
#24861=CARTESIAN_POINT ( 'NONE',  ( -16.22408403259154852, 24.10865257618694102, -5.000000000000000000 ) ) ;
#24866=CARTESIAN_POINT ( 'NONE',  ( 15.25901309658000748, 26.31556895002759688, -7.828263233713028235 ) ) ;
#24870=CARTESIAN_POINT ( 'NONE',  ( -11.55131371627300751, 19.04040767486820940, -22.71169724931953482 ) ) ;
#24872=CARTESIAN_POINT ( 'NONE',  ( -11.33073861718174236, -20.44271155232068793, -20.52225160477277299 ) ) ;
#24875=CARTESIAN_POINT ( 'NONE',  ( -32.12531547378703323, -14.37956203216488049, -11.07915535210666924 ) ) ;
#24876=CARTESIAN_POINT ( 'NONE',  ( -13.73743966556329887, -26.04782550432431165, -7.836754151373586552 ) ) ;
#24878=CARTESIAN_POINT ( 'NONE',  ( 15.30794202828028361, 22.03102559147765405, -12.64584791074079284 ) ) ;
#24880=CARTESIAN_POINT ( 'NONE',  ( 22.62389337662363076, 5.347323980972150892, -17.84045304431403522 ) ) ;
#24886=CARTESIAN_POINT ( 'NONE',  ( -29.84605808524375803, -0.2300388918764082746, -10.15910822650677048 ) ) ;
#24887=CARTESIAN_POINT ( 'NONE',  ( 24.67091124240074862, 0.2026903286398813175, -18.42105149346458859 ) ) ;
#24893=CARTESIAN_POINT ( 'NONE',  ( -7.289639608743041066, -27.06962010326280321, -5.000000000000000000 ) ) ;
#24901=CYLINDRICAL_SURFACE ( 'NONE', #214, 21.00000000000002842 ) ;
#24902=CARTESIAN_POINT ( 'NONE',  ( 2.625031239634822100, 36.35909348746493919, -9.730352021840648291 ) ) ;
#24909=CARTESIAN_POINT ( 'NONE',  ( 15.04722313270411327, 27.70573751427465226, -6.401096178813311610 ) ) ;
#24912=CARTESIAN_POINT ( 'NONE',  ( -18.38703319206937081, 17.23187950328362916, -9.851216774087896866 ) ) ;
#24917=CARTESIAN_POINT ( 'NONE',  ( 14.75481277935874935, -25.65575037643989376, -10.18041772782883214 ) ) ;
#24918=CARTESIAN_POINT ( 'NONE',  ( -22.54724872518345080, -26.68010991916779062, -7.210959810203029896 ) ) ;
#24919=CARTESIAN_POINT ( 'NONE',  ( 15.42079449665415680, 26.76609254708107244, -5.000000000000002665 ) ) ;
#24920=CARTESIAN_POINT ( 'NONE',  ( 15.22764080799647068, 26.42222000209493160, -7.827247944502371269 ) ) ;
#24925=CARTESIAN_POINT ( 'NONE',  ( -14.99825077041236909, -26.12718959772186267, -8.768476732925005734 ) ) ;
#24927=CARTESIAN_POINT ( 'NONE',  ( -18.37535949686024495, -13.48922921807925590, -23.01936354672100293 ) ) ;
#24928=CARTESIAN_POINT ( 'NONE',  ( -0.3658111510020998769, -23.95295762298067643, -11.88201142430637880 ) ) ;
#24929=CARTESIAN_POINT ( 'NONE',  ( 11.19848097534155684, 17.17100607549662072, -30.00000000000000355 ) ) ;
#24930=EDGE_CURVE ( 'NONE', #10849, #7392, #19304, .T. ) ;
#24931=CARTESIAN_POINT ( 'NONE',  ( 21.72105953519021782, 10.88454294244725062, -10.38293942656555480 ) ) ;
#24935=CARTESIAN_POINT ( 'NONE',  ( -21.03490419256541344, -2.515787243126888395, -25.94069391000374836 ) ) ;
#24940=CARTESIAN_POINT ( 'NONE',  ( -30.22364946210556624, 0.6259246664836076723, -5.946350832945448417 ) ) ;
#24941=CARTESIAN_POINT ( 'NONE',  ( 23.14110463828941278, -7.760064457001075056, -20.81805854442341541 ) ) ;
#24953=CARTESIAN_POINT ( 'NONE',  ( -3.020371057517535984, 37.41995014423672217, -7.977523484556464872 ) ) ;
#24954=CARTESIAN_POINT ( 'NONE',  ( 3.863783140547853712E-14, -86.77689918168233874, 0.000000000000000000 ) ) ;
#24959=CARTESIAN_POINT ( 'NONE',  ( 8.712215903382341864, 20.44729472759973632, -23.46250027292118290 ) ) ;
#24962=CARTESIAN_POINT ( 'NONE',  ( -20.62288446763035665, 13.61555273158426083, -7.427349022565545411 ) ) ;
#24964=CARTESIAN_POINT ( 'NONE',  ( 15.68314276670921359, -26.79173994879206688, -5.000000000000000888 ) ) ;
#24966=CARTESIAN_POINT ( 'NONE',  ( 14.26301124034561774, 24.54581302918253627, -12.54423936124191741 ) ) ;
#24967=CARTESIAN_POINT ( 'NONE',  ( -26.31271763591404422, -28.25584584496042240, -5.000000000000000888 ) ) ;
#24970=CARTESIAN_POINT ( 'NONE',  ( -15.28113052511585224, 26.56228617015612414, -7.356869252458130504 ) ) ;
#24971=CARTESIAN_POINT ( 'NONE',  ( -14.67729291545832560, -14.63692594569341310, -27.79627455608592967 ) ) ;
#24972=CARTESIAN_POINT ( 'NONE',  ( 8.752986035078182070, -18.86042647000214956, -26.90452173386816526 ) ) ;
#24973=CARTESIAN_POINT ( 'NONE',  ( 11.05718465110185988, 17.26235906992462787, -30.00000000000000000 ) ) ;
#24974=CARTESIAN_POINT ( 'NONE',  ( 31.64736106748093647, -21.41673248936808349, -6.278375262888240549 ) ) ;
#24977=CARTESIAN_POINT ( 'NONE',  ( -8.406664792321896229, 25.38477432831364311, -17.87301269380117930 ) ) ;
#24983=CARTESIAN_POINT ( 'NONE',  ( 21.27582338407567519, 0.7799646396183672614, -25.01502835885500176 ) ) ;
#24984=CARTESIAN_POINT ( 'NONE',  ( -14.21391437420826165, 30.04769070240181250, -4.999999999999998224 ) ) ;
#24988=CARTESIAN_POINT ( 'NONE',  ( -20.69269121772957121, 0.8588170339218694771, -27.44912421251707713 ) ) ;
#24991=CARTESIAN_POINT ( 'NONE',  ( 33.82615122060476409, -6.056122843722836713, -8.538783554659925557 ) ) ;
#24993=CIRCLE ( 'NONE', #20538, 16.00000000000000000 ) ;
#25000=PLANE ( 'NONE',  #33074 ) ;
#25003=CARTESIAN_POINT ( 'NONE',  ( -12.69445121025463763, 16.09979585365689658, -29.99999999999999289 ) ) ;
#25006=CARTESIAN_POINT ( 'NONE',  ( 7.569476015651482648, 29.31452674637723277, -14.85894962403729203 ) ) ;
#25007=CARTESIAN_POINT ( 'NONE',  ( 13.87647862417395572, -21.94196052813751052, -17.25938925699875881 ) ) ;
#25013=CARTESIAN_POINT ( 'NONE',  ( -11.20417644663015366, 17.31670387387610432, -28.08716411289236703 ) ) ;
#25016=CARTESIAN_POINT ( 'NONE',  ( 12.90216916962276983, -23.08619710550532744, -15.45772932541511580 ) ) ;
#25021=CARTESIAN_POINT ( 'NONE',  ( -12.65668046281904502, 25.53506749916461871, -14.26639179336292784 ) ) ;
#25022=CARTESIAN_POINT ( 'NONE',  ( -11.63144283470464480, -16.96580988189544570, -28.62035570873908341 ) ) ;
#25026=CARTESIAN_POINT ( 'NONE',  ( -31.89533340862117683, -9.891971453653612301, -12.04687614664414674 ) ) ;
#25027=CARTESIAN_POINT ( 'NONE',  ( -10.73556218567333254, -20.01456250315406393, -21.62972654522360827 ) ) ;
#25030=CARTESIAN_POINT ( 'NONE',  ( 20.94835144443074881, 1.007079124089848232, -26.24203246979738324 ) ) ;
#25034=CARTESIAN_POINT ( 'NONE',  ( -20.69701185487514294, 0.7957416167526897288, -27.44504335574468001 ) ) ;
#25036=CARTESIAN_POINT ( 'NONE',  ( 32.28014819601976626, -2.247453943413153077, -7.746584525066519511 ) ) ;
#25037=CARTESIAN_POINT ( 'NONE',  ( 18.33518551373228789, -9.195211339103170900, -30.00000000000004263 ) ) ;
#25040=CARTESIAN_POINT ( 'NONE',  ( -26.05480634030368137, 4.388949531393018688, -10.28550515634381668 ) ) ;
#25053=CARTESIAN_POINT ( 'NONE',  ( -23.47028999752262735, 7.894751856600318973, -10.85062483233681974 ) ) ;
#25056=CARTESIAN_POINT ( 'NONE',  ( 17.36693989509100788, -19.17194112829468366, -18.88888385720245822 ) ) ;
#25059=CARTESIAN_POINT ( 'NONE',  ( 12.25371331340743097, 20.67270376835447365, -19.46752873204117051 ) ) ;
#25061=CARTESIAN_POINT ( 'NONE',  ( -14.53679685137945832, 21.79695616867457630, -14.57185096994714080 ) ) ;
#25065=CARTESIAN_POINT ( 'NONE',  ( 12.15864794129231186, 19.89114798110919580, -20.54594864371944141 ) ) ;
#25069=CARTESIAN_POINT ( 'NONE',  ( -15.07291816638977622, 26.61547165230870959, -8.284995957625287843 ) ) ;
#25071=CARTESIAN_POINT ( 'NONE',  ( -15.53477848226612679, -26.63013453484452597, -6.884701492020882441 ) ) ;
#25075=CARTESIAN_POINT ( 'NONE',  ( -34.90754895111634681, -15.66705718490307753, -5.436414939066039231 ) ) ;
#25076=CARTESIAN_POINT ( 'NONE',  ( -10.06357074363348580, -20.17046618015623238, -21.70867519228511000 ) ) ;
#25078=CARTESIAN_POINT ( 'NONE',  ( 16.49060731112116684, 23.31193391774742807, -5.000000000000002665 ) ) ;
#25080=CARTESIAN_POINT ( 'NONE',  ( 21.49663310311013120, 5.283455890831983304, -20.99229874812046504 ) ) ;
#25084=CARTESIAN_POINT ( 'NONE',  ( -15.52302998184525507, -20.83641103980755460, -18.06021460543220414 ) ) ;
#25086=CARTESIAN_POINT ( 'NONE',  ( -20.50193171233730993, 0.1922071591807820723, -29.99999999999999645 ) ) ;
#25087=CARTESIAN_POINT ( 'NONE',  ( 30.81151147059108908, -0.3616763097095250790, -7.812778536805358165 ) ) ;
#25090=CARTESIAN_POINT ( 'NONE',  ( -35.36940577612494963, -20.42053594592268695, -14.51648065752878480 ) ) ;
#25091=DIRECTION ( 'NONE',  ( 0.000000000000000000, 0.000000000000000000, 1.000000000000000000 ) ) ;
#25092=EDGE_LOOP ( 'NONE', ( #1109, #11985, #9404, #27391 ) ) ;
#25099=CARTESIAN_POINT ( 'NONE',  ( 0.8413128747587147460, 20.74004676862665519, -27.70638048767625605 ) ) ;
#25107=CARTESIAN_POINT ( 'NONE',  ( 13.83999196091766848, 25.56421401852912112, -12.46077667759507790 ) ) ;
#25111=CARTESIAN_POINT ( 'NONE',  ( -14.95315193416318245, 14.07753665216654682, -28.83165291678060882 ) ) ;
#25114=CARTESIAN_POINT ( 'NONE',  ( 9.675278753175428292, -18.44830207160445923, -26.83172255620764446 ) ) ;
#25115=CARTESIAN_POINT ( 'NONE',  ( -21.63262549566270465, -25.67952849192365861, -9.885633078860415424 ) ) ;
#25116=CARTESIAN_POINT ( 'NONE',  ( 15.41782702884244571, 26.77676039938714325, -5.000000000000000000 ) ) ;
#25117=CARTESIAN_POINT ( 'NONE',  ( 14.92826937204305793, 25.82090953808645040, -9.707752144388164695 ) ) ;
#25120=CARTESIAN_POINT ( 'NONE',  ( -15.39818770356525768, -26.71945962344603487, -5.474181265265219309 ) ) ;
#25122=CARTESIAN_POINT ( 'NONE',  ( -16.15747483659607298, -12.61697622026560772, -29.22209380604542872 ) ) ;
#25123=CARTESIAN_POINT ( 'NONE',  ( -2.594368725792287833, -24.77623966133340261, -5.966968964887910509 ) ) ;
#25124=CARTESIAN_POINT ( 'NONE',  ( 15.11376219116451836, 24.32797801075062338, -10.67731718876905234 ) ) ;
#25125=CARTESIAN_POINT ( 'NONE',  ( 19.97175965172673529, 9.167974992394606559, -20.10623141010908910 ) ) ;
#25129=CARTESIAN_POINT ( 'NONE',  ( -33.99706561663532511, -4.510256399178081743, -5.000000000000002665 ) ) ;
#25134=CARTESIAN_POINT ( 'NONE',  ( 19.48557158514988075, -11.24999999999998224, 6.000000000000000000 ) ) ;
#25137=CARTESIAN_POINT ( 'NONE',  ( -21.64275424889105182, 1.072163566031019144, -23.89394571961734570 ) ) ;
#25138=CARTESIAN_POINT ( 'NONE',  ( 33.31245343632154032, -12.22087107712299847, -10.20715524599960311 ) ) ;
#25147=ORIENTED_EDGE ( 'NONE', *, *, #3943, .F. ) ;
#25149=CARTESIAN_POINT ( 'NONE',  ( -3.068187625016429276, 38.20266742920320269, -5.436115964257634658 ) ) ;
#25151=CARTESIAN_POINT ( 'NONE',  ( -19.48557158514985588, -11.25000000000002309, 6.000000000000000000 ) ) ;
#25158=CARTESIAN_POINT ( 'NONE',  ( 8.094548601407083765, 18.84590462288236878, -29.99999999999999289 ) ) ;
#25160=ORIENTED_EDGE ( 'NONE', *, *, #5935, .T. ) ;
#25161=CARTESIAN_POINT ( 'NONE',  ( -20.35271757330227516, 13.41710386861673854, -9.887965968330341582 ) ) ;
#25163=CARTESIAN_POINT ( 'NONE',  ( 11.95392418477062257, -21.48168688891967193, -18.44634885117927325 ) ) ;
#25165=CARTESIAN_POINT ( 'NONE',  ( 11.26454620336414791, 18.07348392246389324, -25.00831616619147724 ) ) ;
#25166=AXIS2_PLACEMENT_3D ( 'NONE', #17064, #30252, #24145 ) ;
#25167=CARTESIAN_POINT ( 'NONE',  ( -13.28992586503615669, -18.25382200079944539, -20.55760979252988463 ) ) ;
#25170=CARTESIAN_POINT ( 'NONE',  ( -24.08910206099691464, -25.46756753362905812, -8.938104685036856623 ) ) ;
#25171=CARTESIAN_POINT ( 'NONE',  ( 12.85889123487801555, -25.78048515081998104, -8.316609656120787619 ) ) ;
#25172=CARTESIAN_POINT ( 'NONE',  ( 13.32213502064756483, 22.03573321722581113, -16.46143111696509465 ) ) ;
#25173=CARTESIAN_POINT ( 'NONE',  ( 19.24076220952862926, -13.86809943524113997, -21.86721313143632983 ) ) ;
#25179=CARTESIAN_POINT ( 'NONE',  ( -7.551239285968937232, 22.78181879830267675, -21.00978300683897615 ) ) ;
#25184=CARTESIAN_POINT ( 'NONE',  ( 20.96668529434488448, 0.8362590005558052653, -26.22736366994790913 ) ) ;
#25188=CARTESIAN_POINT ( 'NONE',  ( -30.86332187973009056, -0.0005132856539961011327, -5.474190270091115806 ) ) ;
#25189=CARTESIAN_POINT ( 'NONE',  ( -20.57926082973601822, -27.21289976943432265, -5.455544558421332013 ) ) ;
#25191=CARTESIAN_POINT ( 'NONE',  ( 20.42343116704461892, -4.183005399031937799, -27.14234199482063659 ) ) ;
#25204=CARTESIAN_POINT ( 'NONE',  ( -20.31755536841790288, -2.811235405436151247, -30.00000000000001066 ) ) ;
#25205=CARTESIAN_POINT ( 'NONE',  ( 19.48557158514975285, -11.24999999999995737, 10.00000000000000000 ) ) ;
#25207=CARTESIAN_POINT ( 'NONE',  ( 17.48494887651980534, 18.07252522714370002, -11.80118198379806316 ) ) ;
#25208=CARTESIAN_POINT ( 'NONE',  ( 5.618065306669937975, 21.88280708645027772, -23.17586028251368546 ) ) ;
#25209=CARTESIAN_POINT ( 'NONE',  ( 11.81349784526102908, -17.96894529079195379, -24.79472172074744307 ) ) ;
#25214=CARTESIAN_POINT ( 'NONE',  ( -10.99360060711668474, 17.30291464612033181, -29.34855223075900454 ) ) ;
#25217=CARTESIAN_POINT ( 'NONE',  ( 15.12799067885430659, -26.57699633146447482, -6.417320784827945879 ) ) ;
#25223=CARTESIAN_POINT ( 'NONE',  ( -14.41188954600920447, 29.53590640632083719, -5.000000000000000000 ) ) ;
#25224=CARTESIAN_POINT ( 'NONE',  ( -11.76462635582750593, -17.13989212898560410, -27.28828191877128972 ) ) ;
#25226=CARTESIAN_POINT ( 'NONE',  ( -23.24156206836136818, -7.249540115697041820, -20.84616574791856891 ) ) ;
#25227=CARTESIAN_POINT ( 'NONE',  ( -9.609681352058309756, -18.47898454444922933, -26.83723954853537919 ) ) ;
#25230=CARTESIAN_POINT ( 'NONE',  ( 30.64962079249725946, 0.2186612821100236415, -5.474121491177763588 ) ) ;
#25234=CARTESIAN_POINT ( 'NONE',  ( -27.76379728900110777, 0.1559794775103171827, -13.51035586821201129 ) ) ;
#25236=CARTESIAN_POINT ( 'NONE',  ( 20.64647571109192370, -0.6209930936118700506, -28.00345359345995888 ) ) ;
#25246=ADVANCED_FACE ( 'NONE', ( #34395 ), #30948, .T. ) ;
#25247=EDGE_CURVE ( 'NONE', #33201, #33096, #18707, .T. ) ;
#25253=CARTESIAN_POINT ( 'NONE',  ( -19.30609231752467991, 7.879336912585563013, -25.47724169212735390 ) ) ;
#25254=CARTESIAN_POINT ( 'NONE',  ( 14.20597032484196376, -14.79219592438034780, -29.25104138637490436 ) ) ;
#25256=CARTESIAN_POINT ( 'NONE',  ( 10.89810581091218111, 17.51759729559895717, -28.06894606240402013 ) ) ;
#25257=ORIENTED_EDGE ( 'NONE', *, *, #32788, .T. ) ;
#25258=CARTESIAN_POINT ( 'NONE',  ( -12.82984808660655318, 16.00373636590108362, -29.38416646348882111 ) ) ;
#25261=CARTESIAN_POINT ( 'NONE',  ( 15.44165670342503205, 26.69129292160669920, -5.000000000000000000 ) ) ;
#25263=LINE ( 'NONE', #22017, #861 ) ;
#25266=CARTESIAN_POINT ( 'NONE',  ( -10.85292483170471023, 17.44571412242369490, -28.70057752128876771 ) ) ;
#25269=CARTESIAN_POINT ( 'NONE',  ( -15.61601735593368012, -26.74911251005942603, -5.944523841747975546 ) ) ;
#25273=VERTEX_POINT ( 'NONE', #23952 ) ;
#25274=CARTESIAN_POINT ( 'NONE',  ( -19.01544318679556511, -9.256926599663669819, -26.26492384747328757 ) ) ;
#25275=CARTESIAN_POINT ( 'NONE',  ( -14.02798880308901275, -26.11055631809762900, -7.834863257364764522 ) ) ;
#25277=CARTESIAN_POINT ( 'NONE',  ( 12.50874981011069664, 16.57754095322059484, -26.94891225080305830 ) ) ;
#25279=CARTESIAN_POINT ( 'NONE',  ( 24.28730508192998983, 4.587782948896792057, -14.73921855142076076 ) ) ;
#25283=CIRCLE ( 'NONE', #7762, 16.00000000000001066 ) ;
#25285=CARTESIAN_POINT ( 'NONE',  ( -27.40511294215596649, -0.1367760914176404108, -14.43413953572169817 ) ) ;
#25286=CARTESIAN_POINT ( 'NONE',  ( 20.62252632493563098, 0.6248223115394143656, -28.06621906308379266 ) ) ;
#25289=CARTESIAN_POINT ( 'NONE',  ( -11.41987377193683528, -19.41918266173334828, -20.90349153980999475 ) ) ;
#25294=CARTESIAN_POINT ( 'NONE',  ( 10.09922753093620962, -27.41777246569289517, -5.000000000000000000 ) ) ;
#25298=CARTESIAN_POINT ( 'NONE',  ( 20.20214925878792656, 14.56229221523759598, -4.999999999999995559 ) ) ;
#25299=CARTESIAN_POINT ( 'NONE',  ( 2.098354962282032776, 20.79632631842905610, -26.98459398919786523 ) ) ;
#25306=CARTESIAN_POINT ( 'NONE',  ( 14.68376815913365085, 27.36567026352939891, -8.715261669753955331 ) ) ;
#25309=CARTESIAN_POINT ( 'NONE',  ( -15.66915680351796070, 13.81629364357497458, -25.43784811616387032 ) ) ;
#25312=CARTESIAN_POINT ( 'NONE',  ( 10.51168368352045057, -19.58291515952883444, -22.73802084914789390 ) ) ;
#25314=CARTESIAN_POINT ( 'NONE',  ( 11.30648189521332725, 18.04080162384157759, -25.01410076809225913 ) ) ;
#25315=CARTESIAN_POINT ( 'NONE',  ( 15.41110799979362511, 26.80090896191098793, -5.000000000000000000 ) ) ;
#25317=CARTESIAN_POINT ( 'NONE',  ( -12.92003364848273783, -23.08707941010340647, -15.45656058803134059 ) ) ;
#25320=CARTESIAN_POINT ( 'NONE',  ( -30.72590368136143724, -21.21574487496830841, -8.410142833198055001 ) ) ;
#25321=CARTESIAN_POINT ( 'NONE',  ( -1.830947598378612096, -20.80176537255082891, -25.50661662362668736 ) ) ;
#25322=CARTESIAN_POINT ( 'NONE',  ( 14.08529064057289482, 22.72790877343337712, -14.51632245905989649 ) ) ;
#25324=CARTESIAN_POINT ( 'NONE',  ( 18.60021360422396342, 8.694919316221673355, -28.85921347423368388 ) ) ;
#25328=CARTESIAN_POINT ( 'NONE',  ( -20.47084386718785609, -3.078924522425823707, -27.88626578634149666 ) ) ;
#25334=CARTESIAN_POINT ( 'NONE',  ( -20.80015496576257661, 2.182957871452693599, -26.33707758174465496 ) ) ;
#25335=CARTESIAN_POINT ( 'NONE',  ( 26.75366824387117148, -10.76373612552858638, -16.67183740961663929 ) ) ;
#25344=CARTESIAN_POINT ( 'NONE',  ( -2.329603726064299885, 28.90242561963931678, -16.64147633399780446 ) ) ;
#25351=CARTESIAN_POINT ( 'NONE',  ( 9.546848429036838724, 20.70351224251990274, -22.40024640956508151 ) ) ;
#25353=CARTESIAN_POINT ( 'NONE',  ( -18.43601137689102742, 10.05164828422247503, -24.41288531576839205 ) ) ;
#25355=CARTESIAN_POINT ( 'NONE',  ( 13.43826639690882985, -23.62933372394671139, -14.47033993370646598 ) ) ;
#25358=CARTESIAN_POINT ( 'NONE',  ( 14.50167871676907616, 25.05847836359596315, -11.59245320002316504 ) ) ;
#25359=CARTESIAN_POINT ( 'NONE',  ( 31.47283671532267846, -25.12609584734865464, -14.45070082761209207 ) ) ;
#25361=CARTESIAN_POINT ( 'NONE',  ( -24.69306225852445991, -24.64882393665288518, -9.807970858657039770 ) ) ;
#25362=CARTESIAN_POINT ( 'NONE',  ( 6.225823723043348856, -25.00732421141256978, -6.924410079875567448 ) ) ;
#25363=CARTESIAN_POINT ( 'NONE',  ( 14.10414194694077494, 23.76207731977601156, -13.52159713385365869 ) ) ;
#25364=CARTESIAN_POINT ( 'NONE',  ( 30.82101031815450654, -22.25462399755607379, -6.702141387976242370 ) ) ;
#25369=CARTESIAN_POINT ( 'NONE',  ( -5.884614315209530488, 19.64670892508010169, -29.25345033631867153 ) ) ;
#25373=CARTESIAN_POINT ( 'NONE',  ( 23.33050994933525146, 0.5154748466008040042, -20.53702464707256681 ) ) ;
#25378=EDGE_CURVE ( 'NONE', #9588, #40031, #4404, .T. ) ;
#25380=CARTESIAN_POINT ( 'NONE',  ( -29.77291926438935477, 0.07581751844958646569, -9.709798205980805008 ) ) ;
#25383=CARTESIAN_POINT ( 'NONE',  ( 34.70961424076313051, -8.320133917892743369, -7.618081809658795223 ) ) ;
#25392=CARTESIAN_POINT ( 'NONE',  ( -20.30900398262955520, 3.084420529719719362, -30.00000000000000000 ) ) ;
#25397=CARTESIAN_POINT ( 'NONE',  ( 15.58421666608182399, 16.80577185948362029, -18.86466076104356659 ) ) ;
#25398=CARTESIAN_POINT ( 'NONE',  ( 6.528576035962029955, 25.38036280295423808, -18.79159262674204456 ) ) ;
#25402=CARTESIAN_POINT ( 'NONE',  ( 16.24958219909836288, -26.89404583347094047, -5.938197498648205119 ) ) ;
#25406=CARTESIAN_POINT ( 'NONE',  ( -11.05465679327823558, 17.41536169098398545, -28.07828314278957293 ) ) ;
#25408=CARTESIAN_POINT ( 'NONE',  ( 9.496368407746681228, -18.31046244359924202, -28.08151151955017255 ) ) ;
#25413=CARTESIAN_POINT ( 'NONE',  ( -8.333876625047521358, 18.93681600531247611, -27.92366777036197334 ) ) ;
#25417=CARTESIAN_POINT ( 'NONE',  ( -35.24538222971869317, -9.860299811780501855, -6.734244107179631733 ) ) ;
#25418=CARTESIAN_POINT ( 'NONE',  ( -15.26244400023809078, -26.61077467321880974, -6.417168005406195697 ) ) ;
#25421=CARTESIAN_POINT ( 'NONE',  ( 23.88555579540136620, 0.6173852234973284947, -19.51149964275768411 ) ) ;
#25422=CARTESIAN_POINT ( 'NONE',  ( 14.94435605704140357, 25.81679485013957631, -9.707589803872810563 ) ) ;
#25425=CARTESIAN_POINT ( 'NONE',  ( -21.28292253093711750, 0.7291719054457980187, -25.00947294987627600 ) ) ;
#25427=CARTESIAN_POINT ( 'NONE',  ( 32.75437695154221274, -2.309567439508531717, -5.000000000000000000 ) ) ;
#25428=CARTESIAN_POINT ( 'NONE',  ( -2.006248926576237324, -20.44716014466324694, -30.00000000000000711 ) ) ;
#25440=CARTESIAN_POINT ( 'NONE',  ( -22.74231906068476050, 9.811850412294511159, -8.402255488763186619 ) ) ;
#25441=CARTESIAN_POINT ( 'NONE',  ( 21.92413472738710212, -26.98779261574284760, -6.338459772264864789 ) ) ;
#25443=CARTESIAN_POINT ( 'NONE',  ( 15.34417538557263683, 26.94339626938088372, -5.944057201105769295 ) ) ;
#25445=CARTESIAN_POINT ( 'NONE',  ( -11.71642904664754070, 16.82516707186347915, -29.36357973296176027 ) ) ;
#25449=CARTESIAN_POINT ( 'NONE',  ( 12.41725554300025713, 20.45587985069801107, -19.50104749346444422 ) ) ;
#25451=CARTESIAN_POINT ( 'NONE',  ( 30.99684195017841404, -17.08716579088729759, -11.06784137463484008 ) ) ;
#25454=CARTESIAN_POINT ( 'NONE',  ( -14.79267235827050619, 26.23776883278636518, -9.685074664482419493 ) ) ;
#25456=CARTESIAN_POINT ( 'NONE',  ( -15.57329205153430429, -25.98394400221819467, -9.671856144017159096 ) ) ;
#25461=CARTESIAN_POINT ( 'NONE',  ( -18.15436357158603897, -9.522238560471439683, -30.00000000000001421 ) ) ;
#25462=CARTESIAN_POINT ( 'NONE',  ( -10.56852682390984199, -20.57919107763412114, -20.61136777398266062 ) ) ;
#25464=CARTESIAN_POINT ( 'NONE',  ( 12.66487866387964978, 16.11973886863585648, -30.00000000000000711 ) ) ;
#25466=CARTESIAN_POINT ( 'NONE',  ( 19.82221245355347605, 5.923645454667767041, -27.10773064487408845 ) ) ;
#25472=CARTESIAN_POINT ( 'NONE',  ( -20.71452086892951172, 0.5024582651441130698, -27.42597503545741944 ) ) ;
#25473=CARTESIAN_POINT ( 'NONE',  ( 29.10019562751751820, -0.1449826646537783481, -11.57629332465059235 ) ) ;
#25477=CARTESIAN_POINT ( 'NONE',  ( -17.81784622497958281, -13.85677843414106292, -30.00000000000001421 ) ) ;
#25484=CARTESIAN_POINT ( 'NONE',  ( 28.92287456541829371, 1.976372635698110614, -4.999999999999999112 ) ) ;
#25485=CARTESIAN_POINT ( 'NONE',  ( 6.045822647813611006, 36.95161842508870365, -7.135958126947899771 ) ) ;
#25491=CARTESIAN_POINT ( 'NONE',  ( 30.14285136919114549, -23.17491017602459280, -5.860341728232943304 ) ) ;
#25495=CARTESIAN_POINT ( 'NONE',  ( 14.90518469689150827, 26.75391244360456966, -8.740800605981732474 ) ) ;
#25498=AXIS2_PLACEMENT_3D ( 'NONE', #37785, #28244, #12605 ) ;
#25499=CARTESIAN_POINT ( 'NONE',  ( -15.89936984974615619, 18.38899797113655055, -15.74513658678639061 ) ) ;
#25502=CARTESIAN_POINT ( 'NONE',  ( 15.45091137245021429, -26.73300375246232008, -5.474195469181999840 ) ) ;
#25504=CARTESIAN_POINT ( 'NONE',  ( 15.29638078504309817, 26.50914737159216372, -7.357895937986722146 ) ) ;
#25505=EDGE_LOOP ( 'NONE', ( #13594, #15396, #29791, #39472 ) ) ;
#25506=CARTESIAN_POINT ( 'NONE',  ( 13.48417877264113685, 22.82990984439727811, -15.44940169434631727 ) ) ;
#25509=CARTESIAN_POINT ( 'NONE',  ( -15.37403055690315590, -26.58998761537970168, -6.888177748688296020 ) ) ;
#25513=CARTESIAN_POINT ( 'NONE',  ( -25.72242270509724449, -17.76379069224040563, -14.74151087500952073 ) ) ;
#25514=CARTESIAN_POINT ( 'NONE',  ( -3.881175749157317334, -22.08623497455011631, -19.01312672737709519 ) ) ;
#25515=CARTESIAN_POINT ( 'NONE',  ( 15.58265619670584989, 25.25374846204108081, -7.834539407195180161 ) ) ;
#25517=EDGE_CURVE ( 'NONE', #25273, #34673, #40182, .T. ) ;
#25518=CARTESIAN_POINT ( 'NONE',  ( 22.26700180465959633, 9.975047470158974861, -10.37867134500859301 ) ) ;
#25522=CARTESIAN_POINT ( 'NONE',  ( -33.65402088194174723, -4.443209378264873166, -7.242161384985005945 ) ) ;
#25527=CARTESIAN_POINT ( 'NONE',  ( -19.48557158514998022, -11.24999999999982414, 3.000000000000000000 ) ) ;
#25530=CARTESIAN_POINT ( 'NONE',  ( 30.43074936207083780, -13.30772945900434756, -12.90888064005893909 ) ) ;
#25536=CARTESIAN_POINT ( 'NONE',  ( -15.41813410374787807, 26.77565562682181266, -5.000000000000003553 ) ) ;
#25538=EDGE_CURVE ( 'NONE', #32074, #9588, #29752, .T. ) ;
#25542=CARTESIAN_POINT ( 'NONE',  ( -0.4275284198932905455, 22.02762823501048217, -24.21675859296236055 ) ) ;
#25548=COLOUR_RGB ( '', 0.31764706, 0.68627451, 0.89019608) ;
#25549=CARTESIAN_POINT ( 'NONE',  ( 13.91852109418007544, 29.04111810746936229, -8.650529261331366015 ) ) ;
#25552=CARTESIAN_POINT ( 'NONE',  ( -19.72315440816933219, 10.70534603068222168, -18.01648663879400303 ) ) ;
#25555=CARTESIAN_POINT ( 'NONE',  ( 10.35225884972404664, -19.11980502629199208, -23.83773470646794479 ) ) ;
#25556=CARTESIAN_POINT ( 'NONE',  ( 15.02655339034802395, -26.00115400090650652, -9.236043780760597954 ) ) ;
#25558=CARTESIAN_POINT ( 'NONE',  ( 11.43104729973414102, 18.48323776028994203, -23.84550412495152116 ) ) ;
#25559=CARTESIAN_POINT ( 'NONE',  ( -35.36940577612494963, -20.42053594592268695, -14.51648065752878480 ) ) ;
#25563=CARTESIAN_POINT ( 'NONE',  ( -22.71156489100481934, -22.69643118484121658, -13.00228647887131750 ) ) ;
#25564=CARTESIAN_POINT ( 'NONE',  ( 6.205112128679617811, -24.95655587313122581, -7.408272597870006138 ) ) ;
#25565=CARTESIAN_POINT ( 'NONE',  ( 13.04743348150465643, 21.46120596883949005, -17.45731936358998126 ) ) ;
#25567=CARTESIAN_POINT ( 'NONE',  ( 31.72993655656084755, -21.47020083663496237, -5.857146272187097047 ) ) ;
#25571=CARTESIAN_POINT ( 'NONE',  ( -7.859885379884856249, 33.27431112823943948, -11.13818915821171274 ) ) ;
#25575=CARTESIAN_POINT ( 'NONE',  ( 20.61132694413180388, 0.8343915772789830543, -28.07671223784028314 ) ) ;
#25579=CARTESIAN_POINT ( 'NONE',  ( -29.71183529215159780, 0.1435226407617324063, -9.711128893466487000 ) ) ;
#25582=CARTESIAN_POINT ( 'NONE',  ( 35.10761102947512313, -8.438163957854742492, -6.314036995521373541 ) ) ;
#25593=DIRECTION ( 'NONE',  ( 1.000000000000000000, 0.000000000000000000, 0.000000000000000000 ) ) ;
#25594=CARTESIAN_POINT ( 'NONE',  ( 4.987357081044728524, 19.92651000211460044, -30.00000000000000000 ) ) ;
#25598=CARTESIAN_POINT ( 'NONE',  ( 17.47098692575351819, 19.68410474348366179, -8.844102737791779134 ) ) ;
#25599=CARTESIAN_POINT ( 'NONE',  ( 9.086865688058274770, 35.45071178617213548, -6.734195449777575782 ) ) ;
#25601=CARTESIAN_POINT ( 'NONE',  ( 11.71983824754993542, -20.36894919573499863, -20.47130099390510338 ) ) ;
#25604=CIRCLE ( 'NONE', #4210, 18.00000000000000355 ) ;
#25606=CARTESIAN_POINT ( 'NONE',  ( -11.12856712346650312, 17.61049140408264080, -26.83074947876917449 ) ) ;
#25608=CARTESIAN_POINT ( 'NONE',  ( 9.271440805881887570, -18.28379014461920349, -29.35293047210549489 ) ) ;
#25612=CARTESIAN_POINT ( 'NONE',  ( -13.62515121305021637, 29.87907916796226360, -8.173113224430574419 ) ) ;
#25614=DIRECTION ( 'NONE',  ( 0.000000000000000000, 0.000000000000000000, -1.000000000000000000 ) ) ;
#25617=CARTESIAN_POINT ( 'NONE',  ( -19.91373213366430761, -4.906168661338282888, -29.25106315047995054 ) ) ;
#25620=CARTESIAN_POINT ( 'NONE',  ( 22.19098149685552102, 0.7861450883651701638, -22.74982018612348966 ) ) ;
#25625=CARTESIAN_POINT ( 'NONE',  ( -23.94331431717321834, 0.4798011554587169325, -19.49553339312929268 ) ) ;
#25628=CARTESIAN_POINT ( 'NONE',  ( 20.72609593855841581, -1.618474817249470954, -27.28862543018874121 ) ) ;
#25629=CARTESIAN_POINT ( 'NONE',  ( 20.37075632078805398, -2.330628970618247919, -29.99999999999998224 ) ) ;
#25645=CARTESIAN_POINT ( 'NONE',  ( -23.10177455024117776, 8.837490529234450776, -9.870891380885264965 ) ) ;
#25647=CARTESIAN_POINT ( 'NONE',  ( 13.26265854479622419, -15.63203989815269779, -29.99999999999999289 ) ) ;
#25650=CARTESIAN_POINT ( 'NONE',  ( 13.67698555827839968, 23.60253768574900946, -14.45466942440959635 ) ) ;
#25652=CARTESIAN_POINT ( 'NONE',  ( -14.83746131866766405, 24.15353679605524562, -11.62345532500183864 ) ) ;
#25655=CARTESIAN_POINT ( 'NONE',  ( 12.96000418219073858, 21.60184555869381384, -17.44299700738821812 ) ) ;
#25657=CARTESIAN_POINT ( 'NONE',  ( 32.54628837895766935, -17.94405776258001239, -8.843653535525763942 ) ) ;
#25660=CARTESIAN_POINT ( 'NONE',  ( -11.06077501432392651, 18.23000144808903755, -24.98034412766138956 ) ) ;
#25662=CARTESIAN_POINT ( 'NONE',  ( -12.84304827169525964, -22.01029806000802935, -17.37299228019244879 ) ) ;
#25665=CARTESIAN_POINT ( 'NONE',  ( -30.61059542336693085, -12.61261197708686588, -12.91721441924257974 ) ) ;
#25666=CARTESIAN_POINT ( 'NONE',  ( -13.49856781751322110, -24.92574764376128371, -11.62344980891660740 ) ) ;
#25668=CARTESIAN_POINT ( 'NONE',  ( 14.84856562538137403, 21.17331135784270657, -14.60805661069002781 ) ) ;
#25670=CARTESIAN_POINT ( 'NONE',  ( 27.04882373375960825, 3.777209956746526043, -8.341230441078749891 ) ) ;
#25677=CARTESIAN_POINT ( 'NONE',  ( -21.00158985414197588, 0.4703539060713058384, -26.19501892574664481 ) ) ;
#25678=CARTESIAN_POINT ( 'NONE',  ( 26.15888819988984437, -0.1763494521739284449, -16.38123973257840760 ) ) ;
#25679=VECTOR ( 'NONE', #22498, 1000.000000000000000 ) ;
#25684=CARTESIAN_POINT ( 'NONE',  ( 16.77267017469755217, -29.13948811618736912, -5.000000000000000888 ) ) ;
#25693=ORIENTED_EDGE ( 'NONE', *, *, #7911, .T. ) ;
#25696=CARTESIAN_POINT ( 'NONE',  ( 25.94815390757270634, -24.00269173140258872, -9.783439592027228571 ) ) ;
#25700=CARTESIAN_POINT ( 'NONE',  ( 14.53483714358199919, 25.97957738232134872, -10.61578658074032333 ) ) ;
#25703=CARTESIAN_POINT ( 'NONE',  ( -15.23813856142597167, 17.31405161251928249, -18.82644271334805453 ) ) ;
#25708=CARTESIAN_POINT ( 'NONE',  ( 15.25374212246388694, -26.48790319330748133, -7.358088638680141180 ) ) ;
#25710=CARTESIAN_POINT ( 'NONE',  ( 13.76937081925355955, 23.39622061500657324, -14.47626747317092466 ) ) ;
#25712=CARTESIAN_POINT ( 'NONE',  ( 11.17466575968340692, 17.76334817009650635, -26.22383286113582201 ) ) ;
#25714=CARTESIAN_POINT ( 'NONE',  ( -15.34454670589055603, 26.76954483690364839, -6.415642936482374381 ) ) ;
#25716=CARTESIAN_POINT ( 'NONE',  ( -9.469408548107701051, -18.18187935292228019, -29.34893421946817682 ) ) ;
#25718=CARTESIAN_POINT ( 'NONE',  ( -26.62430720910999682, -18.39156676930381451, -13.81496718408933333 ) ) ;
#25719=CARTESIAN_POINT ( 'NONE',  ( -4.703611708043858641, -24.60377627214949925, -8.882725814672168596 ) ) ;
#25720=CARTESIAN_POINT ( 'NONE',  ( 11.42783708703505852, 17.06964071376472702, -28.72407638117795514 ) ) ;
#25722=CARTESIAN_POINT ( 'NONE',  ( 22.52668103003253464, 8.989979787406557676, -11.86183922785617462 ) ) ;
#25727=CARTESIAN_POINT ( 'NONE',  ( -28.14360955461928171, -2.773391863289171866, -15.14227585713986812 ) ) ;
#25733=CARTESIAN_POINT ( 'NONE',  ( 19.13306659232624085, -8.411872202393357867, -26.98792224631750258 ) ) ;
#25739=CARTESIAN_POINT ( 'NONE',  ( -27.20167217120908632, 3.999461679458497620, -5.000000000000001776 ) ) ;
#25744=CARTESIAN_POINT ( 'NONE',  ( -0.7539017812582481382, 38.52547057370831141, -5.000000000000002665 ) ) ;
#25750=CARTESIAN_POINT ( 'NONE',  ( 9.326849233417362939, 18.43685803866042150, -27.97763387032424731 ) ) ;
#25754=CARTESIAN_POINT ( 'NONE',  ( -19.54739990906080394, 14.10301885897343155, -11.87122386020018006 ) ) ;
#25757=CARTESIAN_POINT ( 'NONE',  ( 15.14825655869951682, -26.16207617773802596, -8.764898773645015240 ) ) ;
#25759=CARTESIAN_POINT ( 'NONE',  ( 15.21391305131906080, 26.46934913501528541, -7.825681926150065415 ) ) ;
#25760=CARTESIAN_POINT ( 'NONE',  ( -37.62663912510979003, -8.659558992827880886, -14.26382729546507555 ) ) ;
#25763=CARTESIAN_POINT ( 'NONE',  ( -25.31025310574754883, -25.23397962983047194, -8.474964599348188798 ) ) ;
#25764=CARTESIAN_POINT ( 'NONE',  ( 5.866761025329905621, -24.11837628505799458, -11.82181453652845882 ) ) ;
#25765=CARTESIAN_POINT ( 'NONE',  ( 15.37647888069712465, 26.23441537448958272, -7.358884453500203371 ) ) ;
#25766=CARTESIAN_POINT ( 'NONE',  ( 25.27966917872702624, -18.27353908186211839, -14.74917764330799308 ) ) ;
#25767=DIRECTION ( 'NONE',  ( 1.000000000000000000, 0.000000000000000000, 0.000000000000000000 ) ) ;
#25771=CARTESIAN_POINT ( 'NONE',  ( -7.233295743329782646, 30.62580296063414309, -13.90069797551026021 ) ) ;
#25779=CARTESIAN_POINT ( 'NONE',  ( 30.01319108853827444, 0.005912998638344907354, -9.238060575309988920 ) ) ;
#25783=CARTESIAN_POINT ( 'NONE',  ( -23.28487554430953566, 0.6417891521472164351, -20.55291216075323391 ) ) ;
#25786=CARTESIAN_POINT ( 'NONE',  ( 26.20077895376393684, -6.234191634555112493, -17.82519732595303452 ) ) ;
#25799=CARTESIAN_POINT ( 'NONE',  ( -9.103489325454093617, 18.41553740122394345, -29.99999999999998224 ) ) ;
#25803=CARTESIAN_POINT ( 'NONE',  ( 16.07357205507025100, 16.08392265437850810, -18.91655558039364848 ) ) ;
#25805=CARTESIAN_POINT ( 'NONE',  ( 10.90692232337486445, 34.26194292751238635, -4.999999999999999112 ) ) ;
#25809=CARTESIAN_POINT ( 'NONE',  ( 15.35372630195935706, -25.59917946473734673, -10.60842069110901598 ) ) ;
#25812=ORIENTED_EDGE ( 'NONE', *, *, #12493, .F. ) ;
#25813=CARTESIAN_POINT ( 'NONE',  ( -15.02832875975274973, 25.93642894353117256, -9.238718023697360948 ) ) ;
#25815=CARTESIAN_POINT ( 'NONE',  ( 9.727620666417239548, -18.90945770702390760, -25.04146322545150483 ) ) ;
#25817=EDGE_LOOP ( 'NONE', ( #5190, #38184, #19359, #26052, #15532, #10952 ) ) ;
#25819=CARTESIAN_POINT ( 'NONE',  ( -9.245618777199831939, 19.45120513334818568, -24.74765325802571780 ) ) ;
#25822=CARTESIAN_POINT ( 'NONE',  ( -20.69933004820033773, -5.104132961445666972, -25.75960008462992334 ) ) ;
#25825=CARTESIAN_POINT ( 'NONE',  ( 28.18869082171447005, 0.3296785013067420889, -12.55904125333466936 ) ) ;
#25830=CARTESIAN_POINT ( 'NONE',  ( -20.81701148534373047, 0.8134213727834409546, -26.82927742226364032 ) ) ;
#25832=ORIENTED_EDGE ( 'NONE', *, *, #16239, .F. ) ;
#25833=CARTESIAN_POINT ( 'NONE',  ( 31.50878031485120090, -2.153655980402962467, -9.579608105637024806 ) ) ;
#25835=CARTESIAN_POINT ( 'NONE',  ( 20.32885146017839517, -2.671174122295890907, -29.99999999999998224 ) ) ;
#25839=FACE_BOUND ( 'NONE', #37810, .T. ) ;
#25847=CARTESIAN_POINT ( 'NONE',  ( -19.61511227469957319, 7.169619886183266289, -25.45877017602282777 ) ) ;
#25848=CARTESIAN_POINT ( 'NONE',  ( 12.77972917816505927, -16.04224856310990432, -29.27848096932829947 ) ) ;
#25849=CARTESIAN_POINT ( 'NONE',  ( -13.29635151280775140, -18.15191941048946589, -20.55813556249457008 ) ) ;
#25851=CARTESIAN_POINT ( 'NONE',  ( 11.56078434465998761, 19.03143594125964455, -22.71333681129807402 ) ) ;
#25853=CARTESIAN_POINT ( 'NONE',  ( -14.80615464364070810, 23.19894269259860664, -12.60008722521619262 ) ) ;
#25856=CARTESIAN_POINT ( 'NONE',  ( 12.69837305591254761, 20.98788295457261555, -18.46001444634856625 ) ) ;
#25858=CARTESIAN_POINT ( 'NONE',  ( 19.27955278168219522, -10.63738015878406351, -24.21943841340187831 ) ) ;
#25861=CARTESIAN_POINT ( 'NONE',  ( -14.96091455162279438, 26.58795068034906350, -8.747906387789663896 ) ) ;
#25863=CARTESIAN_POINT ( 'NONE',  ( -9.695417275021851466, -18.21019213846330231, -28.07041747300570833 ) ) ;
#25866=CARTESIAN_POINT ( 'NONE',  ( -23.41415742069401773, -10.51963480729080835, -19.65694573768750786 ) ) ;
#25867=CARTESIAN_POINT ( 'NONE',  ( -12.95131304720365328, -24.45778571613171692, -12.59044498358920272 ) ) ;
#25869=CARTESIAN_POINT ( 'NONE',  ( 16.18703989492556872, 19.32897852544927275, -13.73088434759361220 ) ) ;
#25871=CARTESIAN_POINT ( 'NONE',  ( 21.71166764932993232, 3.770909521622002547, -21.95419646536155511 ) ) ;
#25874=DIRECTION ( 'NONE',  ( -0.000000000000000000, -0.000000000000000000, -1.000000000000000000 ) ) ;
#25876=CARTESIAN_POINT ( 'NONE',  ( -30.36316148021155570, -0.1792145421230325053, -8.756721400621293228 ) ) ;
#25878=CARTESIAN_POINT ( 'NONE',  ( 30.28562270265240031, -0.4997343038466697807, -9.672258859702814959 ) ) ;
#25883=EDGE_CURVE ( 'NONE', #35629, #26123, #26087, .T. ) ;
#25884=CARTESIAN_POINT ( 'NONE',  ( -6.155076441694329326, 21.71698211341365337, -20.11584339644705111 ) ) ;
#25896=CARTESIAN_POINT ( 'NONE',  ( 24.68240227516114871, -21.51021177795922412, -12.94802666595622398 ) ) ;
#25899=CARTESIAN_POINT ( 'NONE',  ( 14.59657937566097274, 26.31754401214214667, -10.13852064072044712 ) ) ;
#25903=CARTESIAN_POINT ( 'NONE',  ( -15.45883816434331592, 17.67526787779760866, -17.78974814387579428 ) ) ;
#25905=CARTESIAN_POINT ( 'NONE',  ( 15.38966896450798316, -26.64286542733805163, -6.417027897479346876 ) ) ;
#25907=CARTESIAN_POINT ( 'NONE',  ( 15.42339932183901752, 26.75673767418847859, -5.474198080818684531 ) ) ;
#25909=CARTESIAN_POINT ( 'NONE',  ( 15.17329373222789357, 26.28549969035448086, -8.297710605404072126 ) ) ;
#25913=CARTESIAN_POINT ( 'NONE',  ( -11.07661461107485046, 17.64654016112482182, -26.82585402569723954 ) ) ;
#25915=CARTESIAN_POINT ( 'NONE',  ( -14.92943112510105053, -25.97912449464955387, -9.238937178076628953 ) ) ;
#25917=CARTESIAN_POINT ( 'NONE',  ( -32.94090784223518398, -19.89252564384590016, -5.855569924352811206 ) ) ;
#25918=CARTESIAN_POINT ( 'NONE',  ( -6.958230700871959051, -24.96871470505583090, -7.888467374285714762 ) ) ;
#25919=CARTESIAN_POINT ( 'NONE',  ( 11.71780135332492634, 17.71433433733627538, -25.06800478147926725 ) ) ;
#25921=CARTESIAN_POINT ( 'NONE',  ( 23.41645241902980601, 8.181230565227640028, -10.35730366361351074 ) ) ;
#25923=CARTESIAN_POINT ( 'NONE',  ( -5.023663292579894524, -24.92826071503396790, -5.000000000000000888 ) ) ;
#25926=CARTESIAN_POINT ( 'NONE',  ( -31.91632926199020659, -2.416287452245505118, -9.107245833971825633 ) ) ;
#25932=CARTESIAN_POINT ( 'NONE',  ( 31.89048545145299585, -15.10830598425978266, -11.07426897462641513 ) ) ;
#25942=CARTESIAN_POINT ( 'NONE',  ( -0.7005653291773012992, 35.42634926839502185, -11.06665404971477784 ) ) ;
#25949=CARTESIAN_POINT ( 'NONE',  ( 14.11003552855667209, 29.50458854998396419, -7.283368533493259633 ) ) ;
#25952=CARTESIAN_POINT ( 'NONE',  ( -19.97103809025421484, 14.46599866876007034, -8.894276274733421417 ) ) ;
#25955=CARTESIAN_POINT ( 'NONE',  ( 10.57564039356294572, -19.56442984277105168, -22.72982311932152655 ) ) ;
#25957=CARTESIAN_POINT ( 'NONE',  ( 15.31881962885621640, 26.68583777872107632, -6.886503466024833209 ) ) ;
#25958=CARTESIAN_POINT ( 'NONE',  ( -3.091399026088746727, 22.35909668862748134, -29.99999999999999289 ) ) ;
#25959=FACE_OUTER_BOUND ( 'NONE', #25817, .T. ) ;
#25960=CARTESIAN_POINT ( 'NONE',  ( -19.03618297789652303, -16.83210767772735750, -19.74809521649639521 ) ) ;
#25961=CARTESIAN_POINT ( 'NONE',  ( 5.670805767156023691, -19.83282806932450271, -28.23774505010902303 ) ) ;
#25962=CARTESIAN_POINT ( 'NONE',  ( 12.48668498222315826, 20.36467295304646186, -19.51308572712811795 ) ) ;
#25963=CARTESIAN_POINT ( 'NONE',  ( 17.14480940267289455, 11.33456439865563148, -28.29661424734811348 ) ) ;
#25968=CARTESIAN_POINT ( 'NONE',  ( -9.332086639220589674, 35.22756758965231683, -6.737663000051229645 ) ) ;
#25973=CARTESIAN_POINT ( 'NONE',  ( 27.75798668795975743, 0.1628108966169759808, -13.51197211289437305 ) ) ;
#25975=CARTESIAN_POINT ( 'NONE',  ( 10.98647152928294446, 17.30743895948372213, -29.99999999999999289 ) ) ;
#25979=CARTESIAN_POINT ( 'NONE',  ( -29.26835155205951366, 0.1731288304656850296, -10.65622225438751691 ) ) ;
#25981=CARTESIAN_POINT ( 'NONE',  ( 24.30836135983651758, -6.551983109444438291, -19.83190686569865946 ) ) ;
#25994=CARTESIAN_POINT ( 'NONE',  ( 40.48557158514985588, -11.25000000000009415, 3.000000000000000000 ) ) ;
#25999=CARTESIAN_POINT ( 'NONE',  ( 14.27219392008591292, 14.71651433334269043, -30.00000000000000711 ) ) ;
#26000=CARTESIAN_POINT ( 'NONE',  ( 10.72270391973751558, 33.55271709729109375, -8.067294441686739148 ) ) ;
#26001=VERTEX_POINT ( 'NONE', #30755 ) ;
#26004=CARTESIAN_POINT ( 'NONE',  ( 12.10068356543891710, -20.90411770709192041, -19.42675082364999639 ) ) ;
#26008=CARTESIAN_POINT ( 'NONE',  ( -14.03186475831749647, 23.92943759979809570, -13.51384694048713619 ) ) ;
#26011=CARTESIAN_POINT ( 'NONE',  ( 9.462549223031706092, -18.54705810577948455, -26.84942688299948799 ) ) ;
#26016=CARTESIAN_POINT ( 'NONE',  ( -8.851921390983532589, 18.49121495627866452, -29.30371079639624909 ) ) ;
#26017=CARTESIAN_POINT ( 'NONE',  ( -13.16997834948020873, -17.85564821404134150, -23.48525574773325886 ) ) ;
#26020=CARTESIAN_POINT ( 'NONE',  ( -28.17101914744512925, -6.941970696622886905, -15.85777330802162055 ) ) ;
#26023=CARTESIAN_POINT ( 'NONE',  ( 25.78250412838150041, 0.4551448022510044544, -16.45580364150897879 ) ) ;
#26025=CARTESIAN_POINT ( 'NONE',  ( 14.32492426577155165, 24.55152792996899080, -12.54456079180045514 ) ) ;
#26029=CARTESIAN_POINT ( 'NONE',  ( -29.37198519057492163, 0.05438766727590542416, -10.65228692739096594 ) ) ;
#26032=CARTESIAN_POINT ( 'NONE',  ( 22.03578752383834072, -1.794605797681862791, -23.55611175985229266 ) ) ;
#26034=CARTESIAN_POINT ( 'NONE',  ( 20.32145253026429188, 2.784070299583892183, -30.00000000000000000 ) ) ;
#26048=CARTESIAN_POINT ( 'NONE',  ( -18.97876558365113553, 7.800091065717492889, -28.85243984144211993 ) ) ;
#26050=CARTESIAN_POINT ( 'NONE',  ( 20.56439459974750150, -26.83426525695362130, -7.688853040980692555 ) ) ;
#26052=ORIENTED_EDGE ( 'NONE', *, *, #11413, .T. ) ;
#26053=CARTESIAN_POINT ( 'NONE',  ( 11.08031616781238782, 17.83112152660168093, -26.21360684684639963 ) ) ;
#26055=CARTESIAN_POINT ( 'NONE',  ( -11.76523398598002323, 16.92967342931978791, -28.11894497090000300 ) ) ;
#26058=CARTESIAN_POINT ( 'NONE',  ( 11.12516802696661067, 17.46729153672471924, -27.45183205712903884 ) ) ;
#26060=CARTESIAN_POINT ( 'NONE',  ( 19.98779029393962503, -11.02768449253182403, -22.98586908969943110 ) ) ;
#26063=CARTESIAN_POINT ( 'NONE',  ( -14.83546550674832432, 26.53435752211777299, -9.210659735667860559 ) ) ;
#26065=CARTESIAN_POINT ( 'NONE',  ( -14.70647767559404784, -24.71655422085136777, -12.49785459478513161 ) ) ;
#26068=CARTESIAN_POINT ( 'NONE',  ( -35.14568626021495845, -14.53237387118475610, -5.437296911868972238 ) ) ;
#26069=CARTESIAN_POINT ( 'NONE',  ( -9.443825133297737651, -18.71410463014245096, -26.25643312767523341 ) ) ;
#26071=CARTESIAN_POINT ( 'NONE',  ( 13.25821341800907227, 15.76719205175851002, -28.19245977045222773 ) ) ;
#26073=CARTESIAN_POINT ( 'NONE',  ( 27.88619785758654857, 2.892813575489728173, -7.853246008088212271 ) ) ;
#26078=CARTESIAN_POINT ( 'NONE',  ( -20.49112616741955506, 0.6095660351776287511, -29.99999999999999645 ) ) ;
#26079=CARTESIAN_POINT ( 'NONE',  ( 30.84690724597788858, -0.7292977086491185812, -8.727067712974493574 ) ) ;
#26083=CARTESIAN_POINT ( 'NONE',  ( -20.48369986121767283, 1.531721084589908966, -28.72957500320905311 ) ) ;
#26084=CARTESIAN_POINT ( 'NONE',  ( -22.40982762235196191, 2.618079236897031148, -29.99999999999999645 ) ) ;
#26087=LINE ( 'NONE', #10866, #16114 ) ;
#26093=EDGE_CURVE ( 'NONE', #20959, #39797, #16150, .T. ) ;
#26097=CARTESIAN_POINT ( 'NONE',  ( 27.17408060449223228, -25.06914451978216718, -6.725518816324792759 ) ) ;
#26101=CARTESIAN_POINT ( 'NONE',  ( 11.77932827439872199, 20.33358996693879561, -20.47140772640445050 ) ) ;
#26104=CARTESIAN_POINT ( 'NONE',  ( -17.34987630490782351, 20.70268335502479928, -6.910411782773334011 ) ) ;
#26107=CARTESIAN_POINT ( 'NONE',  ( 12.20016556335618141, -22.02549961372093179, -17.44539159223752378 ) ) ;
#26110=CARTESIAN_POINT ( 'NONE',  ( 13.77648659466977854, 23.38131483086550944, -14.47688990636883943 ) ) ;
#26112=CARTESIAN_POINT ( 'NONE',  ( 10.97760868008098889, 17.31306259807076131, -30.00000000000000000 ) ) ;
#26113=B_SPLINE_CURVE_WITH_KNOTS ( 'NONE', 3,
 ( #20045, #10092, #13331, #38117, #35277, #7229, #10289, #19630, #4393, #16798, #32026, #4191, #10696, #7639, #32440, #30189, #18202, #8246 ),
 .UNSPECIFIED., .F., .F.,
 ( 4, 2, 2, 2, 2, 2, 2, 2, 4 ),
 ( 0.2985673197444002613, 0.3862464047763500274, 0.4739254898082998491, 0.5616045748402497262, 0.6492836598721997143, 0.7369627449041498135, 0.8246418299360998017, 0.9123209149680500119, 1.000000000000000000 ),
 .UNSPECIFIED. ) ;
#26115=CARTESIAN_POINT ( 'NONE',  ( -15.39213581000993436, 26.86843326188214576, -5.473789308097052775 ) ) ;
#26117=CARTESIAN_POINT ( 'NONE',  ( -14.70529695197427422, -25.64556149301234456, -10.18130632746762920 ) ) ;
#26120=CARTESIAN_POINT ( 'NONE',  ( -17.43379632413495983, -11.24738337999374593, -27.70877160700983310 ) ) ;
#26121=CARTESIAN_POINT ( 'NONE',  ( -2.301023503631009159, -23.23531080007942506, -14.91665611832322114 ) ) ;
#26122=CARTESIAN_POINT ( 'NONE',  ( 14.30052602520593474, 22.28094600777651380, -14.54308252804225887 ) ) ;
#26123=VERTEX_POINT ( 'NONE', #40082 ) ;
#26124=CARTESIAN_POINT ( 'NONE',  ( 18.97764795543955785, 8.024778375806581820, -27.72202992318708681 ) ) ;
#26126=CARTESIAN_POINT ( 'NONE',  ( 10.13720066964783939, -25.55706996539716513, -5.000000000000003553 ) ) ;
#26129=CARTESIAN_POINT ( 'NONE',  ( -25.45953608835651139, -1.714497824024611594, -18.18611588942592405 ) ) ;
#26136=CARTESIAN_POINT ( 'NONE',  ( 34.95664498758854677, -15.33017443246186495, -5.436732254870795700 ) ) ;
#26146=CARTESIAN_POINT ( 'NONE',  ( -0.7484310965467956267, 38.13046687410084701, -7.116911809159399027 ) ) ;
#26148=EDGE_CURVE ( 'NONE', #31785, #8550, #21963, .T. ) ;
#26154=CARTESIAN_POINT ( 'NONE',  ( 10.62820802463951964, 21.51424845583950685, -20.27260820117726681 ) ) ;
#26157=CARTESIAN_POINT ( 'NONE',  ( -19.36646015756375760, 13.94833338277440582, -12.87628227385044433 ) ) ;
#26162=CARTESIAN_POINT ( 'NONE',  ( 15.19304689221615412, -26.28704695153315285, -8.297102716332286576 ) ) ;
#26165=CARTESIAN_POINT ( 'NONE',  ( 15.15493471932264491, 26.34784287548288262, -8.295283454795825406 ) ) ;
#26166=CARTESIAN_POINT ( 'NONE',  ( -11.31392148919591811, 36.91540483778867099, -14.26382729546508088 ) ) ;
#26169=CARTESIAN_POINT ( 'NONE',  ( -25.14789180526689805, -22.31687521175224376, -12.03118656357111860 ) ) ;
#26170=CARTESIAN_POINT ( 'NONE',  ( 7.832614783866235442, -20.65680624402197907, -21.94422844697728792 ) ) ;
#26171=CARTESIAN_POINT ( 'NONE',  ( 12.83367166058087072, 20.79141030706715298, -18.48305212125895736 ) ) ;
#26172=CARTESIAN_POINT ( 'NONE',  ( 18.62263446944652046, 13.67603366424814837, -15.92850824050840863 ) ) ;
#26176=CARTESIAN_POINT ( 'NONE',  ( -7.058933474767617788, 34.49725963336143764, -10.22158782810721256 ) ) ;
#26178=CARTESIAN_POINT ( 'NONE',  ( -14.82146137012738940, -25.95528464061796825, -9.240260087632112374 ) ) ;
#26186=CARTESIAN_POINT ( 'NONE',  ( -20.47826699597012023, 0.9446083685552518761, -29.34992276858810811 ) ) ;
#26188=CARTESIAN_POINT ( 'NONE',  ( 20.72580500889552013, -4.914281886810445421, -25.77267062739201364 ) ) ;
#26199=CARTESIAN_POINT ( 'NONE',  ( -15.93611613685307482, -12.91202363157417565, -30.00000000000004263 ) ) ;
#26203=CARTESIAN_POINT ( 'NONE',  ( 18.59382115548298131, 17.96292538557851515, -5.000000000000004441 ) ) ;
#26204=CARTESIAN_POINT ( 'NONE',  ( 8.607820399192389615, 29.73311969603586746, -13.95432102836428889 ) ) ;
#26210=CARTESIAN_POINT ( 'NONE',  ( 16.27219429315636390, -26.92618254030204383, -5.470502546158905410 ) ) ;
#26214=CARTESIAN_POINT ( 'NONE',  ( -12.64541957868966193, 21.06527240651957200, -18.45049806135583736 ) ) ;
#26217=CARTESIAN_POINT ( 'NONE',  ( 13.95335475392358759, -25.00100328124352345, -11.61047761660894118 ) ) ;
#26221=CARTESIAN_POINT ( 'NONE',  ( -12.42600970353487533, 29.09350466320093531, -11.32961783136679657 ) ) ;
#26225=CARTESIAN_POINT ( 'NONE',  ( -34.94942070055063255, -7.655693536555084222, -6.319957789537046899 ) ) ;
#26228=CARTESIAN_POINT ( 'NONE',  ( 22.17991941591415639, 0.8307563611647147406, -22.75514243441729789 ) ) ;
#26233=CARTESIAN_POINT ( 'NONE',  ( -30.18693267962284565, 0.009138568670973495206, -8.767643421507747448 ) ) ;
#26237=CARTESIAN_POINT ( 'NONE',  ( 33.67507661585143808, -4.155749373709020311, -6.800351445119964033 ) ) ;
#26239=CARTESIAN_POINT ( 'NONE',  ( 17.61751615880474020, 10.50706712441501978, -29.99999999999999645 ) ) ;
#26250=CIRCLE ( 'NONE', #28837, 17.00000000000000355 ) ;
#26251=CARTESIAN_POINT ( 'NONE',  ( 4.942291792648391358, 37.16033961302324684, -7.558059442438699982 ) ) ;
#26255=CARTESIAN_POINT ( 'NONE',  ( -22.10434164247800481, 10.70873872237885394, -8.898544400284965405 ) ) ;
#26256=CARTESIAN_POINT ( 'NONE',  ( 21.54393101763996654, -26.56854998837850701, -8.110961036857599282 ) ) ;
#26261=CARTESIAN_POINT ( 'NONE',  ( 10.98519287105149544, 17.56129497315728827, -27.44095920151953649 ) ) ;
#26264=CARTESIAN_POINT ( 'NONE',  ( -15.66962402360438666, 25.81090189859874684, -5.946396493405305961 ) ) ;
#26267=CYLINDRICAL_SURFACE ( 'NONE', #14667, 56.99999999999991473 ) ;
#26268=CARTESIAN_POINT ( 'NONE',  ( 15.44688523099049959, 26.67261462138580441, -5.000000000000000000 ) ) ;
#26270=CARTESIAN_POINT ( 'NONE',  ( 33.65939441685168276, -18.56364632560252304, -5.855820354545722140 ) ) ;
#26272=CARTESIAN_POINT ( 'NONE',  ( -14.59220174411789017, 25.82205283844941590, -10.62570393986304396 ) ) ;
#26273=CARTESIAN_POINT ( 'NONE',  ( 3.863783140547853712E-14, -86.77689918168233874, -5.000000000000000000 ) ) ;
#26274=CARTESIAN_POINT ( 'NONE',  ( -11.32539160478685858, -19.87450722000827241, -21.55174846688731805 ) ) ;
#26277=CARTESIAN_POINT ( 'NONE',  ( -33.95062610603429221, -14.00321741133104148, -8.861547101450529595 ) ) ;
#26278=CARTESIAN_POINT ( 'NONE',  ( -9.862602973713741505, -19.28908076663119076, -23.89725503471435530 ) ) ;
#26280=CARTESIAN_POINT ( 'NONE',  ( 16.96835065415153210, 20.59718713987552263, -9.315625699485860167 ) ) ;
#26282=CARTESIAN_POINT ( 'NONE',  ( 26.93411999856199301, 3.776180714121243565, -8.821889400297479256 ) ) ;
#26287=CARTESIAN_POINT ( 'NONE',  ( -27.88474080230812646, -0.0008730228811752835556, -13.49305137967154344 ) ) ;
#26290=CARTESIAN_POINT ( 'NONE',  ( 28.89633671753446009, -0.5709352303838933773, -12.48089840086014668 ) ) ;
#26293=CARTESIAN_POINT ( 'NONE',  ( -28.33534295838423844, 2.626085861103411023, -6.423780397466612335 ) ) ;
#26295=CARTESIAN_POINT ( 'NONE',  ( 15.29245034862073283, 32.56469986092002955, -4.999999999999995559 ) ) ;
#26302=CARTESIAN_POINT ( 'NONE',  ( -20.23296131041716706, 28.12381335138030636, 0.000000000000000000 ) ) ;
#26309=CARTESIAN_POINT ( 'NONE',  ( 16.06823390034044152, -13.10808670322615832, -27.74124904695872473 ) ) ;
#26312=CARTESIAN_POINT ( 'NONE',  ( 15.17508192504865683, 27.32470433355475237, -6.406894672669320556 ) ) ;
#26315=CARTESIAN_POINT ( 'NONE',  ( -14.49642055680277331, 14.68297716386891594, -27.65792624604139860 ) ) ;
#26317=CARTESIAN_POINT ( 'NONE',  ( 14.55400969869553229, -25.44726499792421492, -10.65473343070086010 ) ) ;
#26319=CARTESIAN_POINT ( 'NONE',  ( 11.19624587173573893, 17.74773942844264596, -26.22615366399902470 ) ) ;
#26320=ORIENTED_EDGE ( 'NONE', *, *, #968, .F. ) ;
#26321=CARTESIAN_POINT ( 'NONE',  ( 15.10138251737948600, 26.13808434145718351, -8.767643565617396106 ) ) ;
#26323=CARTESIAN_POINT ( 'NONE',  ( -13.16545571440353335, 22.31697612090500016, -16.43388903272470714 ) ) ;
#26325=CARTESIAN_POINT ( 'NONE',  ( -13.01110499904087980, -23.09146633989079334, -15.45099639591618690 ) ) ;
#26329=CARTESIAN_POINT ( 'NONE',  ( -22.52291761385160740, -14.54607051226803449, -18.61927420860634541 ) ) ;
#26330=CARTESIAN_POINT ( 'NONE',  ( -6.891701031399811050, -24.81840269475382499, -8.859753654562227965 ) ) ;
#26331=CARTESIAN_POINT ( 'NONE',  ( 11.63255956027453841, 17.11425915239349393, -27.48977356258791360 ) ) ;
#26332=EDGE_LOOP ( 'NONE', ( #4489, #22679 ) ) ;
#26333=CARTESIAN_POINT ( 'NONE',  ( 18.88780196539459055, 8.001059241770983377, -29.99999999999999645 ) ) ;
#26335=CARTESIAN_POINT ( 'NONE',  ( -15.47933092437222768, -26.74032362632396342, -5.000000000000000888 ) ) ;
#26338=CARTESIAN_POINT ( 'NONE',  ( -29.45776514400509072, -1.389050121157273665, -12.41183737987973323 ) ) ;
#26345=CARTESIAN_POINT ( 'NONE',  ( 23.21470675034833775, -11.03075323633567528, -19.64526940384888576 ) ) ;
#26347=ORIENTED_EDGE ( 'NONE', *, *, #9131, .T. ) ;
#26353=CARTESIAN_POINT ( 'NONE',  ( 1.195900963322536814, 29.06378828199482101, -16.62768215971903984 ) ) ;
#26356=CARTESIAN_POINT ( 'NONE',  ( 3.485571585149869200, -11.24999999999998224, 0.000000000000000000 ) ) ;
#26357=CARTESIAN_POINT ( 'NONE',  ( 34.47241746879583957, 3.460351812918713854, 0.000000000000000000 ) ) ;
#26360=CARTESIAN_POINT ( 'NONE',  ( 11.80513401506518001, 23.30479376290859506, -17.22064554265607228 ) ) ;
#26363=CARTESIAN_POINT ( 'NONE',  ( -17.52657988488712704, 12.36839558647593051, -22.23037286673406143 ) ) ;
#26366=CARTESIAN_POINT ( 'NONE',  ( 9.523339034571952411, -18.15368110581538019, -30.00000000000000000 ) ) ;
#26368=CARTESIAN_POINT ( 'NONE',  ( 14.99969651570772378, 26.02920516864225675, -9.235286274286707453 ) ) ;
#26369=CARTESIAN_POINT ( 'NONE',  ( -37.49625565938783467, -14.69322820095469240, -5.000000000000006217 ) ) ;
#26371=CARTESIAN_POINT ( 'NONE',  ( -27.87119330683370677, -24.65308250635607479, -6.720147514500800057 ) ) ;
#26372=CARTESIAN_POINT ( 'NONE',  ( 3.491862997321047324, -22.96065156239022897, -15.91807752016459432 ) ) ;
#26373=CARTESIAN_POINT ( 'NONE',  ( 15.36189083411322187, 25.97148884136161939, -7.830196362163139412 ) ) ;
#26374=CARTESIAN_POINT ( 'NONE',  ( 20.43196929446886401, 13.86938077394290580, -7.915868592357410805 ) ) ;
#26377=CARTESIAN_POINT ( 'NONE',  ( -6.250014167710259194, 36.16780209143936986, -8.434276216203160814 ) ) ;
#26380=ORIENTED_EDGE ( 'NONE', *, *, #20817, .T. ) ;
#26385=CARTESIAN_POINT ( 'NONE',  ( -25.80299850805823425, 0.4204530589918408223, -16.45275957436017933 ) ) ;
#26387=CARTESIAN_POINT ( 'NONE',  ( 34.97939493771907848, -10.55727357374866493, -7.588994557062878954 ) ) ;
#26402=CARTESIAN_POINT ( 'NONE',  ( 18.78138322832032969, 16.61749776086161035, -9.368813598564180722 ) ) ;
#26403=AXIS2_PLACEMENT_3D ( 'NONE', #11105, #16596, #38929 ) ;
#26404=CARTESIAN_POINT ( 'NONE',  ( 10.84964834875164463, 34.03396980005788919, -6.755589542877508791 ) ) ;
#26411=CARTESIAN_POINT ( 'NONE',  ( 12.67954175781115822, -22.01374323132807476, -17.39205990358088272 ) ) ;
#26412=CARTESIAN_POINT ( 'NONE',  ( 19.48557158514975285, -11.24999999999995737, 6.000000000000000000 ) ) ;
#26417=CARTESIAN_POINT ( 'NONE',  ( -15.40573053741202791, 26.82015453055286969, -5.000000000000001776 ) ) ;
#26419=CARTESIAN_POINT ( 'NONE',  ( 12.39246001483761539, -23.54175171672831723, -14.52989995892280106 ) ) ;
#26423=CARTESIAN_POINT ( 'NONE',  ( -12.61462386970939775, 32.22368281794742018, -6.341505710337779433 ) ) ;
#26426=CARTESIAN_POINT ( 'NONE',  ( -23.48166808057901989, -5.066536945620522481, -20.99526510558111170 ) ) ;
#26429=CARTESIAN_POINT ( 'NONE',  ( 20.68909164424603730, 0.9095261957111510087, -27.45237514931904954 ) ) ;
#26434=CARTESIAN_POINT ( 'NONE',  ( -27.15853788013058079, 0.2099631823020539356, -14.47428761516277618 ) ) ;
#26438=CARTESIAN_POINT ( 'NONE',  ( 20.73891562577072634, -0.9609881625880122291, -27.33083722918737735 ) ) ;
#26451=CARTESIAN_POINT ( 'NONE',  ( 4.986586119666859496, 37.59550631332245985, -6.283304853315398120 ) ) ;
#26455=CARTESIAN_POINT ( 'NONE',  ( 12.14263327931022474, -17.31510639158323173, -25.99352023739256623 ) ) ;
#26461=CARTESIAN_POINT ( 'NONE',  ( 15.13632466973338353, 26.41015704048310297, -8.292868291921246637 ) ) ;
#26464=CARTESIAN_POINT ( 'NONE',  ( -13.03586472630768078, 20.49849890579186962, -18.51679387589177139 ) ) ;
#26468=CARTESIAN_POINT ( 'NONE',  ( 14.77255199613913739, 25.29418844797250898, -10.65547838526898694 ) ) ;
#26470=CARTESIAN_POINT ( 'NONE',  ( 17.54066805493992121, -11.09882095461065710, -27.70640768852350888 ) ) ;
#26471=B_SPLINE_CURVE_WITH_KNOTS ( 'NONE', 3,
 ( #14179, #33290, #17652, #5632, #2399, #23929 ),
 .UNSPECIFIED., .F., .F.,
 ( 4, 2, 4 ),
 ( 0.000000000000000000, 0.5000000000000001110, 1.000000000000000000 ),
 .UNSPECIFIED. ) ;
#26474=CARTESIAN_POINT ( 'NONE',  ( -13.77510122325607789, 24.52954501137963916, -13.45804258254887209 ) ) ;
#26476=CARTESIAN_POINT ( 'NONE',  ( -10.52265961525695559, -18.21930999212262137, -26.15301577430472335 ) ) ;
#26481=CARTESIAN_POINT ( 'NONE',  ( -34.66916150951502829, -13.09694564545405626, -7.995340687606282692 ) ) ;
#26482=CARTESIAN_POINT ( 'NONE',  ( -10.85943135922135561, -20.52714661791293338, -20.57883059674998805 ) ) ;
#26484=CARTESIAN_POINT ( 'NONE',  ( 16.54809703417162225, 21.62887500659449103, -9.299666550987730318 ) ) ;
#26486=CARTESIAN_POINT ( 'NONE',  ( 20.51437803745783484, 4.510445312378868365, -25.33195205685563423 ) ) ;
#26490=CARTESIAN_POINT ( 'NONE',  ( -20.61986670983709402, 0.6792029499141194471, -28.06894698849345460 ) ) ;
#26492=CARTESIAN_POINT ( 'NONE',  ( 23.48977253511795737, 0.06509944194096961567, -20.47537068515592296 ) ) ;
#26495=ORIENTED_EDGE ( 'NONE', *, *, #4858, .F. ) ;
#26496=CARTESIAN_POINT ( 'NONE',  ( -23.30533847871739184, 2.001508224256452362, -19.66258829786930562 ) ) ;
#26497=CARTESIAN_POINT ( 'NONE',  ( 16.84920187454417828, 29.09530251867925443, -5.000000000000000000 ) ) ;
#26509=CARTESIAN_POINT ( 'NONE',  ( -26.14285255608131209, 5.307274672128771797, -6.434788150531786322 ) ) ;
#26512=CARTESIAN_POINT ( 'NONE',  ( 28.04695191141788158, -24.37772861669491320, -7.143925439455689030 ) ) ;
#26518=CARTESIAN_POINT ( 'NONE',  ( 11.89959718257016164, 20.19666440959803921, -20.49464208040282642 ) ) ;
#26519=DIRECTION ( 'NONE',  ( 1.000000000000000000, 0.000000000000000000, 0.000000000000000000 ) ) ;
#26521=CARTESIAN_POINT ( 'NONE',  ( -13.39027686378713788, 15.57931273310112985, -28.79240298120324226 ) ) ;
#26523=CARTESIAN_POINT ( 'NONE',  ( 9.583578724557431983, -18.35907664999004396, -27.45048110621220872 ) ) ;
#26525=CARTESIAN_POINT ( 'NONE',  ( 11.31934672680579723, 18.03076597873480935, -25.01582983836050644 ) ) ;
#26529=CARTESIAN_POINT ( 'NONE',  ( -10.95814459664155294, 17.32538844660855659, -29.99999999999999645 ) ) ;
#26531=CARTESIAN_POINT ( 'NONE',  ( -11.96823149460782254, -21.48079789499611536, -18.44457378902819400 ) ) ;
#26534=CARTESIAN_POINT ( 'NONE',  ( -20.72646010994916210, -13.37970267315822781, -20.69910896450166149 ) ) ;
#26535=CARTESIAN_POINT ( 'NONE',  ( -6.348761669075202008, -23.58403035214085008, -13.80701084941673606 ) ) ;
#26536=CARTESIAN_POINT ( 'NONE',  ( 11.55093992908412126, 16.93669310835906572, -29.36020701913010456 ) ) ;
#26538=CARTESIAN_POINT ( 'NONE',  ( 19.51861134948594056, 7.376813021019582806, -25.46285920900043109 ) ) ;
#26539=CARTESIAN_POINT ( 'NONE',  ( 17.34253826607186255, 27.32041144404028543, -5.000000000000000000 ) ) ;
#26544=CARTESIAN_POINT ( 'NONE',  ( -32.63376561907040951, -2.508419813268226939, -7.282485175223003537 ) ) ;
#26552=CARTESIAN_POINT ( 'NONE',  ( 34.23814126792781565, -17.55187814006816538, -5.435598090313549235 ) ) ;
#26553=CARTESIAN_POINT ( 'NONE',  ( -19.48557158514985588, -11.25000000000002309, 6.000000000000000000 ) ) ;
#26560=CARTESIAN_POINT ( 'NONE',  ( 1.576739634193316197, 38.46478598617967748, -5.000000000000004441 ) ) ;
#26566=CARTESIAN_POINT ( 'NONE',  ( 12.28075117147713513, 22.65327156252982022, -17.30410852053039861 ) ) ;
#26569=CARTESIAN_POINT ( 'NONE',  ( -16.87192496629801397, 11.79917111600507162, -27.72865834311171795 ) ) ;
#26572=CARTESIAN_POINT ( 'NONE',  ( 11.56771891837488120, -20.97406469625146386, -19.49405188942785117 ) ) ;
#26574=CARTESIAN_POINT ( 'NONE',  ( 11.87119298004463097, 19.40464818915105383, -21.61300753313285128 ) ) ;
#26575=CARTESIAN_POINT ( 'NONE',  ( 6.155076441694339096, 21.71698211341367468, -20.11584339644708308 ) ) ;
#26577=CARTESIAN_POINT ( 'NONE',  ( -15.37450020624324232, -14.42786494016273124, -26.36729165574789491 ) ) ;
#26578=CARTESIAN_POINT ( 'NONE',  ( 3.990328747834301915, -24.74414097261287537, -7.420647813714800201 ) ) ;
#26579=CARTESIAN_POINT ( 'NONE',  ( 15.41962056465840369, 26.08857641750358880, -7.359439485418601379 ) ) ;
#26580=CARTESIAN_POINT ( 'NONE',  ( 21.03405174098776342, 12.96318115116885394, -6.940238061123360502 ) ) ;
#26583=CARTESIAN_POINT ( 'NONE',  ( -6.386588552221052595, 37.17016244130430636, -4.999999999999996447 ) ) ;
#26589=DIRECTION ( 'NONE',  ( -0.000000000000000000, -0.000000000000000000, -1.000000000000000000 ) ) ;
#26592=CARTESIAN_POINT ( 'NONE',  ( -30.19789697583199839, 0.4197591680151108728, -7.359975557626077247 ) ) ;
#26594=CARTESIAN_POINT ( 'NONE',  ( 33.75734116780339633, -10.15240224287356519, -9.788738968072763669 ) ) ;
#26606=CARTESIAN_POINT ( 'NONE',  ( 16.16724516751253660, 14.83928554355248330, -21.07326466058601611 ) ) ;
#26607=CARTESIAN_POINT ( 'NONE',  ( 10.52168943551277280, 32.83820809845378363, -9.399405207729710554 ) ) ;
#26612=CARTESIAN_POINT ( 'NONE',  ( 15.33699111502133583, -26.20517303025969369, -8.756749650358152337 ) ) ;
#26616=CARTESIAN_POINT ( 'NONE',  ( -13.76002159541111247, 23.41745082153441615, -14.47402975780730117 ) ) ;
#26618=CARTESIAN_POINT ( 'NONE',  ( 9.154532225212971497, -18.83911771395485601, -26.28255396391754672 ) ) ;
#26624=CARTESIAN_POINT ( 'NONE',  ( -7.700672618952613568, 19.08108758880122480, -28.57812135046165736 ) ) ;
#26628=CARTESIAN_POINT ( 'NONE',  ( -22.77417947270713228, -3.486102136050852618, -22.25714798909087833 ) ) ;
#26630=ORIENTED_EDGE ( 'NONE', *, *, #4272, .F. ) ;
#26631=CARTESIAN_POINT ( 'NONE',  ( 30.55543456312852157, 0.04490906986981075405, -7.358140873893511902 ) ) ;
#26632=FACE_OUTER_BOUND ( 'NONE', #25505, .T. ) ;
#26635=UNCERTAINTY_MEASURE_WITH_UNIT (LENGTH_MEASURE( 1.000000000000000082E-05 ), #35352, 'distance_accuracy_value', 'NONE');
#26638=CARTESIAN_POINT ( 'NONE',  ( -30.16151852821994694, 0.03644184463863008039, -8.767989454590962239 ) ) ;
#26641=CARTESIAN_POINT ( 'NONE',  ( 27.72733811610554966, -4.089226208729503043, -16.01998001631908508 ) ) ;
#26653=CARTESIAN_POINT ( 'NONE',  ( 5.661823860689081833, 34.35857903786058642, -11.10029543532181684 ) ) ;
#26658=CARTESIAN_POINT ( 'NONE',  ( 15.48507841534874174, -21.65259304786752992, -17.10787087048629473 ) ) ;
#26664=CARTESIAN_POINT ( 'NONE',  ( 14.48160356497363210, 25.11524105193378631, -11.58817748003706249 ) ) ;
#26666=CARTESIAN_POINT ( 'NONE',  ( -15.47773846523890917, 25.89138777182121842, -7.360181588512314299 ) ) ;
#26669=CARTESIAN_POINT ( 'NONE',  ( 12.18240653381212546, 19.86309505633298400, -20.55012464957514240 ) ) ;
#26672=CARTESIAN_POINT ( 'NONE',  ( 18.20742805688900745, -10.77041048090527475, -26.25434379449587752 ) ) ;
#26675=CARTESIAN_POINT ( 'NONE',  ( -10.58469681223512637, 17.55611623359288131, -29.99999999999999289 ) ) ;
#26677=CARTESIAN_POINT ( 'NONE',  ( -12.80954651559351554, -20.78165554548692739, -19.34070390230921888 ) ) ;
#26680=CARTESIAN_POINT ( 'NONE',  ( -35.48442078681456024, -11.08901139838818040, -5.440863991683305478 ) ) ;
#26681=CARTESIAN_POINT ( 'NONE',  ( -13.47854813221718828, -24.52993117364806608, -12.57113449638200819 ) ) ;
#26683=CARTESIAN_POINT ( 'NONE',  ( 16.67513756147528525, 21.84779437510598754, -8.337953292251496507 ) ) ;
#26685=CARTESIAN_POINT ( 'NONE',  ( 28.38291952110844463, 2.016127822867134878, -8.795360184343094190 ) ) ;
#26689=CARTESIAN_POINT ( 'NONE',  ( -26.02112680601035422, 0.05871972700698699366, -16.41040207964921294 ) ) ;
#26690=CARTESIAN_POINT ( 'NONE',  ( 21.37444128088304041, -0.04091218078597470137, -24.92512316553253271 ) ) ;
#26696=CARTESIAN_POINT ( 'NONE',  ( -20.44235121065545613, 1.535337040937289510, -30.00000000000000000 ) ) ;
#26698=CARTESIAN_POINT ( 'NONE',  ( -22.52744239175981278, -0.1803094636421871677, -30.00000000000000000 ) ) ;
#26702=LINE ( 'NONE', #26302, #27915 ) ;
#26706=CARTESIAN_POINT ( 'NONE',  ( -20.65325954363973793, 5.772693315354555210, -23.19235817845973102 ) ) ;
#26709=CARTESIAN_POINT ( 'NONE',  ( 19.41133145638843871, -19.02227157888451714, -17.76749197532162583 ) ) ;
#26714=CARTESIAN_POINT ( 'NONE',  ( 10.72171203101364867, 17.52793616594421877, -28.69511805704588170 ) ) ;
#26718=CARTESIAN_POINT ( 'NONE',  ( -16.84357371261561198, 21.61857896997960893, -7.862167963560605877 ) ) ;
#26720=DIRECTION ( 'NONE',  ( -0.000000000000000000, -0.000000000000000000, -1.000000000000000000 ) ) ;
#26721=CARTESIAN_POINT ( 'NONE',  ( 10.99531269100861763, 17.30182433700542788, -29.34858954477268611 ) ) ;
#26725=CARTESIAN_POINT ( 'NONE',  ( -11.10439374658453637, 17.81390274193991274, -26.21621397894739403 ) ) ;
#26728=CARTESIAN_POINT ( 'NONE',  ( -9.632883284787542522, -18.33499355343117543, -27.44695152100973701 ) ) ;
#26730=CARTESIAN_POINT ( 'NONE',  ( -32.09753123880218340, -19.38851364860806470, -8.404147750168046827 ) ) ;
#26731=CARTESIAN_POINT ( 'NONE',  ( -5.215330786035433874, -21.06133893932229029, -22.11287648887297408 ) ) ;
#26732=CARTESIAN_POINT ( 'NONE',  ( 15.30762326431969456, 23.80283413495887501, -10.68953207114196680 ) ) ;
#26734=CARTESIAN_POINT ( 'NONE',  ( 19.52319669605035912, 6.624509332748552026, -27.69642029748051471 ) ) ;
#26740=CARTESIAN_POINT ( 'NONE',  ( -22.62547799901289025, -1.388567265765580760, -22.47904496567277022 ) ) ;
#26741=CARTESIAN_POINT ( 'NONE',  ( 27.16112558961255630, 0.2057471714452771827, -14.47458546668211454 ) ) ;
#26752=CARTESIAN_POINT ( 'NONE',  ( 0.2626407527151565779, 24.68515879224474929, -20.69159593321769464 ) ) ;
#26760=CARTESIAN_POINT ( 'NONE',  ( 12.35707315130249562, 23.65243939895810144, -16.27315544969195571 ) ) ;
#26761=CARTESIAN_POINT ( 'NONE',  ( 35.48538791413476190, -11.24999995268670006, -5.000000000000002665 ) ) ;
#26763=CARTESIAN_POINT ( 'NONE',  ( -18.72571766207202160, 17.65421610605874747, -5.960612349730155302 ) ) ;
#26767=CARTESIAN_POINT ( 'NONE',  ( 9.649927930759803374, -18.32663946374046660, -27.44572378285204550 ) ) ;
#26769=CARTESIAN_POINT ( 'NONE',  ( 14.82926489102576184, 25.64310198477804192, -10.17817126611451783 ) ) ;
#26772=ADVANCED_FACE ( 'NONE', ( #19105, #40030 ), #25000, .T. ) ;
#26773=CARTESIAN_POINT ( 'NONE',  ( -26.09240205010872060, -24.51935322919086602, -8.901813507160523997 ) ) ;
#26774=CARTESIAN_POINT ( 'NONE',  ( 3.334020111461103664, -22.39794475360687542, -17.98710033329706803 ) ) ;
#26775=CARTESIAN_POINT ( 'NONE',  ( 14.97853101390886010, 25.19679915242138080, -10.18807554250177816 ) ) ;
#26776=CARTESIAN_POINT ( 'NONE',  ( 17.58948748090468328, 12.74787095466262343, -21.15892960070590334 ) ) ;
#26779=CARTESIAN_POINT ( 'NONE',  ( -7.424996026816661043, 36.56248452709654373, -6.293540445570466879 ) ) ;
#26781=AXIS2_PLACEMENT_3D ( 'NONE', #37449, #31155, #12461 ) ;
#26788=CARTESIAN_POINT ( 'NONE',  ( -20.47628691903608811, 0.9865603022909631425, -30.00000000000000000 ) ) ;
#26792=CARTESIAN_POINT ( 'NONE',  ( 34.00946725009706029, -11.35794860730630162, -9.327975789640845505 ) ) ;
#26804=CARTESIAN_POINT ( 'NONE',  ( -14.16516198183350639, -14.87677494158405977, -30.00000000000001421 ) ) ;
#26809=CARTESIAN_POINT ( 'NONE',  ( 18.41721206756663776, 17.73514788426912858, -8.380454930519549706 ) ) ;
#26811=CARTESIAN_POINT ( 'NONE',  ( 6.908205946113894491, 19.31174812457788548, -30.00000000000000000 ) ) ;
#26814=CARTESIAN_POINT ( 'NONE',  ( -1.829593030691901284E-15, 22.50000000000001066, 3.000000000000000000 ) ) ;
#26816=CARTESIAN_POINT ( 'NONE',  ( 15.94498026452435901, -26.77773472525574405, -6.408825021150274637 ) ) ;
#26818=CARTESIAN_POINT ( 'NONE',  ( 16.24796006241085422, 15.88921519459651144, -21.50719306941225639 ) ) ;
#26819=CARTESIAN_POINT ( 'NONE',  ( -15.16784012994541087, 26.30413795963287527, -8.296983500820855895 ) ) ;
#26822=CARTESIAN_POINT ( 'NONE',  ( 9.319357777823674027, -19.06942296064119802, -25.08597432989563814 ) ) ;
#26826=CARTESIAN_POINT ( 'NONE',  ( -11.56028495311938720, 32.06293909086500094, -8.988039450567926636 ) ) ;
#26832=CARTESIAN_POINT ( 'NONE',  ( 24.52064454744603594, 0.5127890810554470713, -18.46105024167576403 ) ) ;
#26837=CARTESIAN_POINT ( 'NONE',  ( -30.33764259824372900, 0.01140825290230679939, -8.297842417475935761 ) ) ;
#26840=CARTESIAN_POINT ( 'NONE',  ( 25.12025796159581859, -3.672407670025477522, -19.02952475234523888 ) ) ;
#26855=CARTESIAN_POINT ( 'NONE',  ( 6.925036540929339957, 35.55535081222223681, -8.883103387068663537 ) ) ;
#26859=CARTESIAN_POINT ( 'NONE',  ( 15.74947785296019021, -20.78724321937316333, -18.03682299684260570 ) ) ;
#26863=ORIENTED_EDGE ( 'NONE', *, *, #4895, .T. ) ;
#26864=CARTESIAN_POINT ( 'NONE',  ( 13.14824004184070638, 22.34849671386530190, -16.42994992985817149 ) ) ;
#26866=EDGE_LOOP ( 'NONE', ( #28876, #14903, #12895, #35325 ) ) ;
#26867=CARTESIAN_POINT ( 'NONE',  ( -15.29345365570516435, 25.52021322302956818, -8.773791920665329869 ) ) ;
#26871=CARTESIAN_POINT ( 'NONE',  ( 12.21409306628939184, 19.82566689378781888, -20.55567861157228648 ) ) ;
#26873=CARTESIAN_POINT ( 'NONE',  ( 27.95286989306738690, -16.54226243461976154, -13.80388540367800054 ) ) ;
#26875=CARTESIAN_POINT ( 'NONE',  ( -13.26571186845993289, 23.26405244385044924, -15.39968056061676549 ) ) ;
#26877=CARTESIAN_POINT ( 'NONE',  ( -10.23258877305064196, -17.82419513942780753, -28.67841817144874739 ) ) ;
#26879=CIRCLE ( 'NONE', #32720, 16.00000000000000000 ) ;
#26881=CARTESIAN_POINT ( 'NONE',  ( -34.55718164801944425, -11.87514214786398448, -8.441259157958310055 ) ) ;
#26882=CARTESIAN_POINT ( 'NONE',  ( -9.018257521923398912, -18.41052938026230024, -30.00000000000000000 ) ) ;
#26885=CARTESIAN_POINT ( 'NONE',  ( 28.97648499451679527, 1.995013090243813236, -5.474227664210660649 ) ) ;
#26889=CARTESIAN_POINT ( 'NONE',  ( -29.87381286097529198, -0.03451733885659702405, -9.704015530497390074 ) ) ;
#26890=CARTESIAN_POINT ( 'NONE',  ( 20.50011096633554786, 0.05624224123783942708, -29.33361002156190978 ) ) ;
#26895=CARTESIAN_POINT ( 'NONE',  ( -26.41979680957344812, 2.663940752761243758, -12.66501335940618311 ) ) ;
#26905=DIRECTION ( 'NONE',  ( 0.000000000000000000, 0.000000000000000000, 1.000000000000000000 ) ) ;
#26908=CARTESIAN_POINT ( 'NONE',  ( -24.91587395908689828, 6.157934535019561118, -9.832588768546241198 ) ) ;
#26911=CARTESIAN_POINT ( 'NONE',  ( 14.80116457086245063, -14.50031048367034003, -27.79137631540835329 ) ) ;
#26914=CARTESIAN_POINT ( 'NONE',  ( 15.22398294079505732, 27.00394357737293660, -6.879655644394929936 ) ) ;
#26917=CARTESIAN_POINT ( 'NONE',  ( -13.95161305026674015, 16.60687172368021081, -23.05558987895942380 ) ) ;
#26923=CARTESIAN_POINT ( 'NONE',  ( 11.13905890951745548, 17.60318892418004566, -26.83172267188130533 ) ) ;
#26925=CARTESIAN_POINT ( 'NONE',  ( 10.98647152928299597, 17.30743895948370081, -29.34839841643595904 ) ) ;
#26927=CARTESIAN_POINT ( 'NONE',  ( -11.12155928551759132, 17.80160828069594459, -26.21807330386510060 ) ) ;
#26929=CARTESIAN_POINT ( 'NONE',  ( -13.79154419894701711, -24.12836806479996099, -13.50637930408640486 ) ) ;
#26932=CARTESIAN_POINT ( 'NONE',  ( -24.36260255128434693, -13.71872778104093626, -17.59360786939599919 ) ) ;
#26933=CARTESIAN_POINT ( 'NONE',  ( -7.584868861406902418, -22.23149659495907216, -17.80198783937951035 ) ) ;
#26935=CARTESIAN_POINT ( 'NONE',  ( 15.39490642557507805, 24.42544543857336237, -9.730889705983216231 ) ) ;
#26937=CARTESIAN_POINT ( 'NONE',  ( 24.00150849657053342, 7.288234594027279023, -10.34479505154993006 ) ) ;
#26939=FACE_OUTER_BOUND ( 'NONE', #27593, .T. ) ;
#26943=CARTESIAN_POINT ( 'NONE',  ( -20.50243331965346627, -0.1390943044478715751, -30.00000000000000000 ) ) ;
#26944=CARTESIAN_POINT ( 'NONE',  ( 26.54774961419984791, 0.2119857837146491009, -15.44276492342872942 ) ) ;
#26957=CARTESIAN_POINT ( 'NONE',  ( 0.3974060216068843188, 36.87773723323857666, -9.281964161181997852 ) ) ;
#26963=FACE_OUTER_BOUND ( 'NONE', #23545, .T. ) ;
#26965=CARTESIAN_POINT ( 'NONE',  ( 10.88564509527626711, 20.38589894840641037, -21.43542534558934420 ) ) ;
#26969=CARTESIAN_POINT ( 'NONE',  ( -19.27426644434435943, 15.23580267750421768, -10.36995949012763951 ) ) ;
#26973=CARTESIAN_POINT ( 'NONE',  ( 12.67787564303985093, -22.55830435898898045, -16.44121654803666033 ) ) ;
#26975=DIRECTION ( 'NONE',  ( 1.000000000000000000, 0.000000000000000000, 0.000000000000000000 ) ) ;
#26976=CARTESIAN_POINT ( 'NONE',  ( 13.19712304331239849, 22.25851351613993501, -16.44121704333481659 ) ) ;
#26979=CARTESIAN_POINT ( 'NONE',  ( -15.84100732309063453, -13.15637747550469605, -28.47180823155512286 ) ) ;
#26980=CARTESIAN_POINT ( 'NONE',  ( 1.757052035680020996, -24.31965863861416466, -9.891202175810470010 ) ) ;
#26981=CARTESIAN_POINT ( 'NONE',  ( 15.47372898463780899, 26.31603480030968711, -6.417418525855842937 ) ) ;
#26982=CARTESIAN_POINT ( 'NONE',  ( 20.56691591868512603, 12.65939849767090131, -10.88559607822821640 ) ) ;
#26985=CARTESIAN_POINT ( 'NONE',  ( -5.057544419104798905, 24.90275516936592126, -19.74804168192481058 ) ) ;
#26994=CARTESIAN_POINT ( 'NONE',  ( -20.80125368753044057, 0.9936892722615382478, -26.84302245589054081 ) ) ;
#26996=CARTESIAN_POINT ( 'NONE',  ( 35.47190708691255168, -11.90251233358380212, -5.439855546327714286 ) ) ;
#27009=DIRECTION ( 'NONE',  ( -1.000000000000000000, 0.000000000000000000, 0.000000000000000000 ) ) ;
#27012=CARTESIAN_POINT ( 'NONE',  ( 19.19831057544300634, 15.58298917004336381, -9.871960784555227519 ) ) ;
#27013=CARTESIAN_POINT ( 'NONE',  ( 9.500247868936627427, 26.82341383387064582, -15.94768270033280366 ) ) ;
#27015=CARTESIAN_POINT ( 'NONE',  ( -18.81973674586063439, 9.357238322791348040, -24.40929192524837887 ) ) ;
#27018=CARTESIAN_POINT ( 'NONE',  ( 9.846686707545563522, -18.36693667979134048, -26.81703511278297469 ) ) ;
#27024=CARTESIAN_POINT ( 'NONE',  ( -12.12621152392383372, 19.92962288602521781, -20.53998900965990160 ) ) ;
#27026=CARTESIAN_POINT ( 'NONE',  ( 9.072119448907619343, -18.72396509061168501, -26.88084378092850102 ) ) ;
#27031=CARTESIAN_POINT ( 'NONE',  ( -7.145981593079294925, 19.42380627178312480, -27.86802767370806677 ) ) ;
#27036=CARTESIAN_POINT ( 'NONE',  ( 25.16949050179799841, 0.4568851818789111952, -17.44635195342746314 ) ) ;
#27041=CARTESIAN_POINT ( 'NONE',  ( -20.48147506303724441, 0.8713082578521279542, -30.00000000000000000 ) ) ;
#27045=CARTESIAN_POINT ( 'NONE',  ( 20.60546234692413847, -2.909310255760186870, -27.21192818574509786 ) ) ;
#27051=CARTESIAN_POINT ( 'NONE',  ( -35.84808252048276955, -3.038699442442200027, -5.000000000000005329 ) ) ;
#27060=CARTESIAN_POINT ( 'NONE',  ( 7.011078276407629595, 36.06490844421831099, -8.006587430816212603 ) ) ;
#27063=CARTESIAN_POINT ( 'NONE',  ( 18.66842418841368101, -27.23445290579710232, -5.917650609604824474 ) ) ;
#27068=CARTESIAN_POINT ( 'NONE',  ( 12.07661549505689536, 19.98892357814243681, -20.52991758538416889 ) ) ;
#27070=CARTESIAN_POINT ( 'NONE',  ( -11.90844352419377827, 18.06674963033532322, -23.91691853855833116 ) ) ;
#27073=CARTESIAN_POINT ( 'NONE',  ( 11.25263760713990280, 17.70681266469984294, -26.23215722482760981 ) ) ;
#27075=CARTESIAN_POINT ( 'NONE',  ( 17.72709310700289720, -10.48608855509684901, -28.44358586278453060 ) ) ;
#27077=CARTESIAN_POINT ( 'NONE',  ( -10.64042804724655689, 17.68140777639901984, -28.05361844119051540 ) ) ;
#27079=CARTESIAN_POINT ( 'NONE',  ( -17.30319042518958383, -25.82435514465430515, -10.50227512508310923 ) ) ;
#27084=CARTESIAN_POINT ( 'NONE',  ( -20.53428788010907979, -7.794484820519511636, -24.29087954726551857 ) ) ;
#27085=CARTESIAN_POINT ( 'NONE',  ( -9.394160329388485664, -18.36112709139673171, -28.08710526393325324 ) ) ;
#27088=CARTESIAN_POINT ( 'NONE',  ( 22.69882725526681710, 2.255467933073600051, -20.73643980054142943 ) ) ;
#27093=CARTESIAN_POINT ( 'NONE',  ( -25.91514792629616437, 0.2343253458700045866, -16.43276076001953356 ) ) ;
#27095=CARTESIAN_POINT ( 'NONE',  ( 25.57042713151565749, -0.2977480437168726346, -17.35121141349176455 ) ) ;
#27098=CARTESIAN_POINT ( 'NONE',  ( -23.46629586039856363, 2.745952860400708406, -18.68457461683295762 ) ) ;
#27107=ORIENTED_EDGE ( 'NONE', *, *, #851, .F. ) ;
#27108=CARTESIAN_POINT ( 'NONE',  ( -20.36783817944476027, 5.016842631823707599, -25.36215431227993022 ) ) ;
#27111=CARTESIAN_POINT ( 'NONE',  ( 16.13373544545436999, -15.79625797353112482, -23.17830139746911655 ) ) ;
#27115=CARTESIAN_POINT ( 'NONE',  ( 12.11058524023762040, 20.85765977519871939, -19.43838798737532514 ) ) ;
#27119=CARTESIAN_POINT ( 'NONE',  ( -16.58187255403813509, 22.94673014519461773, -5.949379142203228277 ) ) ;
#27123=CARTESIAN_POINT ( 'NONE',  ( 11.70346012238788980, 18.89484313388442160, -22.73802100965551176 ) ) ;
#27127=CARTESIAN_POINT ( 'NONE',  ( -15.30745419785728778, 26.89740918011089121, -6.413591019650938918 ) ) ;
#27129=CARTESIAN_POINT ( 'NONE',  ( -10.89308438657891465, -19.97759514595176356, -21.60980701075553867 ) ) ;
#27131=CARTESIAN_POINT ( 'NONE',  ( -20.35163850574221556, -12.28510868635483000, -21.83632322477828680 ) ) ;
#27132=CARTESIAN_POINT ( 'NONE',  ( -7.667318022502500163, -19.44231725057151294, -26.40555248174693048 ) ) ;
#27134=CARTESIAN_POINT ( 'NONE',  ( 11.91108122330540375, 16.91021841892633049, -27.50939510565961044 ) ) ;
#27137=CARTESIAN_POINT ( 'NONE',  ( 23.59500296165097666, 6.292542308228194159, -13.80885738943037389 ) ) ;
#27143=CARTESIAN_POINT ( 'NONE',  ( -30.31125568725408570, -1.084487226365530743, -10.56604182229928135 ) ) ;
#27145=CARTESIAN_POINT ( 'NONE',  ( 26.60678562830161553, 0.1240764605644925633, -15.43182042406326815 ) ) ;
#27149=CARTESIAN_POINT ( 'NONE',  ( 23.06249103411542478, 13.31513540672987972, -4.999999999999992006 ) ) ;
#27152=EDGE_CURVE ( 'NONE', #1450, #32508, #1273, .T. ) ;
#27158=CARTESIAN_POINT ( 'NONE',  ( 0.2195541181463148694, 20.74688730825959837, -27.70547263837515217 ) ) ;
#27166=CARTESIAN_POINT ( 'NONE',  ( 13.53295666386236995, 26.20769765665461648, -12.41112605713692396 ) ) ;
#27170=CARTESIAN_POINT ( 'NONE',  ( -16.62029253314668864, 12.60395031145305289, -25.48503712365854312 ) ) ;
#27173=CARTESIAN_POINT ( 'NONE',  ( 12.29527272661349713, -22.02268596340331186, -17.43674506788135048 ) ) ;
#27175=CARTESIAN_POINT ( 'NONE',  ( 13.75279816399555877, 23.43377685412391287, -14.47231226931382864 ) ) ;
#27181=CARTESIAN_POINT ( 'NONE',  ( -17.92780664361741927, -14.00736870931739375, -23.04536792413068724 ) ) ;
#27182=CARTESIAN_POINT ( 'NONE',  ( 4.025418116673052715, -24.86707171575129038, -5.481476286668475417 ) ) ;
#27183=CARTESIAN_POINT ( 'NONE',  ( 15.58410715161808824, 26.18909738223269557, -5.474078854422544715 ) ) ;
#27184=CARTESIAN_POINT ( 'NONE',  ( 18.48238482655413861, 11.30487917964827105, -21.18117017502385480 ) ) ;
#27186=CARTESIAN_POINT ( 'NONE',  ( -4.180913945065587889, 37.58733905612867687, -7.125526861301994863 ) ) ;
#27192=CARTESIAN_POINT ( 'NONE',  ( -20.60009190789856959, 1.015461553205563083, -28.08564569100201780 ) ) ;
#27193=CARTESIAN_POINT ( 'NONE',  ( 19.80298806677364709, -5.334938486795024026, -29.99999999999998579 ) ) ;
#27209=CARTESIAN_POINT ( 'NONE',  ( 29.55170335801485493, -22.74801049114014972, -7.986860386523519928 ) ) ;
#27210=CARTESIAN_POINT ( 'NONE',  ( 17.32108554687955149, 13.66007284228603602, -20.07984646109152038 ) ) ;
#27211=CARTESIAN_POINT ( 'NONE',  ( 9.198933924422197705, 23.73018153482928128, -19.01023341765094798 ) ) ;
#27213=CARTESIAN_POINT ( 'NONE',  ( -19.43993472154038216, 9.610213393078213429, -21.17343657839546722 ) ) ;
#27216=CARTESIAN_POINT ( 'NONE',  ( 15.22921972075588748, -26.04634760375180491, -9.226272813048730370 ) ) ;
#27219=CARTESIAN_POINT ( 'NONE',  ( 17.34253826539385201, 27.32041144647958575, -13.70816084473008800 ) ) ;
#27221=CARTESIAN_POINT ( 'NONE',  ( -15.35818044939771632, 26.72156206222938124, -6.416418653425738583 ) ) ;
#27223=CARTESIAN_POINT ( 'NONE',  ( -20.50183232903691177, -24.38735400865616754, -12.17096377724693035 ) ) ;
#27224=CARTESIAN_POINT ( 'NONE',  ( 14.14567267149670293, -26.22303375651868151, -7.362319143684429079 ) ) ;
#27229=CARTESIAN_POINT ( 'NONE',  ( -10.84359833522533023, 29.92721541907581084, -12.17318395035172074 ) ) ;
#27234=CARTESIAN_POINT ( 'NONE',  ( 20.60758928576245452, 0.8974886860145109280, -28.07985037303415510 ) ) ;
#27238=CARTESIAN_POINT ( 'NONE',  ( -28.88209946128927896, 0.1111908453527043067, -11.59938499466097817 ) ) ;
#27241=CARTESIAN_POINT ( 'NONE',  ( 22.75668780360189203, -3.280807789042111899, -22.27935141650941375 ) ) ;
#27256=CARTESIAN_POINT ( 'NONE',  ( 7.928258658476393883, 35.05882616698742282, -8.896045816660139494 ) ) ;
#27259=CARTESIAN_POINT ( 'NONE',  ( 19.27831178257280698, -25.27455051888069804, -11.31654119470542064 ) ) ;
#27266=CARTESIAN_POINT ( 'NONE',  ( 11.63972795867577936, 18.95610267478247479, -22.72707233481362721 ) ) ;
#27268=CARTESIAN_POINT ( 'NONE',  ( -15.59869368156687486, 26.13660472685725722, -5.474064220111173995 ) ) ;
#27271=CARTESIAN_POINT ( 'NONE',  ( 14.80295835475978627, -25.81819152709282505, -9.710063844406016997 ) ) ;
#27274=CARTESIAN_POINT ( 'NONE',  ( 11.16022610508474067, 17.44351855606713642, -27.45452920518326678 ) ) ;
#27276=CARTESIAN_POINT ( 'NONE',  ( 30.53904149796068879, -19.36372090394836931, -10.17381678346307972 ) ) ;
#27278=CARTESIAN_POINT ( 'NONE',  ( -10.92505544481902469, 18.33161101182201236, -24.96188984657137055 ) ) ;
#27280=CARTESIAN_POINT ( 'NONE',  ( -15.65190729232149280, -24.80065730001655666, -12.43069847511498338 ) ) ;
#27284=CARTESIAN_POINT ( 'NONE',  ( -34.95683723113188535, -12.02710497262000366, -7.574730441631502664 ) ) ;
#27285=CARTESIAN_POINT ( 'NONE',  ( -9.435257979599080969, -18.55952215190476551, -26.85164704141170589 ) ) ;
#27288=CARTESIAN_POINT ( 'NONE',  ( 29.53226466533872596, 1.120089121006105692, -7.363481725902196295 ) ) ;
#27293=CARTESIAN_POINT ( 'NONE',  ( -30.91306671499135916, -0.08701806214385847393, -5.945400134279025472 ) ) ;
#27295=CARTESIAN_POINT ( 'NONE',  ( 31.33932419087585330, -1.338176013559867261, -8.697177606183496223 ) ) ;
#27298=CARTESIAN_POINT ( 'NONE',  ( -25.48877880442670474, 2.684454445128169997, -14.63412680931335430 ) ) ;
#27308=CARTESIAN_POINT ( 'NONE',  ( -25.27117276387230760, 5.256176016299023424, -10.79590797945013492 ) ) ;
#27310=CARTESIAN_POINT ( 'NONE',  ( 0.000000000000000000, 22.50000000000000355, 0.000000000000000000 ) ) ;
#27311=CARTESIAN_POINT ( 'NONE',  ( 15.13892795146889192, -13.95385527665263403, -28.49116766414493185 ) ) ;
#27313=CARTESIAN_POINT ( 'NONE',  ( 10.83909553179808860, 18.00096194490589951, -26.18758634457435264 ) ) ;
#27316=CARTESIAN_POINT ( 'NONE',  ( -13.42818987338513459, 17.16911081534734862, -22.99155224325752300 ) ) ;
#27320=CARTESIAN_POINT ( 'NONE',  ( 15.43121851897235786, 26.72868093004962020, -4.999999999999998224 ) ) ;
#27324=CARTESIAN_POINT ( 'NONE',  ( -13.95668707828244059, 24.11263528183340554, -13.49652051132212094 ) ) ;
#27325=CARTESIAN_POINT ( 'NONE',  ( -37.48557158514997667, -11.24999999999982414, 3.000000000000000000 ) ) ;
#27326=CARTESIAN_POINT ( 'NONE',  ( -14.07101309938052403, -24.61591519948004603, -12.54868197112087103 ) ) ;
#27329=CARTESIAN_POINT ( 'NONE',  ( -29.19019149203798591, -16.43308044909656829, -12.88835385468937744 ) ) ;
#27330=CARTESIAN_POINT ( 'NONE',  ( -9.622411929345382475, -22.55102273573495353, -16.66494747511510610 ) ) ;
#27331=FACE_OUTER_BOUND ( 'NONE', #19677, .T. ) ;
#27332=CARTESIAN_POINT ( 'NONE',  ( 15.09791029636327764, 22.51266978359509707, -12.62702112920867847 ) ) ;
#27334=CARTESIAN_POINT ( 'NONE',  ( 24.22245084703565610, 6.361410862367799623, -11.80793526373495261 ) ) ;
#27340=CARTESIAN_POINT ( 'NONE',  ( -24.47322330375783039, -0.9128233859311521980, -19.31502028455822639 ) ) ;
#27341=CARTESIAN_POINT ( 'NONE',  ( 27.86069736982781464, 0.03076757672864667559, -13.49648488625461340 ) ) ;
#27344=CARTESIAN_POINT ( 'NONE',  ( 21.88499642459564143, -5.528038495964486820, -20.11584339644707597 ) ) ;
#27351=CARTESIAN_POINT ( 'NONE',  ( 33.62187204924162387, 0.04418559750794539415, -5.000000000000002665 ) ) ;
#27352=CARTESIAN_POINT ( 'NONE',  ( 3.669446457248423332, 35.72068143852440869, -10.18510980848603253 ) ) ;
#27353=AXIS2_PLACEMENT_3D ( 'NONE', #17275, #4665, #38588 ) ;
#27359=DIRECTION ( 'NONE',  ( -0.000000000000000000, -0.000000000000000000, 1.000000000000000000 ) ) ;
#27361=CARTESIAN_POINT ( 'NONE',  ( 14.82527878907322538, 28.13924469978218923, -6.856551512622178990 ) ) ;
#27363=ORIENTED_EDGE ( 'NONE', *, *, #4272, .T. ) ;
#27364=CARTESIAN_POINT ( 'NONE',  ( -16.15483981359775001, 13.22461535667768473, -25.46561888468577806 ) ) ;
#27367=CARTESIAN_POINT ( 'NONE',  ( 15.42709217669442090, -26.65236356593726796, -6.416988218343957939 ) ) ;
#27368=CARTESIAN_POINT ( 'NONE',  ( -21.08265500991413788, -26.45952537750927291, -8.564919882568894138 ) ) ;
#27370=CARTESIAN_POINT ( 'NONE',  ( 15.40434907611582638, 26.82505288294843027, -4.999999999999998224 ) ) ;
#27374=CARTESIAN_POINT ( 'NONE',  ( -16.86820373146711205, -13.17562041779036441, -25.62346928861798290 ) ) ;
#27375=CARTESIAN_POINT ( 'NONE',  ( -0.3862909676465622333, -24.66147537587169225, -7.427960836158034930 ) ) ;
#27376=CARTESIAN_POINT ( 'NONE',  ( 15.50752910295250864, 26.03341394949190857, -6.889194152022838580 ) ) ;
#27377=CARTESIAN_POINT ( 'NONE',  ( 21.38745727808766617, 11.90858952770566503, -8.901519087829083077 ) ) ;
#27380=CARTESIAN_POINT ( 'NONE',  ( -3.058361328855125905, 21.76692312865797518, -24.27252685025706924 ) ) ;
#27382=CARTESIAN_POINT ( 'NONE',  ( -30.62108498763855380, -5.687012903234330174, -13.09446411654519160 ) ) ;
#27388=CARTESIAN_POINT ( 'NONE',  ( -30.06895585930082149, 0.4279890562384842112, -7.831005020092066893 ) ) ;
#27389=CARTESIAN_POINT ( 'NONE',  ( 21.31962645927955435, -7.874799234479001875, -23.07151141173847364 ) ) ;
#27391=ORIENTED_EDGE ( 'NONE', *, *, #15617, .F. ) ;
#27395=CARTESIAN_POINT ( 'NONE',  ( -19.48557158514985588, -11.25000000000002309, 6.000000000000000000 ) ) ;
#27397=PRODUCT_DEFINITION ( 'UNKNOWN', '', #15190, #33399 ) ;
#27404=ADVANCED_FACE ( 'NONE', ( #34103 ), #27802, .T. ) ;
#27406=CARTESIAN_POINT ( 'NONE',  ( 30.06306975117524871, -23.11802603997359284, -6.283344179835762766 ) ) ;
#27407=CARTESIAN_POINT ( 'NONE',  ( 17.66171978117526109, 15.32956390713761685, -15.88260630329942025 ) ) ;
#27408=CARTESIAN_POINT ( 'NONE',  ( 8.281587164622539632, 23.34602691232715088, -19.97899749236660938 ) ) ;
#27410=CARTESIAN_POINT ( 'NONE',  ( -19.92126674643909823, 9.807663499646920968, -19.05809710863068318 ) ) ;
#27414=CARTESIAN_POINT ( 'NONE',  ( 9.734775949363912773, -18.28479368612017808, -27.43959765210956547 ) ) ;
#27416=CARTESIAN_POINT ( 'NONE',  ( 22.52744239175980923, -0.1803094636422790109, -20.90349153981001606 ) ) ;
#27417=CARTESIAN_POINT ( 'NONE',  ( -13.46909128543195777, 22.86125717629003873, -15.44550393738605187 ) ) ;
#27418=CARTESIAN_POINT ( 'NONE',  ( -20.30842559917252288, -22.79334907695596613, -14.00205457863687997 ) ) ;
#27419=CARTESIAN_POINT ( 'NONE',  ( 9.644836438174420934, -23.72159211153909908, -13.69389272877596575 ) ) ;
#27426=CARTESIAN_POINT ( 'NONE',  ( -10.14280199068175214, 30.64235453448604218, -12.13460695665965972 ) ) ;
#27432=CARTESIAN_POINT ( 'NONE',  ( 26.50276232455322400, 0.2790718576921050187, -15.45068151253284761 ) ) ;
#27435=VERTEX_POINT ( 'NONE', #24747 ) ;
#27436=CARTESIAN_POINT ( 'NONE',  ( -30.32473157615882542, 0.02510865282379010077, -8.297974377023098924 ) ) ;
#27439=CARTESIAN_POINT ( 'NONE',  ( 32.94587109690223059, -4.956964677168978817, -9.466786290515122104 ) ) ;
#27449=CARTESIAN_POINT ( 'NONE',  ( 19.48557158514988075, -11.24999999999998224, 3.000000000000000000 ) ) ;
#27452=CARTESIAN_POINT ( 'NONE',  ( 3.517372515104220998, 21.68025459727664384, -24.29102002352656697 ) ) ;
#27456=CARTESIAN_POINT ( 'NONE',  ( 16.88935835353887427, -24.86429512234964534, -12.34860920598776168 ) ) ;
#27463=CARTESIAN_POINT ( 'NONE',  ( -14.75406920065014482, 25.34787871228437695, -10.65428902387546728 ) ) ;
#27464=CIRCLE ( 'NONE', #28095, 60.00000000000002132 ) ;
#27466=CARTESIAN_POINT ( 'NONE',  ( 10.46763271599406053, -19.59569900990302571, -22.74339197413747371 ) ) ;
#27470=CARTESIAN_POINT ( 'NONE',  ( -13.23108492885968523, 26.81331637706469806, -12.36580983879895612 ) ) ;
#27472=CARTESIAN_POINT ( 'NONE',  ( -14.75978416138969962, -21.06827879612096055, -18.13044228312590178 ) ) ;
#27477=CARTESIAN_POINT ( 'NONE',  ( -31.75624639457006637, -11.96584483983997771, -12.01004037356029031 ) ) ;
#27478=CARTESIAN_POINT ( 'NONE',  ( -14.17779411611103946, -25.03930879169686108, -11.60410842717421609 ) ) ;
#27481=CARTESIAN_POINT ( 'NONE',  ( 21.96305308675481172, 3.028777170395801299, -21.88341145178896596 ) ) ;
#27486=CARTESIAN_POINT ( 'NONE',  ( -23.34921024300090053, 0.4641876397533150622, -20.52991899298079659 ) ) ;
#27488=CARTESIAN_POINT ( 'NONE',  ( 20.86070950977947547, 0.1829700343765511272, -26.78014837192183251 ) ) ;
#27492=CARTESIAN_POINT ( 'NONE',  ( -21.64712599719590713, 2.830533044877102000, -22.97171106603809321 ) ) ;
#27505=CARTESIAN_POINT ( 'NONE',  ( -20.58226371439221225, 7.343079615373506286, -21.10892354972650509 ) ) ;
#27508=CARTESIAN_POINT ( 'NONE',  ( 25.01399590262306205, -25.94755112289962895, -7.176433082738011393 ) ) ;
#27510=CARTESIAN_POINT ( 'NONE',  ( 11.10459398110999629, 18.19651370294324977, -24.98634877528791876 ) ) ;
#27514=CARTESIAN_POINT ( 'NONE',  ( -14.01353083633360441, 19.92937566205294786, -17.60551373979553347 ) ) ;
#27517=CARTESIAN_POINT ( 'NONE',  ( 12.67211246595664598, 21.02606612804661879, -18.45550099276037415 ) ) ;
#27522=CARTESIAN_POINT ( 'NONE',  ( -13.69293301799758034, 23.56752051744286192, -14.45830943805128932 ) ) ;
#27525=CARTESIAN_POINT ( 'NONE',  ( -9.658050167131792207, -18.22926657306539866, -28.07251639296444168 ) ) ;
#27528=CARTESIAN_POINT ( 'NONE',  ( -34.06221145678576079, -17.84677894165469070, -4.999999999999999112 ) ) ;
#27530=CARTESIAN_POINT ( 'NONE',  ( -10.58748765286974702, -24.15557699858428009, -12.67670956590171016 ) ) ;
#27532=CARTESIAN_POINT ( 'NONE',  ( 16.13774221630713157, 23.57012646024468339, -7.846364408462076057 ) ) ;
#27534=CARTESIAN_POINT ( 'NONE',  ( 24.60615563309142573, 7.381059274176844376, -6.443417821428254477 ) ) ;
#27539=CARTESIAN_POINT ( 'NONE',  ( -21.05108527408817665, -0.1996147791734167454, -26.13566238484483506 ) ) ;
#27541=CARTESIAN_POINT ( 'NONE',  ( 30.05477332892332498, -0.03847789688773560479, -9.234382374539894300 ) ) ;
#27544=CARTESIAN_POINT ( 'NONE',  ( 16.24796006241085422, 15.88921519459651144, -30.00000000000001421 ) ) ;
#27549=ORIENTED_EDGE ( 'NONE', *, *, #9525, .T. ) ;
#27553=CARTESIAN_POINT ( 'NONE',  ( 2.739358956307748727, 38.25484015033369189, -5.856888471774574612 ) ) ;
#27561=CARTESIAN_POINT ( 'NONE',  ( 10.27379371539876907, 17.74076016529687649, -29.33306961566889015 ) ) ;
#27564=CARTESIAN_POINT ( 'NONE',  ( -18.73768915581330674, 17.66930787322032259, -5.479690743329737046 ) ) ;
#27567=CARTESIAN_POINT ( 'NONE',  ( 14.05380968864566071, -24.61301880703936362, -12.55008158153441578 ) ) ;
#27568=CARTESIAN_POINT ( 'NONE',  ( -16.28627583843819693, -20.60454327135679975, -17.98998692793695398 ) ) ;
#27569=CARTESIAN_POINT ( 'NONE',  ( 15.23218277980887159, 26.40650644525699775, -7.827771362956433165 ) ) ;
#27570=CARTESIAN_POINT ( 'NONE',  ( 10.96431188987212479, 17.32148673788787718, -30.00000000000000355 ) ) ;
#27577=CARTESIAN_POINT ( 'NONE',  ( -28.40992215798796039, -23.67713899482849627, -7.998235878429071910 ) ) ;
#27578=CARTESIAN_POINT ( 'NONE',  ( -0.3593151151631351348, -23.72602201120211518, -12.88856356360667199 ) ) ;
#27579=CARTESIAN_POINT ( 'NONE',  ( 14.53668546275618567, 23.85743596623326823, -12.57427534489166021 ) ) ;
#27580=CARTESIAN_POINT ( 'NONE',  ( 17.58908954919914436, 10.72208735757384979, -27.73727666948197879 ) ) ;
#27583=CARTESIAN_POINT ( 'NONE',  ( -3.525063703014029048, 20.58869973712754842, -27.01785507751000637 ) ) ;
#27585=CARTESIAN_POINT ( 'NONE',  ( -33.08849987016296978, -5.231495020973413901, -9.455626480001546597 ) ) ;
#27588=DIRECTION ( 'NONE',  ( 1.000000000000000000, 0.000000000000000000, 0.000000000000000000 ) ) ;
#27590=CARTESIAN_POINT ( 'NONE',  ( -30.04950648410215308, 0.8457024189327569941, -5.000000000000000000 ) ) ;
#27591=CARTESIAN_POINT ( 'NONE',  ( 27.95927371423643848, -10.27070572539359716, -15.74113732760950413 ) ) ;
#27593=EDGE_LOOP ( 'NONE', ( #31725, #8931, #6982, #10703 ) ) ;
#27603=CARTESIAN_POINT ( 'NONE',  ( -1.631256786664503577, 20.52137151614312316, -28.45067076138309403 ) ) ;
#27606=CARTESIAN_POINT ( 'NONE',  ( 26.21828973787456007, -21.49016925214971963, -12.01153406443311766 ) ) ;
#27607=CARTESIAN_POINT ( 'NONE',  ( 17.12406237791118357, 13.45638816638915358, -21.13750791658128847 ) ) ;
#27608=CARTESIAN_POINT ( 'NONE',  ( 13.73220224370217579, 30.78478150535875457, -4.999999999999995559 ) ) ;
#27610=CARTESIAN_POINT ( 'NONE',  ( -21.15916498104113685, 10.31847808661841626, -13.90054347323569139 ) ) ;
#27612=CARTESIAN_POINT ( 'NONE',  ( 9.721599711338530625, -18.19680360149917320, -28.06894580268500405 ) ) ;
#27614=CARTESIAN_POINT ( 'NONE',  ( 33.62187204924162387, 0.04418559750795045954, -13.79123840944733992 ) ) ;
#27615=CARTESIAN_POINT ( 'NONE',  ( -15.09127514311057716, 26.17197197711360346, -8.766134727060833853 ) ) ;
#27616=CARTESIAN_POINT ( 'NONE',  ( -14.12043127772994922, -15.90989924622459384, -25.81352569219153281 ) ) ;
#27617=CARTESIAN_POINT ( 'NONE',  ( 8.584620562788320086, -18.61902014996657684, -30.00000000000000000 ) ) ;
#27622=CARTESIAN_POINT ( 'NONE',  ( -10.17671610307063546, 34.24920776341300410, -7.617059711015554235 ) ) ;
#27624=FACE_OUTER_BOUND ( 'NONE', #29967, .T. ) ;
#27630=CARTESIAN_POINT ( 'NONE',  ( 30.60837755444375929, -0.01021490497896947874, -7.357883460921571306 ) ) ;
#27632=CARTESIAN_POINT ( 'NONE',  ( -15.41558956984166251, 26.78481017248024898, -5.000000000000000000 ) ) ;
#27637=CARTESIAN_POINT ( 'NONE',  ( -30.14882232463217804, 0.05009394220924950902, -8.768162902875424436 ) ) ;
#27640=CARTESIAN_POINT ( 'NONE',  ( 33.62754581830257194, -6.995946598033712327, -9.406918306848506717 ) ) ;
#27644=CARTESIAN_POINT ( 'NONE',  ( -22.57322471865059299, -29.08065073755651042, -4.999999999999997335 ) ) ;
#27652=EDGE_CURVE ( 'NONE', #10849, #6755, #25283, .T. ) ;
#27654=CARTESIAN_POINT ( 'NONE',  ( 7.126104678631604905, 36.82515065381944197, -5.439468800721699360 ) ) ;
#27658=CARTESIAN_POINT ( 'NONE',  ( 17.23496854698099057, -26.67902877899678060, -8.224554605899342619 ) ) ;
#27663=CARTESIAN_POINT ( 'NONE',  ( -12.28379231215668810, 19.74341564248685899, -20.56797969728914310 ) ) ;
#27665=CARTESIAN_POINT ( 'NONE',  ( 14.08933265271751978, -25.02402006024204084, -11.60661225095639715 ) ) ;
#27669=CARTESIAN_POINT ( 'NONE',  ( -14.28732406086307449, 29.23536459232070328, -7.289172933315514413 ) ) ;
#27670=CARTESIAN_POINT ( 'NONE',  ( -19.47283267323017597, -27.28889818631711250, -5.458695607782805048 ) ) ;
#27674=CARTESIAN_POINT ( 'NONE',  ( -35.47307300072858283, -9.938437602308624719, -5.000000000000004441 ) ) ;
#27675=CARTESIAN_POINT ( 'NONE',  ( -13.21629450091423053, -23.60900218953552354, -14.48483131059268558 ) ) ;
#27678=CARTESIAN_POINT ( 'NONE',  ( 25.25749706778072579, 1.346561751027687936, -16.53357011407651456 ) ) ;
#27682=CARTESIAN_POINT ( 'NONE',  ( -26.56841411643160455, 0.1811368447264279369, -15.43893401616002947 ) ) ;
#27684=CARTESIAN_POINT ( 'NONE',  ( 20.64823133129570110, -0.2909966358367886974, -28.02009057262635139 ) ) ;
#27689=CARTESIAN_POINT ( 'NONE',  ( -20.52618863457681542, 3.592373843541286416, -26.42718072739731028 ) ) ;
#27698=CARTESIAN_POINT ( 'NONE',  ( -24.12023144843434252, 8.019543126731839777, -6.929311169682339511 ) ) ;
#27701=CARTESIAN_POINT ( 'NONE',  ( 13.79453690055875370, -15.27553076837868495, -28.53576636504390152 ) ) ;
#27702=DIRECTION ( 'NONE',  ( -0.000000000000000000, -0.000000000000000000, -1.000000000000000000 ) ) ;
#27703=CARTESIAN_POINT ( 'NONE',  ( 15.21680204932512304, 26.78069555836370697, -7.350879659809681499 ) ) ;
#27706=CARTESIAN_POINT ( 'NONE',  ( -12.84546241753605855, 16.03363458260228924, -28.77567867939699653 ) ) ;
#27710=CARTESIAN_POINT ( 'NONE',  ( 11.05637708650255036, 17.41422535994987086, -28.07838520724235565 ) ) ;
#27712=CARTESIAN_POINT ( 'NONE',  ( -2.485571585149885632, -11.24999999999987566, 10.00000000000000000 ) ) ;
#27715=CARTESIAN_POINT ( 'NONE',  ( -12.00916977197048752, 20.06877922548516935, -20.51635596422970664 ) ) ;
#27718=CARTESIAN_POINT ( 'NONE',  ( -10.93634242917226373, -19.96742847112642849, -21.60398965136151972 ) ) ;
#27722=CARTESIAN_POINT ( 'NONE',  ( -21.14746589409385535, -12.76649274373130183, -20.68958427074545980 ) ) ;
#27723=CARTESIAN_POINT ( 'NONE',  ( -11.22534350456744612, -25.23047905509118394, -9.287595664362980230 ) ) ;
#27725=CARTESIAN_POINT ( 'NONE',  ( 11.87983786580489820, 16.84351847752386178, -28.12481558007895899 ) ) ;
#27728=CARTESIAN_POINT ( 'NONE',  ( 19.82805615916967312, 5.207665154685882314, -29.40699823107372524 ) ) ;
#27734=CARTESIAN_POINT ( 'NONE',  ( -31.19464554439533899, -0.7868789741791578640, -7.795315093382260585 ) ) ;
#27735=CARTESIAN_POINT ( 'NONE',  ( 21.28465047978626146, 0.7165814371454377607, -25.00808991143824755 ) ) ;
#27740=CARTESIAN_POINT ( 'NONE',  ( 22.45323650136968396, -2.382502413133517738, -20.55760979252983134 ) ) ;
#27746=CARTESIAN_POINT ( 'NONE',  ( -10.09922753093611192, -27.41777246569288451, -4.999999999999999112 ) ) ;
#27752=CARTESIAN_POINT ( 'NONE',  ( 0.8308715916267807033, 20.49243450554475743, -29.21251993523028290 ) ) ;
#27753=CARTESIAN_POINT ( 'NONE',  ( 16.00000000000000000, 22.50000000000000711, 10.00000000000000000 ) ) ;
#27759=CARTESIAN_POINT ( 'NONE',  ( 10.33186281181274424, 17.87145931443220093, -28.03536056408174915 ) ) ;
#27762=CARTESIAN_POINT ( 'NONE',  ( -16.21686205092897026, 15.87015845977987638, -18.92977423509347190 ) ) ;
#27765=CARTESIAN_POINT ( 'NONE',  ( 9.504747149499191750, -18.16341882422712573, -30.00000000000000000 ) ) ;
#27766=CARTESIAN_POINT ( 'NONE',  ( -15.20277289067466420, -19.27049939871586304, -20.06318638457704395 ) ) ;
#27767=CARTESIAN_POINT ( 'NONE',  ( 13.76661467574959907, 23.40248112065832231, -14.47560752045290755 ) ) ;
#27768=CARTESIAN_POINT ( 'NONE',  ( 13.76109791490951473, 23.41500128713417439, -14.47428817913493582 ) ) ;
#27771=CARTESIAN_POINT ( 'NONE',  ( -15.41457889571365669, -26.69797501666770145, -5.946085984683254999 ) ) ;
#27777=CARTESIAN_POINT ( 'NONE',  ( -28.71250260137452059, -23.91295777942312739, -7.138176182773029232 ) ) ;
#27778=CARTESIAN_POINT ( 'NONE',  ( -2.553198430222350712, -24.56346249274959348, -8.406762110482494776 ) ) ;
#27779=CARTESIAN_POINT ( 'NONE',  ( 15.61108509054414917, 26.00910297926085235, -5.946291585397761814 ) ) ;
#27781=CARTESIAN_POINT ( 'NONE',  ( 20.01029315168119282, 12.29792661527229569, -13.90631728972765124 ) ) ;
#27783=CARTESIAN_POINT ( 'NONE',  ( -4.379796608956421977, 30.71736661111763667, -14.76804172563591777 ) ) ;
#27786=CARTESIAN_POINT ( 'NONE',  ( -34.83329005959444657, -6.589775719143758259, -5.448933541975200967 ) ) ;
#27790=DIRECTION ( 'NONE',  ( 0.000000000000000000, 0.000000000000000000, 1.000000000000000000 ) ) ;
#27792=CARTESIAN_POINT ( 'NONE',  ( -25.00566865627084923, 0.7636625105755581178, -17.47633105975672052 ) ) ;
#27793=CARTESIAN_POINT ( 'NONE',  ( 30.70933288805361983, -12.32817769576170441, -12.91955702887979562 ) ) ;
#27794=ORIENTED_EDGE ( 'NONE', *, *, #39941, .T. ) ;
#27802=CYLINDRICAL_SURFACE ( 'NONE', #18165, 17.00000000000000711 ) ;
#27804=CARTESIAN_POINT ( 'NONE',  ( -1.923949180127531466, 38.42603324025853340, -5.435599845266582797 ) ) ;
#27809=CARTESIAN_POINT ( 'NONE',  ( 27.76036423759017424, -22.74041533840534157, -9.756283338662747440 ) ) ;
#27810=CARTESIAN_POINT ( 'NONE',  ( 16.30176999113392355, 13.74177821074143147, -23.26433688756818086 ) ) ;
#27811=AXIS2_PLACEMENT_3D ( 'NONE', #25134, #27790, #40174 ) ;
#27812=CARTESIAN_POINT ( 'NONE',  ( 12.46298602409325618, 29.89662867798026369, -10.40118216561738151 ) ) ;
#27814=CARTESIAN_POINT ( 'NONE',  ( -20.71763460597477291, 13.68537009249746461, -5.482835118453670553 ) ) ;
#27816=CARTESIAN_POINT ( 'NONE',  ( 13.54728634190223779, -23.64058435204617226, -14.45986489698174182 ) ) ;
#27818=CARTESIAN_POINT ( 'NONE',  ( 35.36940577612500647, -20.42053594592275800, -14.51648065752882566 ) ) ;
#27820=CARTESIAN_POINT ( 'NONE',  ( -12.63876190530728216, 21.07525087859380974, -18.44901738601522467 ) ) ;
#27821=CARTESIAN_POINT ( 'NONE',  ( -19.05194404211813008, -21.38509357595906124, -15.91629285646954273 ) ) ;
#27822=CARTESIAN_POINT ( 'NONE',  ( 10.72379324094551833, -25.60257746891399577, -6.426360612472806544 ) ) ;
#27826=CARTESIAN_POINT ( 'NONE',  ( -6.589341983113207846, 19.77883683989693253, -27.14241267237451538 ) ) ;
#27830=AXIS2_PLACEMENT_3D ( 'NONE', #8474, #20874, #24704 ) ;
#27833=CARTESIAN_POINT ( 'NONE',  ( 20.61009167187485147, 0.8554190281657136907, -28.07775950742859550 ) ) ;
#27835=DIRECTION ( 'NONE',  ( 1.000000000000000000, 0.000000000000000000, 0.000000000000000000 ) ) ;
#27839=CARTESIAN_POINT ( 'NONE',  ( -29.94841971816240545, 0.07655252488241326425, -9.239200560549260643 ) ) ;
#27842=CARTESIAN_POINT ( 'NONE',  ( 34.50778285978141469, -6.214036658931777701, -6.771707614261031516 ) ) ;
#27855=CARTESIAN_POINT ( 'NONE',  ( 8.872206882450816678, 34.45812223078402781, -8.912361989433076559 ) ) ;
#27859=CARTESIAN_POINT ( 'NONE',  ( 11.00000970693004554, -17.98380166451403639, -26.10610249844645026 ) ) ;
#27865=CARTESIAN_POINT ( 'NONE',  ( -11.17092706714288397, 17.24184491651588758, -28.71381065368748509 ) ) ;
#27867=CARTESIAN_POINT ( 'NONE',  ( 9.540210792438220011, -18.51136029728062127, -26.84305259188365156 ) ) ;
#27871=CARTESIAN_POINT ( 'NONE',  ( -9.821329010893958156, 19.10955050348507456, -24.81548820641463848 ) ) ;
#27872=CARTESIAN_POINT ( 'NONE',  ( -15.25086691884292911, -21.72593466508776316, -17.12598327003187393 ) ) ;
#27875=CARTESIAN_POINT ( 'NONE',  ( -25.13972300716358532, -7.830238314601142058, -18.75331848047975569 ) ) ;
#27876=CARTESIAN_POINT ( 'NONE',  ( -10.32636287134091546, -19.63648956442319005, -22.76047509490289400 ) ) ;
#27879=CARTESIAN_POINT ( 'NONE',  ( 27.56524107966918535, 0.4215817824878217990, -13.52655066544985729 ) ) ;
#27884=CARTESIAN_POINT ( 'NONE',  ( -26.53893653578703038, 0.2251345205519453829, -15.44439873174107980 ) ) ;
#27886=CARTESIAN_POINT ( 'NONE',  ( 21.40780153129764685, -0.3772474073816712292, -24.88848197966343889 ) ) ;
#27888=CARTESIAN_POINT ( 'NONE',  ( -7.961096663582920563, -18.90310754077565747, -30.00000000000000355 ) ) ;
#27890=ORIENTED_EDGE ( 'NONE', *, *, #13414, .F. ) ;
#27891=CARTESIAN_POINT ( 'NONE',  ( -23.15794617311298254, 4.315003200217033985, -17.77638817182914721 ) ) ;
#27894=CARTESIAN_POINT ( 'NONE',  ( 0.000000000000000000, 22.50000000000000355, 10.00000000000000000 ) ) ;
#27900=CARTESIAN_POINT ( 'NONE',  ( -19.59498488650715231, 6.415608140812385507, -27.69164703474022815 ) ) ;
#27904=CARTESIAN_POINT ( 'NONE',  ( 13.74558791142738734, -15.22183123319549125, -30.00000000000000355 ) ) ;
#27907=CARTESIAN_POINT ( 'NONE',  ( 13.37007945456113411, 23.06071637790597251, -15.42265832664474878 ) ) ;
#27909=CARTESIAN_POINT ( 'NONE',  ( -15.75218124485975757, 24.12653032028219258, -8.789014821092310470 ) ) ;
#27912=CARTESIAN_POINT ( 'NONE',  ( 11.01299302568612859, 17.29057472414998742, -29.34897105029772746 ) ) ;
#27915=VECTOR ( 'NONE', #10869, 1000.000000000000000 ) ;
#27917=CARTESIAN_POINT ( 'NONE',  ( -14.44494323251225865, 25.21727681637074170, -11.58053765247176514 ) ) ;
#27919=CARTESIAN_POINT ( 'NONE',  ( -15.18541056174788650, -26.03681117208375539, -9.228366842610254750 ) ) ;
#27922=CARTESIAN_POINT ( 'NONE',  ( -18.51744266559586904, -9.015907171310754364, -28.44847492086340424 ) ) ;
#27923=CARTESIAN_POINT ( 'NONE',  ( -8.819735198518117159, -18.71328657623911340, -27.50136144446895514 ) ) ;
#27925=CARTESIAN_POINT ( 'NONE',  ( 16.00132168787127540, 24.22562490985221118, -7.367879038845686068 ) ) ;
#27927=CARTESIAN_POINT ( 'NONE',  ( 26.24647792831409632, 4.660060628212018941, -8.835378462270252697 ) ) ;
#27934=CARTESIAN_POINT ( 'NONE',  ( -29.68641950918352990, -0.3073957355675461245, -10.62315473450874315 ) ) ;
#27935=CARTESIAN_POINT ( 'NONE',  ( 26.05478663030475062, 0.0009985127382727311540, -16.40327240360535299 ) ) ;
#27940=DIRECTION ( 'NONE',  ( -0.000000000000000000, -0.000000000000000000, -1.000000000000000000 ) ) ;
#27948=CARTESIAN_POINT ( 'NONE',  ( 2.699333757401777500, 37.52124286414814236, -7.975407974893957253 ) ) ;
#27951=CARTESIAN_POINT ( 'NONE',  ( -1.485571585149857210, -11.24999999999982236, 3.000000000000000000 ) ) ;
#27955=CARTESIAN_POINT ( 'NONE',  ( 11.81616528917939668, 21.22289557514309877, -19.38120235366460875 ) ) ;
#27959=CARTESIAN_POINT ( 'NONE',  ( -18.50828174693830519, 17.38258355848637393, -8.870643964797142900 ) ) ;
#27963=CARTESIAN_POINT ( 'NONE',  ( 9.522022774849094873, -18.20502493181615122, -28.70691128024250105 ) ) ;
#27964=CARTESIAN_POINT ( 'NONE',  ( -12.53503680232439699, -17.06533640674901164, -25.95590166166768853 ) ) ;
#27966=CARTESIAN_POINT ( 'NONE',  ( 10.97317656914242967, 17.31587133052951089, -30.00000000000000000 ) ) ;
#27969=CARTESIAN_POINT ( 'NONE',  ( -11.81623611950272412, -21.49189391620961942, -18.46105202309505344 ) ) ;
#27971=CARTESIAN_POINT ( 'NONE',  ( -31.45852298323876539, -21.70319895717350533, -6.278571233013221509 ) ) ;
#27972=CARTESIAN_POINT ( 'NONE',  ( -0.3222516639411605599, -22.43452379100889615, -18.01744884572263672 ) ) ;
#27973=CARTESIAN_POINT ( 'NONE',  ( 15.11639032187935072, 25.24504664587892222, -9.717601439789641304 ) ) ;
#27974=CARTESIAN_POINT ( 'NONE',  ( 21.63149483547664076, 10.84510153107085095, -10.88148262729828453 ) ) ;
#27977=CARTESIAN_POINT ( 'NONE',  ( -4.212426069905327530, 37.97930161814787198, -4.999999999999994671 ) ) ;
#27979=CARTESIAN_POINT ( 'NONE',  ( -29.56208081133425836, -4.613024107137377428, -14.07453195671733504 ) ) ;
#27985=CARTESIAN_POINT ( 'NONE',  ( -23.11816775549578651, 1.104452855686005375, -20.60762089766639704 ) ) ;
#27986=CARTESIAN_POINT ( 'NONE',  ( 22.31642213958092924, -7.486323157245182713, -21.96314972916734831 ) ) ;
#27998=EDGE_CURVE ( 'NONE', #31785, #31854, #12507, .T. ) ;
#27999=CARTESIAN_POINT ( 'NONE',  ( -2.493496152838000857, 22.65825999365475951, -23.01938064764903302 ) ) ;
#28005=CARTESIAN_POINT ( 'NONE',  ( 9.081295331449249275, 19.56124383720467108, -24.72641353342787340 ) ) ;
#28008=CARTESIAN_POINT ( 'NONE',  ( -20.94101416334770249, 12.52813585024752463, -9.396077220118929318 ) ) ;
#28010=CARTESIAN_POINT ( 'NONE',  ( 9.808763409072279060, -18.38515136357905888, -26.82030050216148709 ) ) ;
#28012=CARTESIAN_POINT ( 'NONE',  ( 11.06964067281062825, 17.65134693061273907, -26.82519749397791031 ) ) ;
#28013=CARTESIAN_POINT ( 'NONE',  ( -20.55563217186186620, -29.52600041847739831, -13.99876745781540777 ) ) ;
#28015=CARTESIAN_POINT ( 'NONE',  ( -12.91061715790210407, 21.68268698219946344, -17.43355264670666926 ) ) ;
#28017=CARTESIAN_POINT ( 'NONE',  ( -14.77834355681148715, -14.73733460233652437, -27.08378865361848042 ) ) ;
#28018=CARTESIAN_POINT ( 'NONE',  ( 8.691294114719063657, -18.77241989521133902, -27.50980908539149183 ) ) ;
#28019=CARTESIAN_POINT ( 'NONE',  ( 15.14522103274069131, 25.99557503532075842, -8.769033976177988521 ) ) ;
#28020=CARTESIAN_POINT ( 'NONE',  ( 28.45022969918851885, -19.27983063241365969, -11.98101230249146099 ) ) ;
#28023=CARTESIAN_POINT ( 'NONE',  ( -6.508188039552276649, 19.52556562270282470, -28.54081524349888355 ) ) ;
#28025=CARTESIAN_POINT ( 'NONE',  ( 14.23945615837883949, -31.58416516429907972, 0.000000000000000000 ) ) ;
#28030=CARTESIAN_POINT ( 'NONE',  ( 20.48067366615298468, 0.8901913013804809705, -29.34893421961264082 ) ) ;
#28035=CARTESIAN_POINT ( 'NONE',  ( -20.48102978849703604, 0.8817738089609834518, -30.00000000000000000 ) ) ;
#28038=CARTESIAN_POINT ( 'NONE',  ( 34.12941852828814149, -7.118180197318186408, -8.515197907227713969 ) ) ;
#28049=CARTESIAN_POINT ( 'NONE',  ( -14.87461375695690791, 14.12245287598898535, -30.00000000000001776 ) ) ;
#28052=CARTESIAN_POINT ( 'NONE',  ( 4.547395191718751839, 20.23153756940337900, -27.77134476049675627 ) ) ;
#28054=CARTESIAN_POINT ( 'NONE',  ( 11.21391615930829211, -18.27285559791526381, -24.86675532714961534 ) ) ;
#28059=CARTESIAN_POINT ( 'NONE',  ( -15.43019833371434579, 26.73233873233005653, -5.474191317994603345 ) ) ;
#28062=CARTESIAN_POINT ( 'NONE',  ( 10.74482040370065228, -20.01237387469337392, -21.62860023531220577 ) ) ;
#28066=CARTESIAN_POINT ( 'NONE',  ( -13.82240055979716686, 28.15033208048753011, -10.03898445905979209 ) ) ;
#28067=CARTESIAN_POINT ( 'NONE',  ( -19.47283267323017597, -27.28889818631711250, -4.999999999999996447 ) ) ;
#28071=CARTESIAN_POINT ( 'NONE',  ( -19.56896045557411767, -6.106514739740910969, -30.00000000000000711 ) ) ;
#28072=CARTESIAN_POINT ( 'NONE',  ( -15.29981816934335548, -26.62016922504712468, -6.417125710678260653 ) ) ;
#28075=CARTESIAN_POINT ( 'NONE',  ( 24.08789872664181786, 1.422585201480351724, -18.55812312260739105 ) ) ;
#28080=CARTESIAN_POINT ( 'NONE',  ( -30.23117059640172144, -0.03771030696743234156, -8.764896985320813627 ) ) ;
#28082=CARTESIAN_POINT ( 'NONE',  ( 32.24877215592500335, -1.831602888277810814, -6.842981059139255251 ) ) ;
#28087=CARTESIAN_POINT ( 'NONE',  ( -22.72592367914349509, 4.308210353041426188, -18.81253349342975056 ) ) ;
#28095=AXIS2_PLACEMENT_3D ( 'NONE', #17632, #17018, #39343 ) ;
#28097=CARTESIAN_POINT ( 'NONE',  ( -24.85289228938016493, 7.121634862230863838, -5.000000000000001776 ) ) ;
#28101=CARTESIAN_POINT ( 'NONE',  ( 14.25810169807962424, -14.84648812655576045, -28.51942066398886055 ) ) ;
#28103=CARTESIAN_POINT ( 'NONE',  ( 13.89677717944467794, 24.25367973778722686, -13.48336797208005677 ) ) ;
#28106=CARTESIAN_POINT ( 'NONE',  ( -12.90278709585224348, 16.14496159291350352, -27.57500629962238747 ) ) ;
#28110=CARTESIAN_POINT ( 'NONE',  ( 15.35804996106242193, 26.54817030761798335, -6.888046620688911936 ) ) ;
#28114=CARTESIAN_POINT ( 'NONE',  ( -11.76301876381887368, 19.51941272550443429, -21.59238037788203357 ) ) ;
#28116=CARTESIAN_POINT ( 'NONE',  ( -15.47508831886704250, -26.54255591950745341, -7.353815494023745458 ) ) ;
#28120=CARTESIAN_POINT ( 'NONE',  ( -30.95555434509626025, -15.01264802092781281, -11.97973923657508699 ) ) ;
#28121=CARTESIAN_POINT ( 'NONE',  ( -14.53723555501347242, -26.50432973120043911, -5.000000000000000888 ) ) ;
#28123=CARTESIAN_POINT ( 'NONE',  ( 12.70988183501878055, 16.20822673541097458, -28.16655794507315491 ) ) ;
#28125=CARTESIAN_POINT ( 'NONE',  ( 23.45594209662042573, 4.561666950054395819, -16.77008761711584128 ) ) ;
#28131=CARTESIAN_POINT ( 'NONE',  ( -31.27312981421062688, -0.4309787749141145707, -4.999999999999999112 ) ) ;
#28132=CARTESIAN_POINT ( 'NONE',  ( 31.15015558338321711, -0.2976252405140638602, -5.000000000000000888 ) ) ;
#28138=CARTESIAN_POINT ( 'NONE',  ( -7.289639608743034849, -27.06962010326280321, -13.42901749168595060 ) ) ;
#28146=CARTESIAN_POINT ( 'NONE',  ( 3.842267464956742096, 37.63229749218292852, -7.124829648924612790 ) ) ;
#28147=DIRECTION ( 'NONE',  ( -0.000000000000000000, -0.000000000000000000, -1.000000000000000000 ) ) ;
#28155=CARTESIAN_POINT ( 'NONE',  ( 14.51296530378405336, 26.99756090190063773, -9.645496975165400499 ) ) ;
#28158=CARTESIAN_POINT ( 'NONE',  ( -17.72206997426596686, 16.40768990500343349, -13.83464017129110957 ) ) ;
#28162=CARTESIAN_POINT ( 'NONE',  ( 9.766980772230919428, -18.57228960779583815, -26.22661689184167955 ) ) ;
#28163=CARTESIAN_POINT ( 'NONE',  ( -21.99343813880628673, -26.08014713514513971, -8.986661558301907604 ) ) ;
#28164=CARTESIAN_POINT ( 'NONE',  ( 15.41782702884244571, 26.77676039938714325, -5.474246347568364257 ) ) ;
#28165=CARTESIAN_POINT ( 'NONE',  ( 15.16872908693824407, 26.30108831384980661, -8.297102614751414862 ) ) ;
#28169=CARTESIAN_POINT ( 'NONE',  ( -9.922080038078478381, -18.83169384875433039, -25.01962877829346965 ) ) ;
#28172=CARTESIAN_POINT ( 'NONE',  ( -21.16141018750222713, -14.58779178538210175, -19.64528038461644499 ) ) ;
#28173=CARTESIAN_POINT ( 'NONE',  ( -0.3069599879515859109, -21.90886338974817349, -20.12108918057204221 ) ) ;
#28174=CARTESIAN_POINT ( 'NONE',  ( 15.11801385582561963, 24.79072481137326278, -10.19584184461111143 ) ) ;
#28175=CARTESIAN_POINT ( 'NONE',  ( 18.36494381186184910, 9.412039940421420781, -27.17404324301481111 ) ) ;
#28178=CARTESIAN_POINT ( 'NONE',  ( -29.25378966048014107, -3.741898191150933695, -14.12891680041362363 ) ) ;
#28185=CARTESIAN_POINT ( 'NONE',  ( -20.46571904345125148, 1.196608941699672135, -29.35443162036549580 ) ) ;
#28186=CARTESIAN_POINT ( 'NONE',  ( 35.25372542428971201, -14.20602460021386193, -5.437452493555934296 ) ) ;
#28196=CARTESIAN_POINT ( 'NONE',  ( -2.246677149408780494, 20.47173499388784990, -28.45538990901911447 ) ) ;
#28197=CARTESIAN_POINT ( 'NONE',  ( -35.48538791413474769, -11.24999995268676933, -5.000000000000001776 ) ) ;
#28204=CARTESIAN_POINT ( 'NONE',  ( 13.71665722575384194, 30.74286335228606148, -5.909757821034641978 ) ) ;
#28207=CARTESIAN_POINT ( 'NONE',  ( -20.36441849243354696, 12.17262094050481913, -12.89086137884393324 ) ) ;
#28209=CARTESIAN_POINT ( 'NONE',  ( 15.21101220493249251, -26.17680776644541041, -8.762161127626081125 ) ) ;
#28211=CARTESIAN_POINT ( 'NONE',  ( 12.35927980519502611, 20.53300710371609838, -19.48961259234621934 ) ) ;
#28212=CARTESIAN_POINT ( 'NONE',  ( 12.33616729053617966, -27.99489201236593416, -5.000000000000000000 ) ) ;
#28214=CARTESIAN_POINT ( 'NONE',  ( -23.90157044124041263, -25.28113828194042867, -9.382323413831949566 ) ) ;
#28215=CARTESIAN_POINT ( 'NONE',  ( 10.81257536403207276, -22.55273985443259477, -16.57830297862439295 ) ) ;
#28216=CARTESIAN_POINT ( 'NONE',  ( 15.45156861522514369, 26.56435632827706428, -5.946109696244072040 ) ) ;
#28217=CARTESIAN_POINT ( 'NONE',  ( 21.69387525390884264, -15.65483690961669261, -18.63891047137795098 ) ) ;
#28221=CARTESIAN_POINT ( 'NONE',  ( -10.25240473134331154, 34.56179556857796342, -6.747403775044807261 ) ) ;
#28222=CARTESIAN_POINT ( 'NONE',  ( -14.29712391636367563, -26.44587280164909870, -4.999999999999999112 ) ) ;
#28228=CARTESIAN_POINT ( 'NONE',  ( 29.56235616742567629, 0.08762005067959190152, -10.18130632035143535 ) ) ;
#28230=CARTESIAN_POINT ( 'NONE',  ( -12.26832665498866071, 32.91590888319122854, -4.999999999999996447 ) ) ;
#28235=CARTESIAN_POINT ( 'NONE',  ( -30.82577771627267182, 0.002281058920265444448, -5.946086761298152723 ) ) ;
#28236=CARTESIAN_POINT ( 'NONE',  ( -20.24725037384592952, -26.82317351678327810, -7.696457708727984404 ) ) ;
#28238=CARTESIAN_POINT ( 'NONE',  ( 25.22840985194761387, -4.440669541368661655, -18.96303409332410084 ) ) ;
#28244=DIRECTION ( 'NONE',  ( 0.000000000000000000, 0.000000000000000000, 1.000000000000000000 ) ) ;
#28250=CARTESIAN_POINT ( 'NONE',  ( -20.46375980781524007, 1.787259394981456362, -30.00000000000000711 ) ) ;
#28256=CARTESIAN_POINT ( 'NONE',  ( 17.96157960088948613, 18.73973607591619839, -8.370532139170391517 ) ) ;
#28257=CARTESIAN_POINT ( 'NONE',  ( 4.686106015904482724, 20.84698696610319146, -25.69044758121691885 ) ) ;
#28258=CARTESIAN_POINT ( 'NONE',  ( 17.52734727169944406, -27.07761244028429459, -6.386038267470317109 ) ) ;
#28262=CARTESIAN_POINT ( 'NONE',  ( -11.50355825530538212, 18.42073213090798944, -23.85688228919889653 ) ) ;
#28265=CARTESIAN_POINT ( 'NONE',  ( 12.78263182082741523, -23.08026933373198020, -15.46555305964894167 ) ) ;
#28268=ORIENTED_EDGE ( 'NONE', *, *, #23047, .F. ) ;
#28269=CARTESIAN_POINT ( 'NONE',  ( -12.94388269583936513, 26.17419193811465661, -13.31610081608094198 ) ) ;
#28270=CARTESIAN_POINT ( 'NONE',  ( -17.57421241049386396, -24.84107886702332380, -12.30910806047397088 ) ) ;
#28274=CARTESIAN_POINT ( 'NONE',  ( -19.75415558344636580, -5.512529345569482153, -29.24332315753316891 ) ) ;
#28275=CARTESIAN_POINT ( 'NONE',  ( -9.518731748684004401, -18.39049943551870925, -27.45506815792052180 ) ) ;
#28278=CARTESIAN_POINT ( 'NONE',  ( 29.81424496809705715, 0.2234756960255703251, -9.241590868339290665 ) ) ;
#28283=CARTESIAN_POINT ( 'NONE',  ( -25.88842680114331785, 0.2780094573818647219, -16.43839041040183702 ) ) ;
#28285=CARTESIAN_POINT ( 'NONE',  ( 21.07046404024911013, -0.6704196337341807865, -26.09432862330225333 ) ) ;
#28299=CARTESIAN_POINT ( 'NONE',  ( -20.76109417526653544, 8.238746406137220646, -19.01874696799055897 ) ) ;
#28300=CARTESIAN_POINT ( 'NONE',  ( 13.97675284653878691, -15.47333779752018756, -27.13317248147880534 ) ) ;
#28302=CARTESIAN_POINT ( 'NONE',  ( 13.13589401999236550, 22.37095606609392462, -16.42714977293202949 ) ) ;
#28304=CARTESIAN_POINT ( 'NONE',  ( -16.06107056606509786, 23.80089718141779898, -7.844701006372616803 ) ) ;
#28307=CARTESIAN_POINT ( 'NONE',  ( 11.07396762549639746, 17.40261846349473984, -28.07943001733049115 ) ) ;
#28311=CARTESIAN_POINT ( 'NONE',  ( -10.86943063858312364, 17.38123995523577037, -29.99999999999998934 ) ) ;
#28313=CARTESIAN_POINT ( 'NONE',  ( -14.95650897399027990, -25.69867652498056643, -10.16863992578564613 ) ) ;
#28317=CARTESIAN_POINT ( 'NONE',  ( -20.52236299606704151, -9.986717880826434524, -22.99756460869029340 ) ) ;
#28318=CARTESIAN_POINT ( 'NONE',  ( -10.90147648380924927, -21.05887150913213191, -19.56414284889322630 ) ) ;
#28320=CARTESIAN_POINT ( 'NONE',  ( 13.45249047345274640, 17.67863091976945000, -21.86233792381201724 ) ) ;
#28322=CARTESIAN_POINT ( 'NONE',  ( 21.14860408002057568, 5.266143715497261013, -22.06585488323975142 ) ) ;
#28328=CARTESIAN_POINT ( 'NONE',  ( -24.22435077138248616, -0.2007882836984510588, -19.40349160117432703 ) ) ;
#28329=CARTESIAN_POINT ( 'NONE',  ( 24.71184492219473228, 0.1155084257449812690, -18.40944145481854832 ) ) ;
#28332=CARTESIAN_POINT ( 'NONE',  ( -5.636483973512888213, -22.01575377102104625, -29.99999999999999645 ) ) ;
#28336=AXIS2_PLACEMENT_3D ( 'NONE', #200, #15638, #24380 ) ;
#28340=CARTESIAN_POINT ( 'NONE',  ( 4.649262579009291407, 28.36936852218387983, -16.68779215659397153 ) ) ;
#28348=CARTESIAN_POINT ( 'NONE',  ( 11.04586147422109477, 19.50284389929768381, -22.62640361410345236 ) ) ;
#28352=CARTESIAN_POINT ( 'NONE',  ( -18.23749494249763003, 18.64175607586350480, -6.439786763766045752 ) ) ;
#28356=CARTESIAN_POINT ( 'NONE',  ( 14.34475445268075156, -25.06822468207680288, -11.59938494084682326 ) ) ;
#28358=DIRECTION ( 'NONE',  ( -0.000000000000000000, -0.000000000000000000, -1.000000000000000000 ) ) ;
#28359=CARTESIAN_POINT ( 'NONE',  ( 13.49046931713162145, 22.81729818279096023, -15.45058010560173045 ) ) ;
#28360=CARTESIAN_POINT ( 'NONE',  ( 13.47891791608170209, 22.84109221470872697, -15.44783060290720300 ) ) ;
#28363=CARTESIAN_POINT ( 'NONE',  ( -9.719952024558851988, -18.59326785210745925, -26.23105664925188307 ) ) ;
#28365=CARTESIAN_POINT ( 'NONE',  ( -31.58328445775233106, -21.78494312990649462, -5.436021537729467390 ) ) ;
#28366=CARTESIAN_POINT ( 'NONE',  ( -4.072631098700577823, -22.66826574189022381, -16.93478912211341481 ) ) ;
#28367=CARTESIAN_POINT ( 'NONE',  ( 15.55049802031632034, 25.65338682851541563, -7.361195678376786233 ) ) ;
#28369=CARTESIAN_POINT ( 'NONE',  ( 22.79531528405124163, 10.15988774222570434, -4.999999999999998224 ) ) ;
#28373=CARTESIAN_POINT ( 'NONE',  ( -33.52901403654990276, -3.501605748354566394, -5.000000000000002665 ) ) ;
#28383=CARTESIAN_POINT ( 'NONE',  ( -24.37716644428920887, 0.8142858702769540935, -18.49331350387625150 ) ) ;
#28384=B_SPLINE_CURVE_WITH_KNOTS ( 'NONE', 3,
 ( #1319, #25484, #19004, #28740, #32200, #25298, #10058, #6994, #6794, #22437 ),
 .UNSPECIFIED., .F., .F.,
 ( 4, 2, 2, 2, 4 ),
 ( 0.000000000000000000, 0.2500000000000000000, 0.5000000000000000000, 0.7500000000000000000, 1.000000000000000000 ),
 .UNSPECIFIED. ) ;
#28385=CARTESIAN_POINT ( 'NONE',  ( 25.71601288570474253, -10.35479112961458092, -17.64613853693563073 ) ) ;
#28394=CARTESIAN_POINT ( 'NONE',  ( -2.693587759434362461, 33.22306132784108001, -12.89973256833978787 ) ) ;
#28400=EDGE_CURVE ( 'NONE', #32508, #15787, #26702, .T. ) ;
#28403=CARTESIAN_POINT ( 'NONE',  ( 12.56655098099258794, 27.87547247283417917, -12.29340594856549984 ) ) ;
#28406=CARTESIAN_POINT ( 'NONE',  ( -18.00818492405559823, 9.835074072281088320, -28.86228936887301089 ) ) ;
#28408=CARTESIAN_POINT ( 'NONE',  ( 13.76081720998434221, -24.12408036951367762, -13.50911283364834681 ) ) ;
#28410=CARTESIAN_POINT ( 'NONE',  ( 13.73332615291622005, 23.47756605762641868, -14.46771515761556337 ) ) ;
#28411=CARTESIAN_POINT ( 'NONE',  ( 11.41987377193677489, -19.41918266173338026, -30.00000000000000000 ) ) ;
#28412=CYLINDRICAL_SURFACE ( 'NONE', #5122, 17.00000000000000711 ) ;
#28414=CARTESIAN_POINT ( 'NONE',  ( -14.21852471880019664, -15.07395324936907954, -27.81797908992425761 ) ) ;
#28415=CARTESIAN_POINT ( 'NONE',  ( 8.079555417519777905, -24.49239216019507026, -10.79927774074996094 ) ) ;
#28416=CARTESIAN_POINT ( 'NONE',  ( 15.40046916436526558, 26.40062519190980694, -6.888357274586806689 ) ) ;
#28417=CARTESIAN_POINT ( 'NONE',  ( 19.98114792981366961, -14.40613482780026722, -20.72081132955061022 ) ) ;
#28421=CARTESIAN_POINT ( 'NONE',  ( -7.254375287122624805, 27.20239578260290259, -16.79518470217901438 ) ) ;
#28425=CARTESIAN_POINT ( 'NONE',  ( 25.23308087229151653, 0.3395914844611204186, -17.43355021032456875 ) ) ;
#28426=CARTESIAN_POINT ( 'NONE',  ( -8.301277145684272440, 36.28737808747504801, -5.000000000000000000 ) ) ;
#28429=ADVANCED_FACE ( 'NONE', ( #18317 ), #4969, .T. ) ;
#28431=CARTESIAN_POINT ( 'NONE',  ( -28.30077390381833879, 0.1879860857717292055, -12.55250302845952071 ) ) ;
#28434=CARTESIAN_POINT ( 'NONE',  ( 35.00061772621288725, -7.347685171788704395, -5.885183883027742091 ) ) ;
#28447=CARTESIAN_POINT ( 'NONE',  ( 8.988510393147455702, 18.42811980848636821, -30.00000000000000000 ) ) ;
#28451=CARTESIAN_POINT ( 'NONE',  ( 17.40746082178494447, 19.58779920104105088, -9.330282795758028769 ) ) ;
#28452=CARTESIAN_POINT ( 'NONE',  ( 5.245966764456291287, 20.42028367153013235, -26.38657226523553945 ) ) ;
#28454=CARTESIAN_POINT ( 'NONE',  ( 16.47100665901824001, -26.88200473344899066, -6.401141426531012257 ) ) ;
#28459=CARTESIAN_POINT ( 'NONE',  ( -11.69322940238108188, 18.90460750012263347, -22.73643640026262247 ) ) ;
#28462=CARTESIAN_POINT ( 'NONE',  ( 9.372336683666530277, -18.28158583912481916, -28.71275810336947742 ) ) ;
#28467=CARTESIAN_POINT ( 'NONE',  ( -8.885346522200764596, 20.34420481528383817, -23.48319193123574067 ) ) ;
#28470=CARTESIAN_POINT ( 'NONE',  ( -30.09940253797056897, -9.337810905337370571, -13.89521527110805188 ) ) ;
#28471=CARTESIAN_POINT ( 'NONE',  ( -9.394881763177457046, -18.22048488343288142, -30.00000000000000000 ) ) ;
#28474=CARTESIAN_POINT ( 'NONE',  ( 20.55243914501509650, 1.720701587877496275, -28.11989156925753974 ) ) ;
#28479=CARTESIAN_POINT ( 'NONE',  ( -24.58066270203448411, 0.3884518765734885637, -18.44634674746681569 ) ) ;
#28482=CARTESIAN_POINT ( 'NONE',  ( 32.40677704871944087, -1.850583768531564033, -5.924515326665249937 ) ) ;
#28493=B_SPLINE_SURFACE_WITH_KNOTS ( 'NONE', 3, 3, ( 
 ( #5281, #27219, #2046, #33734 ),
 ( #17695, #17493, #18282, #36563 ),
 ( #36368, #2837, #26818, #21125 ),
 ( #24370, #39404, #33534, #5678 ),
 ( #23972, #18089, #8532, #15228 ),
 ( #15025, #20926, #40000, #33334 ),
 ( #30477, #27614, #27416, #20531 ),
 ( #36766, #5084, #5478, #37564 ),
 ( #31267, #587, #9536, #12575 ),
 ( #12969, #21717, #37761, #391 ),
 ( #12771, #27818, #21518, #9931 ),
 ( #6665, #25359, #19264, #24765 ),
 ( #9734, #21914, #37161, #3429 ),
 ( #3033, #34119, #31664, #33921 ),
 ( #9133, #16024, #15826, #28411 ),
 ( #28212, #34713, #22117, #18876 ),
 ( #22313, #31071, #6077, #6865 ),
 ( #15628, #18481, #34515, #30872 ),
 ( #3830, #16229, #15427, #18679 ),
 ( #13230, #28613, #12376, #3235 ),
 ( #12179, #24573, #36967, #9336 ),
 ( #6276, #28013, #25167, #187 ),
 ( #24967, #37361, #34317, #6471 ),
 ( #19073, #31464, #3629, #10944 ),
 ( #4435, #25559, #23329, #32682 ),
 ( #26369, #16634, #32481, #16838 ),
 ( #13773, #25760, #28815, #35314 ),
 ( #38157, #10734, #32062, #10329 ),
 ( #19880, #35518, #35725, #7266 ),
 ( #4836, #20084, #7877, #38358 ),
 ( #13978, #1595, #22709, #38762 ),
 ( #32269, #29015, #35114, #1191 ),
 ( #10131, #20282, #37960, #13571 ),
 ( #17246, #22506, #4636, #31861 ),
 ( #23119, #13166, #17038, #34917 ),
 ( #13372, #7682, #4232, #19668 ),
 ( #29418, #26166, #7473, #38560 ),
 ( #29219, #783, #10530, #25958 ),
 ( #1389, #22913, #7068, #19466 ),
 ( #4024, #16425, #990, #30024 ),
 ( #38965, #11938, #26575, #2200 ),
 ( #5036, #21083, #35921, #5839 ),
 ( #17448, #29618, #39564, #39160 ),
 ( #32884, #14383, #11740, #11342 ) ),
 .UNSPECIFIED., .T., .F., .F.,
 ( 4, 1, 1, 1, 2, 1, 1, 1, 1, 1, 1, 1, 2, 1, 1, 1, 2, 1, 1, 1, 1, 1, 1, 1, 2, 1, 1, 1, 2, 1, 1, 1, 1, 1, 1, 1, 4 ),
 ( 4, 4 ),
 ( 0.000000000000000000, 0.03553882639362128393, 0.07107765278724256786, 0.1066164791808638657, 0.1421553055744851357, 0.1660525590443411859, 0.1899498125141971805, 0.2138470659840532306, 0.2377443194539092253, 0.2616415729237652754, 0.2855388263936212701, 0.3094360798634773202, 0.3333333333333333703, 0.3688721597269547514, 0.4044109861205760215, 0.4399498125141973470, 0.4754886389078186171, 0.4993858923776745562, 0.5232831458475305508, 0.5471803993173864900, 0.5710776527872425401, 0.5949749062570985902, 0.6188721597269547514, 0.6427694131968104685, 0.6666666666666665186, 0.7022054930602876777, 0.7377443194539090587, 0.7732831458475302178, 0.8088219722411513768, 0.8327192257110074269, 0.8566164791808634771, 0.8805137326507195272, 0.9044109861205756884, 0.9283082395904318496, 0.9522054930602878997, 0.9761027465301439499, 1.000000000000000000 ),
 ( 0.000000000000000000, 1.000000000000000000 ),
 .UNSPECIFIED. ) ;
#28498=CARTESIAN_POINT ( 'NONE',  ( -22.89598029550568015, 9.861910665086448091, -6.936501474781229248 ) ) ;
#28499=CARTESIAN_POINT ( 'NONE',  ( 22.29802552750217259, -25.97160884719322738, -8.980211844774188990 ) ) ;
#28501=CARTESIAN_POINT ( 'NONE',  ( 13.94130713879165562, 24.14927663816028058, -13.49308697109902511 ) ) ;
#28503=CARTESIAN_POINT ( 'NONE',  ( -13.04719345707401779, 18.83419094417813255, -20.69477310159956573 ) ) ;
#28507=CARTESIAN_POINT ( 'NONE',  ( 12.95272860106239499, 21.61356709058502545, -17.44179881794794795 ) ) ;
#28509=CARTESIAN_POINT ( 'NONE',  ( 31.49474942026707325, -16.12477659677660569, -11.06936912200789180 ) ) ;
#28512=CARTESIAN_POINT ( 'NONE',  ( -13.67015811309539153, 23.61746135327068075, -14.45312116646361211 ) ) ;
#28514=CARTESIAN_POINT ( 'NONE',  ( -11.00685563857638449, -19.43747507878832437, -22.67326838232596131 ) ) ;
#28518=CARTESIAN_POINT ( 'NONE',  ( -29.13733599210751990, -14.13474271335126708, -13.81261361319337055 ) ) ;
#28519=CARTESIAN_POINT ( 'NONE',  ( -14.48060417942811817, -26.41903408085133265, -6.418214492182147346 ) ) ;
#28521=CARTESIAN_POINT ( 'NONE',  ( 16.33296907320687552, 23.02383901948744338, -7.850688138034399799 ) ) ;
#28523=CARTESIAN_POINT ( 'NONE',  ( 25.95036642640170754, 5.573903512884414546, -6.435863300068679571 ) ) ;
#28530=CARTESIAN_POINT ( 'NONE',  ( -22.30193131537437168, 0.3262574266873361495, -22.69144778596356460 ) ) ;
#28532=CARTESIAN_POINT ( 'NONE',  ( 29.89909462720550692, -0.2920382172860754855, -10.15462489924079570 ) ) ;
#28535=CARTESIAN_POINT ( 'NONE',  ( -21.88499642459564498, -5.528038495964382015, -20.11584339644715413 ) ) ;
#28543=CARTESIAN_POINT ( 'NONE',  ( 2.081989859667413345, 20.63897288273475894, -27.71951656526475460 ) ) ;
#28549=CARTESIAN_POINT ( 'NONE',  ( 16.71272696259839918, -12.03478187020944645, -28.45356395895326074 ) ) ;
#28554=CARTESIAN_POINT ( 'NONE',  ( 11.08575732160469052, 18.77318094934662795, -23.79130904447407246 ) ) ;
#28557=CARTESIAN_POINT ( 'NONE',  ( -18.44765746950383800, 17.30723153088500155, -9.360930369442520771 ) ) ;
#28560=CARTESIAN_POINT ( 'NONE',  ( 11.15896920475388043, -20.47308817170501172, -20.54455431084991446 ) ) ;
#28562=CARTESIAN_POINT ( 'NONE',  ( 11.07693200130355038, 17.49985971445773458, -27.44810509905307683 ) ) ;
#28564=CARTESIAN_POINT ( 'NONE',  ( 14.93061682650073330, 25.81337123915155729, -9.708168291266565220 ) ) ;
#28567=CARTESIAN_POINT ( 'NONE',  ( -9.575915756022620684, -18.36279351651394620, -27.45102388653645065 ) ) ;
#28570=CARTESIAN_POINT ( 'NONE',  ( -30.73942927727400232, -22.61273690771325917, -5.858838859916063235 ) ) ;
#28571=CARTESIAN_POINT ( 'NONE',  ( -4.793034356438155008, -24.87474678070748269, -6.447031815283989609 ) ) ;
#28572=CARTESIAN_POINT ( 'NONE',  ( 15.71155925927456742, 25.50991634872312730, -6.418619526760371841 ) ) ;
#28574=CARTESIAN_POINT ( 'NONE',  ( 20.22334892891204561, 9.255629639704887168, -19.04855246831971982 ) ) ;
#28578=CARTESIAN_POINT ( 'NONE',  ( -20.28315073442723460, -3.046437751679770933, -29.27849696980957717 ) ) ;
#28585=CARTESIAN_POINT ( 'NONE',  ( -25.39634053522611623, 1.114860656254929028, -16.51261428875549697 ) ) ;
#28586=CARTESIAN_POINT ( 'NONE',  ( 21.10775083282109676, -8.526917100706684849, -23.04258616691868511 ) ) ;
#28595=CARTESIAN_POINT ( 'NONE',  ( -1.044308797982332448, 21.12605994883989879, -26.25946094505387407 ) ) ;
#28600=CARTESIAN_POINT ( 'NONE',  ( 20.23296131041715640, 28.12381335138032412, 0.000000000000000000 ) ) ;
#28602=CARTESIAN_POINT ( 'NONE',  ( 13.99156332179505569, 29.21683596761936741, -8.194172333430742583 ) ) ;
#28604=EDGE_LOOP ( 'NONE', ( #38405, #25693, #3535, #9301, #8714, #20110, #5338, #23322, #11065, #15505 ) ) ;
#28605=CARTESIAN_POINT ( 'NONE',  ( -19.96221307476523421, 10.82707266035624372, -16.98081666870033146 ) ) ;
#28607=CARTESIAN_POINT ( 'NONE',  ( 0.000000000000000000, 22.50000000000000355, 6.000000000000000000 ) ) ;
#28609=CARTESIAN_POINT ( 'NONE',  ( 14.93595915082604186, -25.84735051801111894, -9.705674759444587352 ) ) ;
#28612=CARTESIAN_POINT ( 'NONE',  ( 13.17886393423189162, 22.29227785210140311, -16.43698232960724681 ) ) ;
#28613=CARTESIAN_POINT ( 'NONE',  ( -12.33616729053607486, -27.99489201236593061, -13.58461195433496194 ) ) ;
#28615=CARTESIAN_POINT ( 'NONE',  ( -20.53646817104797506, -21.76128887135726231, -14.90463942194158520 ) ) ;
#28616=CARTESIAN_POINT ( 'NONE',  ( 8.419895509524939925, -25.16897077364957269, -7.395897382025212075 ) ) ;
#28617=CARTESIAN_POINT ( 'NONE',  ( 12.51756012225011894, 20.32411358514038113, -19.51841735849092174 ) ) ;
#28618=CARTESIAN_POINT ( 'NONE',  ( 30.90226151228388574, -22.30983874898413788, -6.280244427829897447 ) ) ;
#28621=B_SPLINE_CURVE_WITH_KNOTS ( 'NONE', 3,
 ( #9206, #3108, #15899, #27888, #22183, #24839, #463, #6736, #25428, #18551, #37825, #3504, #3304, #15501, #37434, #24640, #21590, #60, #5951, #15298, #37237, #6344, #34191, #6540, #30748, #21989, #9608, #18751, #15694, #262, #12649, #25037, #34389, #18945, #12847, #38234, #34991, #25835, #25629, #29088, #35593, #7140, #38027, #26034, #19747, #10201, #29292, #10405, #7750, #26239, #7549, #1061, #19342, #10606, #3899, #28885, #1462, #13847, #13238, #4099 ),
 .UNSPECIFIED., .F., .F.,
 ( 4, 2, 2, 2, 2, 2, 2, 2, 2, 2, 2, 2, 2, 2, 2, 2, 2, 2, 2, 2, 2, 2, 2, 2, 2, 2, 2, 2, 2, 4 ),
 ( 0.000000000000000000, 0.004090388079386704165, 0.006135582119080056247, 0.008180776158773408330, 0.01227116423816010903, 0.01329376125800678550, 0.01431635827785346024, 0.01636155231754680972, 0.02045194039693351215, 0.02249713443662685469, 0.02454232847632019723, 0.02658752251601354671, 0.02863271655570688926, 0.03272310463509358475, 0.03374570165494025775, 0.03476829867478693076, 0.03681349271448028371, 0.04090388079386698961, 0.04192647781371366261, 0.04294907483356033562, 0.04499426887325368857, 0.04703946291294704152, 0.04908465695264038753, 0.05317504503202709343, 0.05522023907172043944, 0.05726543311141379239, 0.06135582119080049829, 0.06237841821064717823, 0.06340101523049386512, 0.06544620927018722500 ),
 .UNSPECIFIED. ) ;
#28623=CARTESIAN_POINT ( 'NONE',  ( -8.411768547097867810, 35.89333961072667023, -6.727922225057652028 ) ) ;
#28627=CARTESIAN_POINT ( 'NONE',  ( 23.94456298200180910, 0.4764677600133929158, -19.49540907187814298 ) ) ;
#28633=CARTESIAN_POINT ( 'NONE',  ( -20.60555239772964242, 0.9311154778176756741, -28.08151642131643655 ) ) ;
#28636=CARTESIAN_POINT ( 'NONE',  ( 29.16726107428658565, -7.828744422222867705, -14.86866462477206419 ) ) ;
#28650=CARTESIAN_POINT ( 'NONE',  ( 18.14143768169351034, 18.99352574702872687, -5.478296980462506127 ) ) ;
#28651=CARTESIAN_POINT ( 'NONE',  ( 5.348610690096846199, 23.76848409712731325, -20.84344495567194500 ) ) ;
#28656=CARTESIAN_POINT ( 'NONE',  ( 16.27219429315636390, -26.92618254030204383, -5.000000000000002665 ) ) ;
#28660=CARTESIAN_POINT ( 'NONE',  ( -11.00242421671864790, 17.29730523913238827, -29.99999999999999645 ) ) ;
#28662=CARTESIAN_POINT ( 'NONE',  ( 11.24122865112338410, -21.01550894017544380, -19.52903937763365150 ) ) ;
#28665=EDGE_LOOP ( 'NONE', ( #9760, #32499, #17557, #29856 ) ) ;
#28667=CARTESIAN_POINT ( 'NONE',  ( -12.95981342954301496, 28.24763295269045926, -11.37950637273800325 ) ) ;
#28670=CARTESIAN_POINT ( 'NONE',  ( -21.28402897910519442, -4.571266421688831016, -24.49177716778804381 ) ) ;
#28673=CARTESIAN_POINT ( 'NONE',  ( 21.68786324554740474, 0.8396193639690311405, -23.86711573477778003 ) ) ;
#28677=CARTESIAN_POINT ( 'NONE',  ( -20.48278845350746380, 0.8398715278162421916, -29.34801594207987208 ) ) ;
#28681=CARTESIAN_POINT ( 'NONE',  ( 21.08291815013172155, -1.666117999273566186, -26.00856586672298221 ) ) ;
#28695=CARTESIAN_POINT ( 'NONE',  ( -21.15495209035839963, 9.289218443130405234, -15.92845176507750793 ) ) ;
#28697=CARTESIAN_POINT ( 'NONE',  ( 17.25312817826965883, -20.19401662141811116, -17.91462702624227532 ) ) ;
#28701=CARTESIAN_POINT ( 'NONE',  ( 10.88003517233900297, 17.37455259072008573, -29.34610220216738696 ) ) ;
#28702=EDGE_LOOP ( 'NONE', ( #1948, #35030, #23568, #16039 ) ) ;
#28703=CARTESIAN_POINT ( 'NONE',  ( -15.22475464391910549, 24.92285436334850601, -9.722768853599610850 ) ) ;
#28706=CARTESIAN_POINT ( 'NONE',  ( 11.34078712063792160, 18.01401842891820948, -25.01870591048817261 ) ) ;
#28708=CARTESIAN_POINT ( 'NONE',  ( 25.87747567411906502, -13.26005397570095035, -16.62966469873034114 ) ) ;
#28709=CARTESIAN_POINT ( 'NONE',  ( -19.48557158514988785, -11.24999999999987743, 6.000000000000000000 ) ) ;
#28711=CARTESIAN_POINT ( 'NONE',  ( -15.27795965409528556, 27.25395738312943195, -5.000000000000000888 ) ) ;
#28713=CARTESIAN_POINT ( 'NONE',  ( -10.10041478618032151, -18.75911771733305144, -24.99883724396762474 ) ) ;
#28717=CARTESIAN_POINT ( 'NONE',  ( -19.51443761669260013, -8.089147095777512675, -26.29262032055718734 ) ) ;
#28718=CARTESIAN_POINT ( 'NONE',  ( -9.200702945070620586, -18.66544396913702286, -26.87043342310872518 ) ) ;
#28720=CARTESIAN_POINT ( 'NONE',  ( 16.07775879733624080, 22.56051826075340827, -9.762945716588777856 ) ) ;
#28722=CARTESIAN_POINT ( 'NONE',  ( 20.01208193039519756, 4.507116686654149440, -30.00000000000000355 ) ) ;
#28724=ORIENTED_EDGE ( 'NONE', *, *, #27998, .F. ) ;
#28725=CARTESIAN_POINT ( 'NONE',  ( -31.18229473435558319, -0.3319675162687186210, -5.472313823790837084 ) ) ;
#28727=CARTESIAN_POINT ( 'NONE',  ( 31.12965019444430226, -0.3871312522807165979, -6.409569423096037610 ) ) ;
#28731=ORIENTED_EDGE ( 'NONE', *, *, #30354, .F. ) ;
#28732=CARTESIAN_POINT ( 'NONE',  ( -5.636483973512888213, -22.01575377102104270, -21.50719306941231679 ) ) ;
#28740=CARTESIAN_POINT ( 'NONE',  ( 24.10033869685532082, 8.113510327255378130, -5.000000000000000888 ) ) ;
#28746=CARTESIAN_POINT ( 'NONE',  ( 21.57777642674768614, -18.77388931612815171, -16.71433531468114708 ) ) ;
#28752=CARTESIAN_POINT ( 'NONE',  ( 14.64031184850172806, 26.19941073413151500, -10.14528853390185859 ) ) ;
#28756=CARTESIAN_POINT ( 'NONE',  ( -14.53439070480614603, 14.74270464415775628, -27.08252300681113667 ) ) ;
#28759=CARTESIAN_POINT ( 'NONE',  ( 13.35281424139188999, -23.62076856857055063, -14.47731724256479247 ) ) ;
#28761=CARTESIAN_POINT ( 'NONE',  ( 15.02387404494793088, 25.95058579368609841, -9.238541711895710051 ) ) ;
#28763=CARTESIAN_POINT ( 'NONE',  ( 12.38717450789916974, 20.49561646409227578, -19.49553371946326763 ) ) ;
#28765=CARTESIAN_POINT ( 'NONE',  ( -12.61875268155488961, 21.10517070559246378, -18.44458008985245456 ) ) ;
#28767=CARTESIAN_POINT ( 'NONE',  ( -15.27591890422142740, -26.49336055367123066, -7.358011338661719414 ) ) ;
#28770=CARTESIAN_POINT ( 'NONE',  ( -29.20118438018936757, -21.52094793055072230, -9.738337299848499384 ) ) ;
#28772=CARTESIAN_POINT ( 'NONE',  ( -3.274116759621854111, -20.28896347757955354, -30.00000000000000000 ) ) ;
#28773=CARTESIAN_POINT ( 'NONE',  ( 12.28356143704143477, 18.96473258983586518, -21.68345190119157806 ) ) ;
#28775=CARTESIAN_POINT ( 'NONE',  ( 24.01170615723790647, 8.305688554546300395, -5.962680836947249041 ) ) ;
#28779=CARTESIAN_POINT ( 'NONE',  ( -20.53764066314045778, -2.436979956095350897, -27.91568385910457906 ) ) ;
#28788=CARTESIAN_POINT ( 'NONE',  ( 34.65956455088738153, -16.45432426470986798, -5.436012016185657103 ) ) ;
#28790=ORIENTED_EDGE ( 'NONE', *, *, #25883, .T. ) ;
#28797=CARTESIAN_POINT ( 'NONE',  ( -1.457936558815239314, 29.04007097956189654, -16.62967044460848598 ) ) ;
#28798=CARTESIAN_POINT ( 'NONE',  ( -30.90412082983564446, -0.04211290444597337590, -5.000000000000000888 ) ) ;
#28803=AXIS2_PLACEMENT_3D ( 'NONE', #33773, #21961, #18522 ) ;
#28804=CARTESIAN_POINT ( 'NONE',  ( 13.32202332345313067, 27.64393215917316482, -11.41592897530081707 ) ) ;
#28807=CARTESIAN_POINT ( 'NONE',  ( -18.97453683301921856, 13.61319736012170445, -14.90564131719889218 ) ) ;
#28812=CARTESIAN_POINT ( 'NONE',  ( 9.532625661562562414, -18.14880370279404076, -29.34763336998847905 ) ) ;
#28814=CARTESIAN_POINT ( 'NONE',  ( 15.34998332328284931, 26.75042238537495720, -6.415952016425999993 ) ) ;
#28815=CARTESIAN_POINT ( 'NONE',  ( -21.88499642459564498, -5.528038495964382015, -20.11584339644715413 ) ) ;
#28818=CARTESIAN_POINT ( 'NONE',  ( -24.91750628164249903, -24.86351076958389328, -9.360757952822334360 ) ) ;
#28819=CARTESIAN_POINT ( 'NONE',  ( 6.046104871185695728, -24.56383547664059819, -9.847241658924353658 ) ) ;
#28820=CARTESIAN_POINT ( 'NONE',  ( 15.42174346112090966, 26.32695858896734364, -6.888516504560381115 ) ) ;
#28821=CARTESIAN_POINT ( 'NONE',  ( 31.56478557840102539, -21.36326414210120817, -6.699604253589384051 ) ) ;
#28822=CARTESIAN_POINT ( 'NONE',  ( -19.48557158514998022, -11.24999999999982414, 0.000000000000000000 ) ) ;
#28825=CARTESIAN_POINT ( 'NONE',  ( -8.315359605991371694, 35.38416871997877422, -8.021598471839368472 ) ) ;
#28829=CARTESIAN_POINT ( 'NONE',  ( 20.48245044547724447, 0.8483310608570678868, -29.34817008848411035 ) ) ;
#28833=CARTESIAN_POINT ( 'NONE',  ( -28.25918702355578915, 0.2404301350531496129, -12.55492373771259373 ) ) ;
#28836=CARTESIAN_POINT ( 'NONE',  ( 33.69202569405961611, -9.057028871410325976, -9.807891961042667361 ) ) ;
#28837=AXIS2_PLACEMENT_3D ( 'NONE', #26412, #11384, #20925 ) ;
#28838=EDGE_LOOP ( 'NONE', ( #2618, #34786, #37614, #4846 ) ) ;
#28844=CIRCLE ( 'NONE', #39232, 21.00000000000001776 ) ;
#28851=CARTESIAN_POINT ( 'NONE',  ( 16.49490170946486955, 16.68252506057627116, -16.84766835659840112 ) ) ;
#28852=CARTESIAN_POINT ( 'NONE',  ( 6.411709375437181002, 19.84076997167131751, -27.13309934696545511 ) ) ;
#28857=CARTESIAN_POINT ( 'NONE',  ( 10.71550314065649800, -18.98782435281344405, -23.79126320886110690 ) ) ;
#28862=CARTESIAN_POINT ( 'NONE',  ( -12.39972473649186568, 20.47873198151344454, -19.49820881543729101 ) ) ;
#28864=CARTESIAN_POINT ( 'NONE',  ( 12.88792179439757568, -23.58175436233876709, -14.50283011526977361 ) ) ;
#28870=CARTESIAN_POINT ( 'NONE',  ( -11.58530453518540959, 27.01100725576757355, -14.14221114289041381 ) ) ;
#28874=CARTESIAN_POINT ( 'NONE',  ( -29.93877630219436625, -6.466002002613472577, -13.99053332719549658 ) ) ;
#28876=ORIENTED_EDGE ( 'NONE', *, *, #20817, .F. ) ;
#28877=CARTESIAN_POINT ( 'NONE',  ( 28.23010493019885914, 0.2772093697871412799, -12.55662080966007110 ) ) ;
#28881=CARTESIAN_POINT ( 'NONE',  ( -30.36177892311615167, -0.01403434324402295062, -8.297102314141014290 ) ) ;
#28884=CARTESIAN_POINT ( 'NONE',  ( 28.41975474895474818, -1.822096834479148386, -14.26935881984800147 ) ) ;
#28885=CARTESIAN_POINT ( 'NONE',  ( 13.19262166295606775, 15.69476543507642852, -30.00000000000001066 ) ) ;
#28901=CARTESIAN_POINT ( 'NONE',  ( -22.67492542834196101, 9.789819215906979011, -8.893573617071718118 ) ) ;
#28902=CARTESIAN_POINT ( 'NONE',  ( 15.95756409205271709, -19.85041831507555798, -19.00748645968882045 ) ) ;
#28905=CARTESIAN_POINT ( 'NONE',  ( 15.31294454353861667, 26.87829293536686137, -6.413898871446972905 ) ) ;
#28907=CARTESIAN_POINT ( 'NONE',  ( -15.68734635201983174, 24.91775635742894579, -7.836637281011617162 ) ) ;
#28910=CARTESIAN_POINT ( 'NONE',  ( 13.79954197581136732, 23.33194756670403436, -14.47988002075514835 ) ) ;
#28912=CARTESIAN_POINT ( 'NONE',  ( 33.35910093694781864, -18.39580519663982727, -7.117606809128307788 ) ) ;
#28915=CARTESIAN_POINT ( 'NONE',  ( -12.45621400986809668, 21.34344825005930346, -18.40940681241713150 ) ) ;
#28917=CARTESIAN_POINT ( 'NONE',  ( -15.68502289456722210, -26.14630305052633119, -9.204429133117855599 ) ) ;
#28920=CARTESIAN_POINT ( 'NONE',  ( -35.14568626021495845, -14.53237387118475432, -5.000000000000003553 ) ) ;
#28921=CARTESIAN_POINT ( 'NONE',  ( -13.87797780512911139, -25.88099118681344990, -8.779743625905863880 ) ) ;
#28923=CARTESIAN_POINT ( 'NONE',  ( 16.86035064919571980, 22.16869397439054978, -5.950760093676068507 ) ) ;
#28925=CARTESIAN_POINT ( 'NONE',  ( 21.11582681380412296, 4.515134061867360771, -23.11302823821948849 ) ) ;
#28929=CARTESIAN_POINT ( 'NONE',  ( -26.68538983161234768, 0.004158945161739156619, -15.41724847776275098 ) ) ;
#28930=CARTESIAN_POINT ( 'NONE',  ( 31.42341880231480644, -0.5937245782808074912, -5.470706975624656465 ) ) ;
#28936=CARTESIAN_POINT ( 'NONE',  ( -20.90924525106831666, -8.502318254486386451, -30.00000000000000711 ) ) ;
#28947=CARTESIAN_POINT ( 'NONE',  ( 26.61403125366520683, -23.18509203170473043, -10.21710804142331419 ) ) ;
#28951=CARTESIAN_POINT ( 'NONE',  ( 10.47400997058416650, 17.78520939947398105, -28.04374864806230150 ) ) ;
#28954=CARTESIAN_POINT ( 'NONE',  ( -14.05926931476738595, 15.33240373186624694, -26.47723576656629163 ) ) ;
#28960=CARTESIAN_POINT ( 'NONE',  ( 13.00677425146152366, -23.09145112541884259, -15.45087358678626366 ) ) ;
#28962=CARTESIAN_POINT ( 'NONE',  ( 10.99973294177321215, 17.29901363094238675, -30.00000000000001421 ) ) ;
#28964=CARTESIAN_POINT ( 'NONE',  ( 15.36806905513557808, 26.68643454456307396, -6.416988418440872977 ) ) ;
#28966=CARTESIAN_POINT ( 'NONE',  ( -13.45748191022267193, 22.88503781989287944, -15.44276203698733774 ) ) ;
#28968=CARTESIAN_POINT ( 'NONE',  ( -15.20090094983863160, -26.38220823943847293, -7.828045879455097555 ) ) ;
#28971=CARTESIAN_POINT ( 'NONE',  ( -31.41171746008181032, -20.30212926178818833, -8.407145291683050914 ) ) ;
#28972=CARTESIAN_POINT ( 'NONE',  ( -1.907480624423063320, -21.18899373848512724, -23.32666558514067390 ) ) ;
#28973=CARTESIAN_POINT ( 'NONE',  ( 15.62450264098779051, 25.80212576317565265, -6.418156584292412425 ) ) ;
#28975=CARTESIAN_POINT ( 'NONE',  ( 23.08677377554354493, 8.111467817205479491, -11.84555345141176907 ) ) ;
#28977=CARTESIAN_POINT ( 'NONE',  ( -8.858816326124456353, -25.39986765292802318, -4.999999999999999112 ) ) ;
#28980=CARTESIAN_POINT ( 'NONE',  ( -32.87372159360177193, -3.395346227908654591, -8.163538743417984023 ) ) ;
#28987=CARTESIAN_POINT ( 'NONE',  ( 19.85478904061002581, -8.024875900502717485, -25.62134553024078087 ) ) ;
#28997=CARTESIAN_POINT ( 'NONE',  ( -1.032345509077061241, 20.89205812428711795, -26.96911111641401604 ) ) ;
#29004=CARTESIAN_POINT ( 'NONE',  ( 13.83290884757558104, 28.83794920898534642, -9.108879102860099053 ) ) ;
#29008=CARTESIAN_POINT ( 'NONE',  ( -19.65695430485491357, 15.61437265943404995, -6.449524717961147680 ) ) ;
#29012=CARTESIAN_POINT ( 'NONE',  ( 9.569772169525011307, -18.12929409070867948, -30.00000000000000000 ) ) ;
#29014=CARTESIAN_POINT ( 'NONE',  ( 12.10580092867515845, 19.95408366012758350, -20.53583464531860159 ) ) ;
#29015=CARTESIAN_POINT ( 'NONE',  ( -23.06249103411543544, 13.31513540672989926, -13.39439507595155554 ) ) ;
#29016=CARTESIAN_POINT ( 'NONE',  ( 19.48557158514988075, -11.24999999999998224, 6.000000000000000000 ) ) ;
#29020=CARTESIAN_POINT ( 'NONE',  ( -15.37464264532748004, -13.57371270378507866, -30.00000000000001421 ) ) ;
#29021=CARTESIAN_POINT ( 'NONE',  ( 6.428110747044506468, -21.25176611192976495, -20.99117257299570838 ) ) ;
#29022=CARTESIAN_POINT ( 'NONE',  ( 14.83059429241407123, 25.12647099005219786, -10.65921042686171560 ) ) ;
#29023=CARTESIAN_POINT ( 'NONE',  ( 18.24293951000086977, 12.18618061105114592, -20.11237983827145115 ) ) ;
#29027=CARTESIAN_POINT ( 'NONE',  ( -9.370244153187160308, 35.41390855819400940, -5.875078464094462660 ) ) ;
#29032=CARTESIAN_POINT ( 'NONE',  ( 30.76077710142195798, -0.06682749899988031650, -6.886782333292955194 ) ) ;
#29036=CARTESIAN_POINT ( 'NONE',  ( -30.24738832504583641, 0.1073154935118994652, -8.298770971096649518 ) ) ;
#29038=CARTESIAN_POINT ( 'NONE',  ( 21.21202041312366049, -5.034384574639595655, -24.45694360859277694 ) ) ;
#29048=FILL_AREA_STYLE ('',( #32306 ) ) ;
#29053=CARTESIAN_POINT ( 'NONE',  ( 13.86124000734726103, 15.40656454556149590, -27.04395577147614915 ) ) ;
#29055=CARTESIAN_POINT ( 'NONE',  ( 11.44944937545603203, 32.55932223515596036, -8.531584680290370315 ) ) ;
#29060=CARTESIAN_POINT ( 'NONE',  ( 15.31709984922062517, -25.22568667072951598, -11.53260946786015317 ) ) ;
#29064=CARTESIAN_POINT ( 'NONE',  ( -11.00242421671864790, 17.29730523913238827, -29.34874318703804263 ) ) ;
#29066=CARTESIAN_POINT ( 'NONE',  ( 14.30475062438041256, -25.71389175379151837, -9.717608377535148279 ) ) ;
#29070=CARTESIAN_POINT ( 'NONE',  ( -12.74940050238178735, 29.92346444574509334, -9.954757084635510012 ) ) ;
#29075=CARTESIAN_POINT ( 'NONE',  ( -20.45380339070934284, -5.041909576501859114, -26.41892961284724350 ) ) ;
#29078=CARTESIAN_POINT ( 'NONE',  ( 30.75747790117273794, 0.1077116562829361079, -5.474152632779671457 ) ) ;
#29082=ORIENTED_EDGE ( 'NONE', *, *, #5365, .T. ) ;
#29083=CARTESIAN_POINT ( 'NONE',  ( -20.96976484853918876, 0.8063829224527387929, -26.22476293720499285 ) ) ;
#29086=CARTESIAN_POINT ( 'NONE',  ( 20.45006009983584860, -1.583034825077791696, -30.00000000000000000 ) ) ;
#29088=CARTESIAN_POINT ( 'NONE',  ( 20.47044054185530726, -1.308743071981321560, -29.99999999999996803 ) ) ;
#29102=CARTESIAN_POINT ( 'NONE',  ( 25.71436706254310067, 9.015208126564360214, -5.000000000000000888 ) ) ;
#29104=CARTESIAN_POINT ( 'NONE',  ( -19.24333380943624050, 7.104126583969421205, -30.00000000000000000 ) ) ;
#29105=CARTESIAN_POINT ( 'NONE',  ( 14.07081834845426016, -16.54739306722566283, -24.54471350758723602 ) ) ;
#29109=CARTESIAN_POINT ( 'NONE',  ( 15.11738838694767217, 26.47243151418015827, -8.290468601944230187 ) ) ;
#29111=CARTESIAN_POINT ( 'NONE',  ( -15.56517687278530282, 24.67863418428501632, -8.782714596946386010 ) ) ;
#29115=CARTESIAN_POINT ( 'NONE',  ( 11.17396215358744271, 17.57883549974418713, -26.83496991786927666 ) ) ;
#29117=CARTESIAN_POINT ( 'NONE',  ( 25.46527745054863345, -14.04222176945395439, -16.62674829446373792 ) ) ;
#29120=CARTESIAN_POINT ( 'NONE',  ( -10.86820090079098122, 17.78895852278078848, -26.80626250025666835 ) ) ;
#29122=CARTESIAN_POINT ( 'NONE',  ( -16.05336419634168266, -26.67939413728697318, -7.338295715723472057 ) ) ;
#29125=CARTESIAN_POINT ( 'NONE',  ( -20.30067844349249029, -8.412790941247147103, -24.26813493527708232 ) ) ;
#29126=CARTESIAN_POINT ( 'NONE',  ( -14.83609535436326254, -26.57805634534657102, -5.474075349637312016 ) ) ;
#29128=CARTESIAN_POINT ( 'NONE',  ( 15.75967858163252977, 18.63110151714538887, -15.73365853743660736 ) ) ;
#29130=CARTESIAN_POINT ( 'NONE',  ( 23.44710309751157951, 3.753209576940052639, -17.73587880687377805 ) ) ;
#29134=CARTESIAN_POINT ( 'NONE',  ( -23.41064877084379248, 0.2929791562720443499, -20.50634540125940219 ) ) ;
#29136=CARTESIAN_POINT ( 'NONE',  ( 20.53937652207208231, 0.5506371726960779256, -28.69615207527581191 ) ) ;
#29144=CARTESIAN_POINT ( 'NONE',  ( -22.52744239175981278, -0.1803094636421871677, -20.90349153980994501 ) ) ;
#29156=CARTESIAN_POINT ( 'NONE',  ( 23.14904545314587025, -21.42671327224799427, -13.89312732397599426 ) ) ;
#29159=CARTESIAN_POINT ( 'NONE',  ( 12.05224603734456679, 20.93102218528974134, -19.42687687656769668 ) ) ;
#29163=CARTESIAN_POINT ( 'NONE',  ( -15.03102915852888444, 16.97105545825134953, -19.88194163820099192 ) ) ;
#29166=CARTESIAN_POINT ( 'NONE',  ( 11.82685544034319314, -21.49105343387592626, -18.46001624164255261 ) ) ;
#29168=DIRECTION ( 'NONE',  ( 1.000000000000000000, 0.000000000000000000, 0.000000000000000000 ) ) ;
#29169=CARTESIAN_POINT ( 'NONE',  ( 15.29903755497086415, 26.49996819934222358, -7.357928002827080149 ) ) ;
#29171=CARTESIAN_POINT ( 'NONE',  ( 11.47567478000847885, 18.44475041446002450, -23.85263498135895688 ) ) ;
#29175=CARTESIAN_POINT ( 'NONE',  ( -15.14009367329834888, 26.39762901518510319, -8.293352721384346538 ) ) ;
#29177=CARTESIAN_POINT ( 'NONE',  ( -11.53523938750379685, -20.97785456172497831, -19.49820750867069918 ) ) ;
#29179=CARTESIAN_POINT ( 'NONE',  ( -32.30830845181216660, -19.51484095444094535, -7.971085280149651453 ) ) ;
#29180=CARTESIAN_POINT ( 'NONE',  ( -1.806066488169840056, -20.67681132108909381, -26.61857900440850599 ) ) ;
#29181=CARTESIAN_POINT ( 'NONE',  ( 15.61778544462205431, 24.86146771946813061, -8.309072973913199434 ) ) ;
#29183=CARTESIAN_POINT ( 'NONE',  ( 23.00570941814261161, 9.122255987794249066, -9.381850414016666306 ) ) ;
#29188=CARTESIAN_POINT ( 'NONE',  ( -32.32461280127759551, -2.467648900451871796, -8.192925622072531056 ) ) ;
#29194=CARTESIAN_POINT ( 'NONE',  ( 18.76590878806661067, -8.252041909800054142, -29.21828954202150541 ) ) ;
#29200=CARTESIAN_POINT ( 'NONE',  ( -17.09304275257433048, 21.59026560281640883, -4.999999999999997335 ) ) ;
#29203=CARTESIAN_POINT ( 'NONE',  ( -1.015836423920226883, 20.57100803839839998, -28.44595161374707004 ) ) ;
#29209=CARTESIAN_POINT ( 'NONE',  ( 12.17552494184827339, 25.04416116006207460, -15.21251802476954396 ) ) ;
#29213=CARTESIAN_POINT ( 'NONE',  ( -19.90936391447298703, 14.41308808657887042, -9.387851554354570638 ) ) ;
#29216=CARTESIAN_POINT ( 'NONE',  ( 15.39191398672864430, -26.52213166449434922, -7.356080702479480316 ) ) ;
#29217=CARTESIAN_POINT ( 'NONE',  ( -75.15099915297791711, 43.38844959084113384, 3.000000000000000000 ) ) ;
#29218=CARTESIAN_POINT ( 'NONE',  ( 13.74447603680569330, 23.45254812458578897, -14.47033917909823053 ) ) ;
#29219=CARTESIAN_POINT ( 'NONE',  ( -6.023418944065157987, 39.81932404830322270, -4.999999999999988454 ) ) ;
#29222=CARTESIAN_POINT ( 'NONE',  ( -20.65774335103317227, -19.41944233773801898, -16.75787539182721275 ) ) ;
#29223=CARTESIAN_POINT ( 'NONE',  ( 5.978239409463006027, -20.40449185056595027, -24.25458186627032120 ) ) ;
#29224=CARTESIAN_POINT ( 'NONE',  ( 15.23844353641876381, 26.06950005415061966, -8.299311558484985696 ) ) ;
#29225=CARTESIAN_POINT ( 'NONE',  ( 21.09554553119179587, 13.00325820389446640, -4.999999999999996447 ) ) ;
#29229=CARTESIAN_POINT ( 'NONE',  ( -8.892437800321363994, 33.34416954038874792, -10.26036216454556538 ) ) ;
#29231=CARTESIAN_POINT ( 'NONE',  ( -9.590349012255924066, -18.48796701930649178, -26.83885042670429755 ) ) ;
#29234=CARTESIAN_POINT ( 'NONE',  ( 20.48156205581511458, 0.8692611811187744841, -30.00000000000000000 ) ) ;
#29238=CARTESIAN_POINT ( 'NONE',  ( -27.66913085872133493, 0.2817421747210221428, -13.51868300798002309 ) ) ;
#29242=CARTESIAN_POINT ( 'NONE',  ( 35.39442739984237818, -9.583334781271833691, -5.874798423248003942 ) ) ;
#29253=CARTESIAN_POINT ( 'NONE',  ( -12.11431921870781281, -16.53859995802357474, -30.00000000000001066 ) ) ;
#29257=CARTESIAN_POINT ( 'NONE',  ( 14.94108027486234391, 14.43501233363183722, -26.53384665043704871 ) ) ;
#29258=CARTESIAN_POINT ( 'NONE',  ( 7.125101744601430198, 22.13210201189419379, -22.13446490823594814 ) ) ;
#29262=CARTESIAN_POINT ( 'NONE',  ( 14.74936230926602754, -24.71673612477145099, -12.49531891550463136 ) ) ;
#29268=CARTESIAN_POINT ( 'NONE',  ( -11.90002364435815885, 19.37375396377245096, -21.61855169659785503 ) ) ;
#29271=CARTESIAN_POINT ( 'NONE',  ( 9.550906370826885095, -18.66785797286095772, -26.24677233048349123 ) ) ;
#29276=CARTESIAN_POINT ( 'NONE',  ( -13.31194575400795266, 31.44560903785412265, -4.999999999999996447 ) ) ;
#29279=CARTESIAN_POINT ( 'NONE',  ( -34.85992093908750178, -7.630325756601307852, -6.756134094771754306 ) ) ;
#29282=CARTESIAN_POINT ( 'NONE',  ( 29.41927195708630549, 0.2493808729530674062, -10.18512608144294873 ) ) ;
#29287=CARTESIAN_POINT ( 'NONE',  ( -30.49613795931812277, -0.02358107124917707340, -7.827247679823234883 ) ) ;
#29291=CARTESIAN_POINT ( 'NONE',  ( 21.47982430794170128, -1.719347241053234221, -24.74632320230637106 ) ) ;
#29292=CARTESIAN_POINT ( 'NONE',  ( 19.38974044528932339, 6.790579630597447292, -30.00000000000001066 ) ) ;
#29304=CARTESIAN_POINT ( 'NONE',  ( 5.194952508988293971, 31.55601946072578912, -13.85024353354532423 ) ) ;
#29307=CARTESIAN_POINT ( 'NONE',  ( -21.08026172065598303, 11.39671773059110471, -11.88141413567837645 ) ) ;
#29309=CARTESIAN_POINT ( 'NONE',  ( 20.01903129369064516, -26.18370256011770536, -9.488982841011081248 ) ) ;
#29313=CARTESIAN_POINT ( 'NONE',  ( 10.91553583107620007, 17.35227997941746025, -29.99999999999999289 ) ) ;
#29315=CARTESIAN_POINT ( 'NONE',  ( -15.68533655378858249, 25.84264350341399208, -5.000000000000000000 ) ) ;
#29318=CARTESIAN_POINT ( 'NONE',  ( 11.05794297925115721, 17.31467482071210995, -28.70911162413052509 ) ) ;
#29320=CARTESIAN_POINT ( 'NONE',  ( 32.95544229134011260, -19.49942389514326280, -6.696085395276597296 ) ) ;
#29322=ORIENTED_EDGE ( 'NONE', *, *, #32788, .F. ) ;
#29323=CARTESIAN_POINT ( 'NONE',  ( -11.73230135076743430, 19.55154583864819529, -21.58659322360452038 ) ) ;
#29325=CARTESIAN_POINT ( 'NONE',  ( -16.19425115350092170, -26.23270428128562060, -9.181978510543402194 ) ) ;
#29328=CARTESIAN_POINT ( 'NONE',  ( -21.86307784644980856, -9.053974127840067609, -21.89187085695087731 ) ) ;
#29329=CARTESIAN_POINT ( 'NONE',  ( -9.042611116926241976, -18.44506910216152207, -28.72510403185944838 ) ) ;
#29331=CARTESIAN_POINT ( 'NONE',  ( 13.62489508051746689, 16.45350914129836184, -24.13972925105511180 ) ) ;
#29333=CARTESIAN_POINT ( 'NONE',  ( 20.49112534608896752, 3.798362884196711420, -26.44148346684262307 ) ) ;
#29335=DIRECTION ( 'NONE',  ( -0.000000000000000000, -0.000000000000000000, 1.000000000000000000 ) ) ;
#29337=CARTESIAN_POINT ( 'NONE',  ( -20.48845606910846939, 0.6931994281368786259, -29.34533676971968319 ) ) ;
#29338=CARTESIAN_POINT ( 'NONE',  ( 31.31041380544943209, -0.5838616379220428199, -6.405593367610136646 ) ) ;
#29342=CARTESIAN_POINT ( 'NONE',  ( -20.39124144463984223, 2.214395427629727742, -30.00000000000000000 ) ) ;
#29343=CARTESIAN_POINT ( 'NONE',  ( 3.091399026088761826, 22.35909668862748489, -19.80438750953543803 ) ) ;
#29348=CARTESIAN_POINT ( 'NONE',  ( 40.48557158514985588, -11.25000000000009415, 0.000000000000000000 ) ) ;
#29352=CARTESIAN_POINT ( 'NONE',  ( 19.36144844918272057, -17.87459393394177098, -18.75074344801209136 ) ) ;
#29355=CARTESIAN_POINT ( 'NONE',  ( 14.99494866545234295, 27.15817369698893557, -7.803426522503517759 ) ) ;
#29358=CARTESIAN_POINT ( 'NONE',  ( -17.79487051664777653, 19.67746942737967686, -6.435833144689066643 ) ) ;
#29362=CARTESIAN_POINT ( 'NONE',  ( 15.31485424103991910, -26.62395559521617727, -6.417108935247511248 ) ) ;
#29364=CARTESIAN_POINT ( 'NONE',  ( 15.18411200369405911, 26.24943595222697112, -8.297974487407337563 ) ) ;
#29366=CARTESIAN_POINT ( 'NONE',  ( 10.98205083975412322, 17.31024513893945382, -29.34830281054965795 ) ) ;
#29368=CARTESIAN_POINT ( 'NONE',  ( -15.07734993948445634, 26.21826188937749080, -8.764079339540616687 ) ) ;
#29370=CARTESIAN_POINT ( 'NONE',  ( -9.514518717948533322, -18.20889895306638095, -28.70720734546157971 ) ) ;
#29373=CARTESIAN_POINT ( 'NONE',  ( -31.78402004932586422, -20.53790200070664795, -7.546523510580437133 ) ) ;
#29374=CARTESIAN_POINT ( 'NONE',  ( -9.284007248013184110, -25.41560839480977663, -5.953717583739019936 ) ) ;
#29375=CARTESIAN_POINT ( 'NONE',  ( 12.77005203192321936, 19.16553846908422187, -20.64983810823187582 ) ) ;
#29378=CARTESIAN_POINT ( 'NONE',  ( 22.82816708945120610, 8.056500230395544193, -12.84677774467560951 ) ) ;
#29384=CARTESIAN_POINT ( 'NONE',  ( -25.92394411639992313, -1.058492705183743610, -17.26204767525081962 ) ) ;
#29390=CARTESIAN_POINT ( 'NONE',  ( 20.60527582150886872, -9.801935859646480509, -23.00172017847723538 ) ) ;
#29396=DIRECTION ( 'NONE',  ( 0.000000000000000000, 0.000000000000000000, 1.000000000000000000 ) ) ;
#29401=CARTESIAN_POINT ( 'NONE',  ( -1.281162814042743125, 25.70428639643705893, -19.63338862114114391 ) ) ;
#29408=CARTESIAN_POINT ( 'NONE',  ( 13.02222589944813613, 25.99981456481483022, -13.33146986105651877 ) ) ;
#29411=CARTESIAN_POINT ( 'NONE',  ( -19.86079119093189860, 13.05667878886535505, -12.88684125302330585 ) ) ;
#29415=CARTESIAN_POINT ( 'NONE',  ( 10.86932238750741675, -19.98308206961400302, -21.61300728401371885 ) ) ;
#29417=CARTESIAN_POINT ( 'NONE',  ( 14.91649050592001657, 25.85859626688330337, -9.705674222665134465 ) ) ;
#29418=CARTESIAN_POINT ( 'NONE',  ( -11.31392148919591811, 36.91540483778867099, -5.000000000000009770 ) ) ;
#29420=DIRECTION ( 'NONE',  ( -0.000000000000000000, -0.000000000000000000, -1.000000000000000000 ) ) ;
#29422=CARTESIAN_POINT ( 'NONE',  ( -27.07092440652241550, -23.98996125867454765, -8.885765738235784639 ) ) ;
#29423=CARTESIAN_POINT ( 'NONE',  ( 4.352148934427582105, -20.44045777049943879, -25.42944795558441129 ) ) ;
#29424=CARTESIAN_POINT ( 'NONE',  ( 14.18108264993914247, 23.58463870654085426, -13.53032800031888705 ) ) ;
#29425=CARTESIAN_POINT ( 'NONE',  ( 17.10314071577965933, 11.30215440122589499, -29.99999999999999645 ) ) ;
#29428=CARTESIAN_POINT ( 'NONE',  ( -5.618023183903376960, 32.38114438848539578, -12.93671402627438027 ) ) ;
#29435=CARTESIAN_POINT ( 'NONE',  ( -22.71722914426532114, 0.6555868368756240239, -21.62299990059295496 ) ) ;
#29437=CARTESIAN_POINT ( 'NONE',  ( 21.79622464777374446, -5.878312547718441472, -23.18940552536372479 ) ) ;
#29452=CARTESIAN_POINT ( 'NONE',  ( 15.30396852670833496, 13.69301631135325792, -28.83852071831171671 ) ) ;
#29453=CARTESIAN_POINT ( 'NONE',  ( 8.334627820638896623, 28.79881821608029213, -14.89598926884550956 ) ) ;
#29458=CARTESIAN_POINT ( 'NONE',  ( 15.90316971415371050, -26.71736174511572059, -6.876908740700370615 ) ) ;
#29462=VERTEX_POINT ( 'NONE', #32049 ) ;
#29463=CARTESIAN_POINT ( 'NONE',  ( -15.01743222564557811, 25.97117291061142552, -9.238173852736359493 ) ) ;
#29466=CARTESIAN_POINT ( 'NONE',  ( 9.977387133527567897, -19.25012270239910350, -23.88382223299232265 ) ) ;
#29472=CARTESIAN_POINT ( 'NONE',  ( -10.02345167188216202, 25.24780830218480432, -16.99244641157628166 ) ) ;
#29476=EDGE_CURVE ( 'NONE', #39512, #2291, #32467, .T. ) ;
#29477=CARTESIAN_POINT ( 'NONE',  ( -30.78709934541342008, -6.653293242902037719, -13.05879633663284345 ) ) ;
#29480=CARTESIAN_POINT ( 'NONE',  ( 23.29810041234063078, 0.6049309071670201376, -20.54846396778402351 ) ) ;
#29484=UNCERTAINTY_MEASURE_WITH_UNIT (LENGTH_MEASURE( 1.000000000000000082E-05 ), #33951, 'distance_accuracy_value', 'NONE');
#29486=CARTESIAN_POINT ( 'NONE',  ( -25.86828471411721964, 0.3106744887170168612, -16.44263060901230133 ) ) ;
#29489=CARTESIAN_POINT ( 'NONE',  ( 20.53469380938287614, -0.9365662817021573883, -28.64349147984585287 ) ) ;
#29501=EDGE_LOOP ( 'NONE', ( #26630, #26495, #15038, #8538 ) ) ;
#29503=AXIS2_PLACEMENT_3D ( 'NONE', #13816, #5083, #38603 ) ;
#29504=CARTESIAN_POINT ( 'NONE',  ( 4.977190560089425730, 37.49800343037592398, -6.706298034499838856 ) ) ;
#29507=CARTESIAN_POINT ( 'NONE',  ( 21.86335951176813097, -26.92177804972322974, -6.781317475430051367 ) ) ;
#29514=CARTESIAN_POINT ( 'NONE',  ( 11.11465799936758536, 17.80655977757938757, -26.21732550182372989 ) ) ;
#29516=CARTESIAN_POINT ( 'NONE',  ( -15.52230086708900991, 25.98154550537155316, -6.889299160236542541 ) ) ;
#29520=CARTESIAN_POINT ( 'NONE',  ( 15.32298969794395305, 26.41742287619900864, -7.358219379429043805 ) ) ;
#29522=CARTESIAN_POINT ( 'NONE',  ( 26.02550586683312162, -15.40048236337812604, -15.67641675238316168 ) ) ;
#29524=CARTESIAN_POINT ( 'NONE',  ( -15.03361511047567944, 26.73982999355708401, -8.280263540186123095 ) ) ;
#29526=CARTESIAN_POINT ( 'NONE',  ( -12.43912898525198507, -20.85335003963435696, -19.38474122678572087 ) ) ;
#29529=CARTESIAN_POINT ( 'NONE',  ( -18.93673219582609946, -7.851978407254149417, -29.22088221090666593 ) ) ;
#29530=CARTESIAN_POINT ( 'NONE',  ( -11.20571940622763663, -21.02004376229801252, -19.53273776196371259 ) ) ;
#29532=CARTESIAN_POINT ( 'NONE',  ( 16.31817167508792110, 21.23338471077256173, -10.75037980594654385 ) ) ;
#29534=CARTESIAN_POINT ( 'NONE',  ( 20.38527744339932468, 3.800983730763423996, -27.02006532963664043 ) ) ;
#29535=DIRECTION ( 'NONE',  ( 0.000000000000000000, 0.000000000000000000, 1.000000000000000000 ) ) ;
#29538=CARTESIAN_POINT ( 'NONE',  ( -31.09037572277983230, -0.2342870890902537251, -5.472932512709705932 ) ) ;
#29540=CARTESIAN_POINT ( 'NONE',  ( 20.72199863514437013, 0.3644282351036394196, -27.41698609587929525 ) ) ;
#29543=CARTESIAN_POINT ( 'NONE',  ( -21.57036019902172441, 1.425437567633411673, -23.93286968654156155 ) ) ;
#29545=CARTESIAN_POINT ( 'NONE',  ( 9.163310636333564574, 20.63632441393291117, -29.99999999999999645 ) ) ;
#29550=CARTESIAN_POINT ( 'NONE',  ( 19.48557158514982746, -11.25000000000009415, -5.000000000000000000 ) ) ;
#29554=CARTESIAN_POINT ( 'NONE',  ( -21.61425450235728718, 5.849382257123279416, -19.97008806117738899 ) ) ;
#29556=CARTESIAN_POINT ( 'NONE',  ( -17.00000000000000000, 22.50000000000000355, 6.000000000000000000 ) ) ;
#29557=CARTESIAN_POINT ( 'NONE',  ( 22.37649770465107224, -19.47939514452113841, -15.75872631881709118 ) ) ;
#29560=CARTESIAN_POINT ( 'NONE',  ( 15.26389162175653880, 27.29890105065966921, -5.471704770948925933 ) ) ;
#29563=CARTESIAN_POINT ( 'NONE',  ( -13.91731628353523220, 15.09031314651060640, -28.80639967540201241 ) ) ;
#29565=CARTESIAN_POINT ( 'NONE',  ( 15.31712116136816348, -26.67315282756072747, -5.946102590047462222 ) ) ;
#29567=CARTESIAN_POINT ( 'NONE',  ( 11.90204051271606112, 19.37169779250840307, -21.61878633652037607 ) ) ;
#29571=CARTESIAN_POINT ( 'NONE',  ( -15.14941780581691511, 26.36647399290094285, -8.294559382431438976 ) ) ;
#29573=CARTESIAN_POINT ( 'NONE',  ( -14.57486702249206623, -25.45132688092154893, -10.65428866108198847 ) ) ;
#29577=CARTESIAN_POINT ( 'NONE',  ( -23.44121009936221611, -15.14254397387390405, -17.60241826803686394 ) ) ;
#29578=CARTESIAN_POINT ( 'NONE',  ( -8.902953248278356213, -24.69963661859840087, -10.29415431459782226 ) ) ;
#29579=CARTESIAN_POINT ( 'NONE',  ( 15.71024529842017436, 24.58213290089141978, -8.311554404203290503 ) ) ;
#29581=CARTESIAN_POINT ( 'NONE',  ( 21.76977311220710121, 8.780111591737426835, -14.89262190181197809 ) ) ;
#29585=VERTEX_POINT ( 'NONE', #4824 ) ;
#29586=CARTESIAN_POINT ( 'NONE',  ( -32.95954470968036532, -2.553576478305152886, -5.461075913141677951 ) ) ;
#29591=CARTESIAN_POINT ( 'NONE',  ( 34.19331540110757572, -17.52795661523900961, -5.856166949180161119 ) ) ;
#29597=VECTOR ( 'NONE', #4590, 1000.000000000000000 ) ;
#29601=CARTESIAN_POINT ( 'NONE',  ( 0.3612209001919436946, 33.46140997383869120, -12.88978858418767715 ) ) ;
#29609=CARTESIAN_POINT ( 'NONE',  ( 13.99338577196167321, 26.32572741696355934, -11.50149747935983413 ) ) ;
#29612=CARTESIAN_POINT ( 'NONE',  ( -17.97661971344022902, 11.67401855304127523, -22.24591093701263134 ) ) ;
#29615=CARTESIAN_POINT ( 'NONE',  ( 15.35992194021738300, -26.51421217328086755, -7.356954887253082553 ) ) ;
#29617=CARTESIAN_POINT ( 'NONE',  ( 12.36626470332232763, 20.52366543882663663, -19.49109148384244605 ) ) ;
#29618=CARTESIAN_POINT ( 'NONE',  ( 16.84920187454417828, 29.09530251867925443, -13.79123840944734880 ) ) ;
#29621=CARTESIAN_POINT ( 'NONE',  ( -24.25258108503407328, -22.82957551827030684, -12.05318650362971766 ) ) ;
#29622=CARTESIAN_POINT ( 'NONE',  ( 2.847707569172010622, -20.70244955242776896, -25.48826837884827512 ) ) ;
#29623=CARTESIAN_POINT ( 'NONE',  ( 13.37878228885757181, 21.93571083929289500, -16.47005970201684377 ) ) ;
#29624=CARTESIAN_POINT ( 'NONE',  ( 16.68830378044837914, 11.92867436094057787, -29.42711812811024430 ) ) ;
#29625=DIRECTION ( 'NONE',  ( 0.000000000000000000, 0.000000000000000000, 1.000000000000000000 ) ) ;
#29628=CARTESIAN_POINT ( 'NONE',  ( -7.439527340440343472, 36.65827423083189274, -5.866875955026374712 ) ) ;
#29637=CARTESIAN_POINT ( 'NONE',  ( -29.98443152904168940, 0.2276001790674742065, -8.770443406083204607 ) ) ;
#29639=CARTESIAN_POINT ( 'NONE',  ( 19.80298806677364709, -5.334938486795024026, -29.24553249901355656 ) ) ;
#29641=PRODUCT_CONTEXT ( 'NONE', #3361, 'mechanical' ) ;
#29655=CARTESIAN_POINT ( 'NONE',  ( 19.01290250727002018, 16.88526884184630461, -6.928959836932907734 ) ) ;
#29657=CARTESIAN_POINT ( 'NONE',  ( 5.802993469575763896, 20.02905561438103987, -27.10461695544125504 ) ) ;
#29662=CARTESIAN_POINT ( 'NONE',  ( 9.870890762638957483, -18.12032902427516490, -28.06054875518065828 ) ) ;
#29663=CARTESIAN_POINT ( 'NONE',  ( 26.31271763591405133, -28.25584584496056806, -4.999999999999992895 ) ) ;
#29664=AXIS2_PLACEMENT_3D ( 'NONE', #36302, #20463, #8464 ) ;
#29667=CARTESIAN_POINT ( 'NONE',  ( -14.92970566726980053, 25.81632110502188127, -9.708005003289713386 ) ) ;
#29669=CARTESIAN_POINT ( 'NONE',  ( 10.40875948710034393, -20.60785335237228821, -20.62936224035580679 ) ) ;
#29675=CARTESIAN_POINT ( 'NONE',  ( -10.97358061145035890, 27.71178282933573556, -14.08931735373363736 ) ) ;
#29678=CARTESIAN_POINT ( 'NONE',  ( -27.80923940722906096, -4.326673682006865640, -16.00039589016309804 ) ) ;
#29681=CARTESIAN_POINT ( 'NONE',  ( 27.10756907707635222, 0.2822830175333150837, -14.47971340185655720 ) ) ;
#29686=CARTESIAN_POINT ( 'NONE',  ( -22.73079022145749661, 0.6103013872901770220, -21.61737968283550515 ) ) ;
#29689=CARTESIAN_POINT ( 'NONE',  ( 31.04069800111786037, -4.622072988384480219, -12.21417130457122369 ) ) ;
#29704=CARTESIAN_POINT ( 'NONE',  ( 6.020667366826272904, 36.76097728554005073, -7.565657333014108588 ) ) ;
#29707=CARTESIAN_POINT ( 'NONE',  ( 14.98275746386106633, -20.98974146216496806, -18.11133193274115172 ) ) ;
#29713=CARTESIAN_POINT ( 'NONE',  ( 14.49168446761245121, 25.08686542864395719, -11.59031123052781176 ) ) ;
#29714=CIRCLE ( 'NONE', #21281, 18.00000000000000000 ) ;
#29716=CARTESIAN_POINT ( 'NONE',  ( -12.17635432242331639, 19.07997197433500958, -21.66576389041598816 ) ) ;
#29720=CARTESIAN_POINT ( 'NONE',  ( 13.25152841075581023, 22.16086677354865841, -16.45058133833084568 ) ) ;
#29722=CARTESIAN_POINT ( 'NONE',  ( 20.46135049998398969, -12.10462214192124897, -21.83542778586768307 ) ) ;
#29725=CARTESIAN_POINT ( 'NONE',  ( -11.10899655815487286, 18.75408899665464091, -23.79491269033197298 ) ) ;
#29727=CARTESIAN_POINT ( 'NONE',  ( -16.30272796611154362, -25.72258041950212970, -10.55552886378998068 ) ) ;
#29731=CARTESIAN_POINT ( 'NONE',  ( -19.39494709936099781, -7.365632527046459543, -27.74002402222404484 ) ) ;
#29732=CARTESIAN_POINT ( 'NONE',  ( -13.16152623113992348, -24.05409641368920504, -13.53816783273080127 ) ) ;
#29734=CARTESIAN_POINT ( 'NONE',  ( 14.38663302965268542, 17.85124432971809583, -19.80540727126786393 ) ) ;
#29736=CARTESIAN_POINT ( 'NONE',  ( 23.72444218837145158, 2.197028041356958727, -18.63410458577873285 ) ) ;
#29740=CARTESIAN_POINT ( 'NONE',  ( -30.90771625177988113, -0.2200328037497713274, -6.882354936934209633 ) ) ;
#29741=CARTESIAN_POINT ( 'NONE',  ( 25.48014744351514693, -0.1196400326508215983, -17.37346584602176591 ) ) ;
#29744=CARTESIAN_POINT ( 'NONE',  ( -29.21107446086027082, 1.733986180571661873, -5.474071973575725281 ) ) ;
#29745=CARTESIAN_POINT ( 'NONE',  ( -18.07620401364299667, 24.68088026512193522, -5.000000000000000000 ) ) ;
#29752=CIRCLE ( 'NONE', #16765, 18.00000000000002842 ) ;
#29759=CARTESIAN_POINT ( 'NONE',  ( -23.53550312530761346, 5.153870508594805777, -15.77917154867632732 ) ) ;
#29760=CARTESIAN_POINT ( 'NONE',  ( 12.05833259093393117, 18.99598562053712314, -30.00000000000000000 ) ) ;
#29762=CARTESIAN_POINT ( 'NONE',  ( 23.61345955422964948, -23.17554374091795566, -12.06964299242005545 ) ) ;
#29765=CARTESIAN_POINT ( 'NONE',  ( 14.61867237244439721, 25.74613599029391153, -10.63056160451222532 ) ) ;
#29767=CARTESIAN_POINT ( 'NONE',  ( -16.59571780117528306, 22.97185772529794434, -4.999999999999999112 ) ) ;
#29769=CARTESIAN_POINT ( 'NONE',  ( 9.534133013345522656, -18.29165158992863738, -28.07943093716786720 ) ) ;
#29771=CARTESIAN_POINT ( 'NONE',  ( 15.37593855497895134, 26.65856383457258261, -6.417017949581364178 ) ) ;
#29775=CARTESIAN_POINT ( 'NONE',  ( -13.97834737394524396, 24.06032382748300691, -13.50144991984861775 ) ) ;
#29778=CARTESIAN_POINT ( 'NONE',  ( -9.487969581998370927, -18.17220041443854583, -30.00000000000000000 ) ) ;
#29782=CARTESIAN_POINT ( 'NONE',  ( -18.00895331265001076, -11.61959776305488923, -25.58275405777271416 ) ) ;
#29783=CARTESIAN_POINT ( 'NONE',  ( -6.481551405175245861, -23.88552407126505628, -12.80164040886976196 ) ) ;
#29784=CARTESIAN_POINT ( 'NONE',  ( 11.55093992908412126, 16.93669310835906572, -30.00000000000000000 ) ) ;
#29786=CARTESIAN_POINT ( 'NONE',  ( 25.30102210956597020, 6.478166462252010760, -5.958356417954576933 ) ) ;
#29791=ORIENTED_EDGE ( 'NONE', *, *, #27152, .T. ) ;
#29792=CARTESIAN_POINT ( 'NONE',  ( -20.48034806427134313, -1.125288817275917008, -30.00000000000000000 ) ) ;
#29797=DIRECTION ( 'NONE',  ( -0.000000000000000000, -0.000000000000000000, -1.000000000000000000 ) ) ;
#29804=CARTESIAN_POINT ( 'NONE',  ( 1.384233241701591899, 33.43667168175883830, -12.89082250209952640 ) ) ;
#29811=CARTESIAN_POINT ( 'NONE',  ( 11.40974394891913057, 20.73802190120719047, -20.40291310562222193 ) ) ;
#29814=CARTESIAN_POINT ( 'NONE',  ( -18.71293717657318112, 16.10063966046890727, -10.85465713401838705 ) ) ;
#29817=CARTESIAN_POINT ( 'NONE',  ( 10.00012431106257083, -18.80013087926857196, -25.01062988768326179 ) ) ;
#29819=CARTESIAN_POINT ( 'NONE',  ( 10.97849594700618425, 17.36583575188205941, -28.70580706648543412 ) ) ;
#29822=CARTESIAN_POINT ( 'NONE',  ( -26.85786336487645798, -23.80939247740336029, -9.326638227506361289 ) ) ;
#29823=CARTESIAN_POINT ( 'NONE',  ( 1.811844033679846255, -24.72003103208043839, -6.454257893813014846 ) ) ;
#29824=CARTESIAN_POINT ( 'NONE',  ( 12.05618289028952894, 19.20794177042097317, -21.64528753798118998 ) ) ;
#29825=CARTESIAN_POINT ( 'NONE',  ( 17.23802802930360301, 12.42931764800617422, -23.31302680604725808 ) ) ;
#29829=CARTESIAN_POINT ( 'NONE',  ( -6.749652402378329086, 32.93967545494245286, -12.03137183237044994 ) ) ;
#29838=CARTESIAN_POINT ( 'NONE',  ( -30.27639200216978921, 0.2080803662807323429, -7.829370471578710244 ) ) ;
#29840=CARTESIAN_POINT ( 'NONE',  ( 34.53444588180299490, -11.54643433007243658, -8.446032751583265608 ) ) ;
#29842=SHAPE_DEFINITION_REPRESENTATION ( #22001, #8618 ) ;
#29850=CARTESIAN_POINT ( 'NONE',  ( -15.51137734265978452, -13.41919184397205989, -30.00000000000002842 ) ) ;
#29854=CARTESIAN_POINT ( 'NONE',  ( 15.03591831393239353, 14.57499296974832781, -25.40006105580101092 ) ) ;
#29855=CARTESIAN_POINT ( 'NONE',  ( 11.29805954857153516, 32.07545058919369296, -9.425914070865543337 ) ) ;
#29856=ORIENTED_EDGE ( 'NONE', *, *, #8762, .F. ) ;
#29859=CARTESIAN_POINT ( 'NONE',  ( 15.74830575105852226, -26.80738400109229147, -5.000000000000000888 ) ) ;
#29863=CARTESIAN_POINT ( 'NONE',  ( -11.47017161796830820, 18.44952784731361461, -23.85172870555624769 ) ) ;
#29865=CARTESIAN_POINT ( 'NONE',  ( 12.69460418788277778, -24.00195335915195471, -13.55933954820171117 ) ) ;
#29870=CARTESIAN_POINT ( 'NONE',  ( -11.48376733107994063, 31.82382468019164534, -9.435985624090092116 ) ) ;
#29874=CARTESIAN_POINT ( 'NONE',  ( -33.14594191503550036, -6.195422458497144014, -9.876726191397294130 ) ) ;
#29877=CARTESIAN_POINT ( 'NONE',  ( 28.83991352859764845, 0.1616784926268942935, -11.60121644625366777 ) ) ;
#29885=CARTESIAN_POINT ( 'NONE',  ( -30.89051437471967887, -0.02824647624105855806, -5.474200716472483741 ) ) ;
#29888=CARTESIAN_POINT ( 'NONE',  ( 25.96735800389505400, -3.809743913480001964, -17.99300411472922079 ) ) ;
#29903=CARTESIAN_POINT ( 'NONE',  ( 6.972704631243735740, 35.83133064181360794, -8.442364626267595540 ) ) ;
#29908=CARTESIAN_POINT ( 'NONE',  ( 18.97005494646916901, -26.22064284678461021, -9.527288771957310942 ) ) ;
#29913=CARTESIAN_POINT ( 'NONE',  ( 11.41474510619553584, 18.49724849801811288, -23.84291374344302028 ) ) ;
#29915=CARTESIAN_POINT ( 'NONE',  ( -11.74180227034369395, 17.69492043334604503, -25.07106241003591407 ) ) ;
#29918=CARTESIAN_POINT ( 'NONE',  ( 13.27975059410090886, 22.11080264522603755, -16.45492753240296580 ) ) ;
#29920=CARTESIAN_POINT ( 'NONE',  ( 24.57022902387958041, -15.56970263708699420, -16.62770197561091479 ) ) ;
#29922=CARTESIAN_POINT ( 'NONE',  ( -14.87717852953102415, 26.83350838914018155, -8.737445087221045625 ) ) ;
#29924=CARTESIAN_POINT ( 'NONE',  ( -17.98522147080449329, -26.74354288057798357, -8.201969047480554664 ) ) ;
#29926=CARTESIAN_POINT ( 'NONE',  ( 17.34253826607186255, 27.32041144404028543, -5.000000000000000000 ) ) ;
#29928=CARTESIAN_POINT ( 'NONE',  ( -35.44912448985124342, -12.22065591061644518, -5.865871141610608852 ) ) ;
#29929=CARTESIAN_POINT ( 'NONE',  ( -10.76246318078418440, -20.54449477115332812, -20.58967632249421342 ) ) ;
#29932=CARTESIAN_POINT ( 'NONE',  ( 29.62645323178156076, 1.115095990645281532, -6.891287580428307358 ) ) ;
#29936=CARTESIAN_POINT ( 'NONE',  ( -20.53086226280845139, 0.7723353936895273053, -28.70396588008199856 ) ) ;
#29937=CARTESIAN_POINT ( 'NONE',  ( 31.77445454197319563, -1.004264897904582954, -5.000000000000000000 ) ) ;
#29942=CARTESIAN_POINT ( 'NONE',  ( -28.10180234942462718, 1.777709783175517977, -10.22205278907307502 ) ) ;
#29943=CARTESIAN_POINT ( 'NONE',  ( -11.31392148919591811, 36.91540483778867099, -14.26382729546508088 ) ) ;
#29953=CARTESIAN_POINT ( 'NONE',  ( -20.02047420364571906, 5.006101022618450358, -27.65113345958681634 ) ) ;
#29956=CARTESIAN_POINT ( 'NONE',  ( 16.65204975395604237, -15.35049418271700006, -23.13297094094993511 ) ) ;
#29959=CARTESIAN_POINT ( 'NONE',  ( 10.75708226969095627, 17.60808951942069456, -28.06054662593295390 ) ) ;
#29963=CARTESIAN_POINT ( 'NONE',  ( -14.32137131676681463, 17.27576680070661297, -20.87916438781902073 ) ) ;
#29966=CARTESIAN_POINT ( 'NONE',  ( 15.42861054628522233, 26.73803055450190058, -5.474192869590372545 ) ) ;
#29967=EDGE_LOOP ( 'NONE', ( #16251, #15123, #32658, #4534, #34525, #16450 ) ) ;
#29970=CARTESIAN_POINT ( 'NONE',  ( -14.87240269245140567, 25.99712635132547689, -9.698082481812916100 ) ) ;
#29972=CARTESIAN_POINT ( 'NONE',  ( -10.84979689475692766, -19.98760476204195058, -21.61563630248454615 ) ) ;
#29975=CARTESIAN_POINT ( 'NONE',  ( -27.33604612326909233, -15.39033642126372037, -14.72902412931908067 ) ) ;
#29976=CARTESIAN_POINT ( 'NONE',  ( -9.295420884976664411, -25.43675055676933638, -5.476495350188955946 ) ) ;
#29978=CARTESIAN_POINT ( 'NONE',  ( 11.99148969583736246, 17.49118954514694124, -25.10245485184838898 ) ) ;
#29981=CARTESIAN_POINT ( 'NONE',  ( 22.20949710084497397, 6.145177408896746130, -17.88822456531065441 ) ) ;
#29987=ORIENTED_EDGE ( 'NONE', *, *, #32271, .F. ) ;
#29988=CARTESIAN_POINT ( 'NONE',  ( -28.54615080091948087, -0.9312913580789032864, -13.39927911465294841 ) ) ;
#29989=CARTESIAN_POINT ( 'NONE',  ( 24.58697627075426695, 0.3755645577039563032, -18.44458219269206722 ) ) ;
#30005=CARTESIAN_POINT ( 'NONE',  ( 0.4029506027351301145, 37.46258620939589434, -8.404766914894960195 ) ) ;
#30013=CARTESIAN_POINT ( 'NONE',  ( 14.58186407764969061, 28.53296701108370925, -7.305968526827398613 ) ) ;
#30017=CARTESIAN_POINT ( 'NONE',  ( -19.19098252355692580, 16.63498700241322936, -5.962789986923132446 ) ) ;
#30020=CARTESIAN_POINT ( 'NONE',  ( 14.65398229857985157, -25.46724026263229135, -10.65132889757489032 ) ) ;
#30023=CARTESIAN_POINT ( 'NONE',  ( 12.91822118044063394, 21.66998749496536902, -17.43529018280291254 ) ) ;
#30024=CARTESIAN_POINT ( 'NONE',  ( 3.091399026088761826, 22.35909668862748489, -30.00000000000000711 ) ) ;
#30027=CARTESIAN_POINT ( 'NONE',  ( -26.78191558544384776, -21.01471732344365151, -12.00199842359465130 ) ) ;
#30029=CARTESIAN_POINT ( 'NONE',  ( 1.745246714805118726, -24.23261900456495965, -10.38794052831897829 ) ) ;
#30030=CARTESIAN_POINT ( 'NONE',  ( 15.21143254768586495, 25.78252244675921290, -8.771152263473718236 ) ) ;
#30032=CARTESIAN_POINT ( 'NONE',  ( 21.25194171196830339, 11.83548972908152841, -9.890527645891060260 ) ) ;
#30034=ORIENTED_EDGE ( 'NONE', *, *, #2619, .T. ) ;
#30035=CARTESIAN_POINT ( 'NONE',  ( -7.357442437755574716, 36.13703667136246622, -7.577783863828958744 ) ) ;
#30044=CARTESIAN_POINT ( 'NONE',  ( -20.47417334391911936, 1.028570030172704763, -29.35142929161455072 ) ) ;
#30046=CARTESIAN_POINT ( 'NONE',  ( 20.19203522719319466, -6.104531446830016250, -26.36559112601934984 ) ) ;
#30057=DIRECTION ( 'NONE',  ( -0.000000000000000000, -0.000000000000000000, -1.000000000000000000 ) ) ;
#30061=CARTESIAN_POINT ( 'NONE',  ( 18.97955609020411316, 16.84654830053328567, -7.414115074451304466 ) ) ;
#30062=CARTESIAN_POINT ( 'NONE',  ( 11.98184379570800218, 31.25359194820647701, -9.457391703318352327 ) ) ;
#30064=CARTESIAN_POINT ( 'NONE',  ( -22.38085876145960640, 10.82216326969894737, -5.482735768144592292 ) ) ;
#30069=CARTESIAN_POINT ( 'NONE',  ( 13.06227854178500181, -22.56613844598916430, -16.39924439641581699 ) ) ;
#30072=CARTESIAN_POINT ( 'NONE',  ( -14.84019340197460934, 25.60882683859346187, -10.18024224215897178 ) ) ;
#30074=CARTESIAN_POINT ( 'NONE',  ( 8.893966021365395491, -18.47319264949478779, -29.36029315992060873 ) ) ;
#30078=CARTESIAN_POINT ( 'NONE',  ( -7.473191970175785848, 20.37911561391303650, -24.56105570974891705 ) ) ;
#30082=LINE ( 'NONE', #5098, #11799 ) ;
#30084=CARTESIAN_POINT ( 'NONE',  ( 30.12592084412306548, 0.07472801878552456922, -8.768476169707916767 ) ) ;
#30089=CARTESIAN_POINT ( 'NONE',  ( -23.92885585469906573, 0.5139776474599682121, -19.49970526494919554 ) ) ;
#30092=CARTESIAN_POINT ( 'NONE',  ( 20.78038650074347160, -2.939622687103573551, -26.54821385022073343 ) ) ;
#30107=CARTESIAN_POINT ( 'NONE',  ( 5.670256885233474264, 29.09287741234969715, -15.76086933226568476 ) ) ;
#30113=CARTESIAN_POINT ( 'NONE',  ( 16.95921849111858748, -23.60331070195671188, -14.18631301038341697 ) ) ;
#30118=CARTESIAN_POINT ( 'NONE',  ( 14.88782195473658909, 25.94899730737486720, -9.700714136109681363 ) ) ;
#30121=CARTESIAN_POINT ( 'NONE',  ( -15.04061483196161753, 25.01295785739290167, -10.19153934133739270 ) ) ;
#30124=CARTESIAN_POINT ( 'NONE',  ( 12.98912340479801131, 21.55496206960689420, -17.44778214844380315 ) ) ;
#30126=CARTESIAN_POINT ( 'NONE',  ( 17.65215317207318080, -10.44170805849464401, -29.21171622812354585 ) ) ;
#30128=CARTESIAN_POINT ( 'NONE',  ( -12.68926805779758027, 22.04200062495521095, -17.38483120121016157 ) ) ;
#30130=CARTESIAN_POINT ( 'NONE',  ( -17.61165795415892532, -26.24323257045744029, -9.577737097562327051 ) ) ;
#30131=CARTESIAN_POINT ( 'NONE',  ( -6.023418944065157987, 39.81932404830322270, -4.999999999999988454 ) ) ;
#30134=CARTESIAN_POINT ( 'NONE',  ( -24.86735191267609224, -9.411377462502228397, -18.68429284230914078 ) ) ;
#30135=CARTESIAN_POINT ( 'NONE',  ( -15.13531929286638977, -26.65245416579944759, -5.474118494994447026 ) ) ;
#30138=CARTESIAN_POINT ( 'NONE',  ( 28.62947963101195725, 2.007663261502573793, -7.844485846290086606 ) ) ;
#30144=CARTESIAN_POINT ( 'NONE',  ( -22.75019642290121880, 0.5465434661334764854, -21.60863951403461414 ) ) ;
#30146=CARTESIAN_POINT ( 'NONE',  ( 30.60780290727160136, -0.8964730165270395901, -9.647732689552546148 ) ) ;
#30148=ORIENTED_EDGE ( 'NONE', *, *, #16239, .T. ) ;
#30149=CARTESIAN_POINT ( 'NONE',  ( -27.66981915501925826, 3.518264008085504990, -5.000000000000000888 ) ) ;
#30161=CARTESIAN_POINT ( 'NONE',  ( -23.05888776652749428, 5.977869874196464650, -15.81723421387264139 ) ) ;
#30164=CARTESIAN_POINT ( 'NONE',  ( 25.90091635383566526, -25.33841663918061116, -7.598904778598901899 ) ) ;
#30167=CARTESIAN_POINT ( 'NONE',  ( 10.84377413474652307, 17.80538317806753668, -26.80397311259553206 ) ) ;
#30170=CARTESIAN_POINT ( 'NONE',  ( -13.37529537539570867, 15.55228444284129097, -30.00000000000000711 ) ) ;
#30173=CARTESIAN_POINT ( 'NONE',  ( 11.02706334812793720, 17.33462162532257977, -28.70783002534086847 ) ) ;
#30177=CARTESIAN_POINT ( 'NONE',  ( -15.05848678793640971, 26.27994695046478313, -8.761354843867154685 ) ) ;
#30180=CARTESIAN_POINT ( 'NONE',  ( -15.06065773102657523, -26.00907756546740401, -9.234374514430680136 ) ) ;
#30183=CARTESIAN_POINT ( 'NONE',  ( -32.17239265530350423, -18.11259179091877414, -9.280970269152343022 ) ) ;
#30184=CARTESIAN_POINT ( 'NONE',  ( -11.56078958348037844, -25.79303082475217224, -5.948641159686665070 ) ) ;
#30185=CYLINDRICAL_SURFACE ( 'NONE', #9884, 21.00000000000002842 ) ;
#30186=CARTESIAN_POINT ( 'NONE',  ( 11.83150832767071314, 16.74097710667822270, -29.36572269274261870 ) ) ;
#30187=VERTEX_POINT ( 'NONE', #13102 ) ;
#30188=CARTESIAN_POINT ( 'NONE',  ( 24.47864856487766261, 6.389536464586502262, -10.82169681586935539 ) ) ;
#30189=CARTESIAN_POINT ( 'NONE',  ( 17.87719828188526705, -27.21529464712563495, -5.000000000000000000 ) ) ;
#30195=CARTESIAN_POINT ( 'NONE',  ( -31.53032910951097989, -1.198340018515870575, -7.780284805138951043 ) ) ;
#30196=CARTESIAN_POINT ( 'NONE',  ( 30.33251295709586159, -0.1458810018284433796, -8.758614351443290147 ) ) ;
#30208=CARTESIAN_POINT ( 'NONE',  ( 0.4067949480120627848, 37.90417743010413432, -7.544532716226419744 ) ) ;
#30217=CARTESIAN_POINT ( 'NONE',  ( 10.07128235380245052, 18.51023362060226063, -26.10639040881114781 ) ) ;
#30222=CARTESIAN_POINT ( 'NONE',  ( -18.38750743028887769, 15.73877471124131233, -12.84865677469772649 ) ) ;
#30226=CARTESIAN_POINT ( 'NONE',  ( 9.590584324842760466, -18.26333419585273887, -28.07628972030180492 ) ) ;
#30227=CARTESIAN_POINT ( 'NONE',  ( 15.17329373222786337, 26.28549969035456613, -8.297710605404065021 ) ) ;
#30228=CARTESIAN_POINT ( 'NONE',  ( 11.09996104015035279, 17.63036184699812381, -26.82805355210400933 ) ) ;
#30232=CARTESIAN_POINT ( 'NONE',  ( -22.87698515175695846, -19.07680134495290503, -15.74116178021451518 ) ) ;
#30233=CARTESIAN_POINT ( 'NONE',  ( 3.101033983210284450, -21.57712604886545193, -21.14822272720248009 ) ) ;
#30234=CARTESIAN_POINT ( 'NONE',  ( 15.44951243528052487, 25.68331376365496865, -7.831890575027415480 ) ) ;
#30235=CARTESIAN_POINT ( 'NONE',  ( 21.49425838908486952, 11.96617313177288011, -7.918919338291130927 ) ) ;
#30237=CARTESIAN_POINT ( 'NONE',  ( -7.446792957322618811, 36.70800515527383823, -5.439754417765567673 ) ) ;
#30246=CARTESIAN_POINT ( 'NONE',  ( -30.68739395818431959, 0.1797671858537337741, -5.474131994021600889 ) ) ;
#30247=CARTESIAN_POINT ( 'NONE',  ( 32.68782978559330843, -10.89902263858124876, -11.12137701297516479 ) ) ;
#30252=DIRECTION ( 'NONE',  ( 0.000000000000000000, 0.000000000000000000, -1.000000000000000000 ) ) ;
#30262=CARTESIAN_POINT ( 'NONE',  ( 0.000000000000000000, 22.50000000000000355, 6.000000000000000000 ) ) ;
#30264=CARTESIAN_POINT ( 'NONE',  ( 20.56955126053106042, -16.81405870680252690, -18.68695065117257315 ) ) ;
#30265=CARTESIAN_POINT ( 'NONE',  ( 18.34675927358811975, 14.71332062100892202, -14.88700802970827120 ) ) ;
#30266=CARTESIAN_POINT ( 'NONE',  ( 12.25923078083974360, 32.08250591462850565, -7.667896807040970764 ) ) ;
#30269=CARTESIAN_POINT ( 'NONE',  ( -18.36874938498262466, 9.174293865845140061, -28.86133430165910951 ) ) ;
#30272=CARTESIAN_POINT ( 'NONE',  ( 14.51603474985190623, -24.68602004783254245, -12.51313738316805768 ) ) ;
#30275=CARTESIAN_POINT ( 'NONE',  ( -11.16442365856205932, 17.77074711030141785, -26.22272145734717697 ) ) ;
#30276=VECTOR ( 'NONE', #39713, 1000.000000000000000 ) ;
#30277=CARTESIAN_POINT ( 'NONE',  ( -15.88203534348982693, -18.94643611089546198, -19.99739510857416036 ) ) ;
#30278=CARTESIAN_POINT ( 'NONE',  ( 9.207210607180677187, -19.50632804910366858, -23.97127578096531053 ) ) ;
#30279=AXIS2_PLACEMENT_3D ( 'NONE', #24626, #36627, #12038 ) ;
#30283=CARTESIAN_POINT ( 'NONE',  ( -12.49268588895353105, 31.85193245464213518, -7.673184180311376501 ) ) ;
#30290=CARTESIAN_POINT ( 'NONE',  ( 27.68069398113840052, 0.2662808206736965722, -13.51781012861318843 ) ) ;
#30294=CARTESIAN_POINT ( 'NONE',  ( -30.59254050256992841, 0.006261417149339938010, -7.357959963668824876 ) ) ;
#30297=CARTESIAN_POINT ( 'NONE',  ( 20.48544130033148747, -2.888783638426572598, -27.89533876242412447 ) ) ;
#30307=EDGE_LOOP ( 'NONE', ( #12064, #26380 ) ) ;
#30312=CARTESIAN_POINT ( 'NONE',  ( 4.305481116379047180, 22.27104015248967173, -23.09767284345425509 ) ) ;
#30315=CARTESIAN_POINT ( 'NONE',  ( 17.34618997557657849, -22.82648989626997604, -15.08118710441591048 ) ) ;
#30320=CARTESIAN_POINT ( 'NONE',  ( 15.15030103098511383, 26.36342365734200399, -8.294678768621148279 ) ) ;
#30322=CARTESIAN_POINT ( 'NONE',  ( -11.51726355202159624, 17.19569276542222269, -27.48129831304505899 ) ) ;
#30325=CARTESIAN_POINT ( 'NONE',  ( 12.71338354207696497, 20.96606222537368325, -18.46259050867353579 ) ) ;
#30327=CARTESIAN_POINT ( 'NONE',  ( 32.65952487167601248, -19.32530057143253543, -7.543753945995782750 ) ) ;
#30329=CARTESIAN_POINT ( 'NONE',  ( -15.06956279710928293, 27.24103417575508246, -7.338594085143288481 ) ) ;
#30331=CARTESIAN_POINT ( 'NONE',  ( -12.01071536255492944, -19.67856823503798935, -21.46176309291517015 ) ) ;
#30336=CARTESIAN_POINT ( 'NONE',  ( -19.38376532770186600, -6.700500133912340672, -30.00000000000000711 ) ) ;
#30337=CARTESIAN_POINT ( 'NONE',  ( -12.02355362826419949, -22.03127078142710360, -17.46066762549815010 ) ) ;
#30340=CARTESIAN_POINT ( 'NONE',  ( 21.01898744346075887, 2.370978427325546534, -25.17228136638972913 ) ) ;
#30347=CARTESIAN_POINT ( 'NONE',  ( -20.48527248842334458, 0.7769947089114559446, -30.00000000000000000 ) ) ;
#30349=CARTESIAN_POINT ( 'NONE',  ( 23.60161110719205269, -0.2824371959814870880, -20.42950721209147602 ) ) ;
#30353=CARTESIAN_POINT ( 'NONE',  ( -27.59133651858127578, 3.518468992289588648, -6.427306901501287584 ) ) ;
#30354=EDGE_CURVE ( 'NONE', #31788, #8093, #14519, .T. ) ;
#30365=CARTESIAN_POINT ( 'NONE',  ( -24.79570961235407012, 6.146241236260801877, -10.32277382243248454 ) ) ;
#30369=CARTESIAN_POINT ( 'NONE',  ( 24.20444226731742177, -25.16656729849181673, -9.375567471260238150 ) ) ;
#30372=CARTESIAN_POINT ( 'NONE',  ( 15.17781109110005389, 26.90704365139002974, -7.347467770236907114 ) ) ;
#30376=CARTESIAN_POINT ( 'NONE',  ( -13.60555342264946432, 17.51225866673465248, -21.88651860859232201 ) ) ;
#30378=DIRECTION ( 'NONE',  ( 1.000000000000000000, 0.000000000000000000, 0.000000000000000000 ) ) ;
#30379=CARTESIAN_POINT ( 'NONE',  ( 11.20492248755046916, 17.74145648390907581, -26.22707998456911227 ) ) ;
#30381=CARTESIAN_POINT ( 'NONE',  ( 13.48758456246939375, 22.82324740036658994, -15.44989232396194723 ) ) ;
#30383=CARTESIAN_POINT ( 'NONE',  ( -15.24884605207680899, 26.67307980227703013, -7.353820275870864620 ) ) ;
#30385=CARTESIAN_POINT ( 'NONE',  ( -9.583030972882045972, -18.26713118289615068, -28.07671138377387621 ) ) ;
#30387=CARTESIAN_POINT ( 'NONE',  ( -18.22632359083961973, -10.26709115745145695, -26.96482044692446678 ) ) ;
#30388=CARTESIAN_POINT ( 'NONE',  ( -13.67153465227740305, -25.94622658622995814, -8.309525041132507894 ) ) ;
#30390=CARTESIAN_POINT ( 'NONE',  ( 15.89516500601641624, 24.02346326373800167, -8.316517264783472640 ) ) ;
#30392=CARTESIAN_POINT ( 'NONE',  ( 21.45806756224683554, 6.896564397286524262, -18.96977795570283831 ) ) ;
#30398=CARTESIAN_POINT ( 'NONE',  ( -27.89312612946301684, -0.8754152598143283281, -14.35503880984175495 ) ) ;
#30401=CARTESIAN_POINT ( 'NONE',  ( 25.94993652933962736, 0.1776616952070861344, -16.42543414208182639 ) ) ;
#30408=LINE ( 'NONE', #39733, #9263 ) ;
#30415=CARTESIAN_POINT ( 'NONE',  ( 0.2743609694596454984, 25.73594535306035525, -19.62891333975765207 ) ) ;
#30425=CARTESIAN_POINT ( 'NONE',  ( 11.44973932604695754, 21.65318152733180668, -19.31446654788366502 ) ) ;
#30429=CARTESIAN_POINT ( 'NONE',  ( -15.91172688669051283, 12.94523012445180399, -29.42231075624701475 ) ) ;
#30432=CARTESIAN_POINT ( 'NONE',  ( 10.24068639920821688, -19.15891185376089112, -23.85198230486452076 ) ) ;
#30434=CARTESIAN_POINT ( 'NONE',  ( 14.72828018990482235, 25.42434042747754219, -10.65132935642424350 ) ) ;
#30439=CARTESIAN_POINT ( 'NONE',  ( -19.60827666070207087, -16.31332699639156303, -19.71403864979324538 ) ) ;
#30440=CARTESIAN_POINT ( 'NONE',  ( 1.243865831159307822, -20.57034976483239319, -28.30086564174369457 ) ) ;
#30441=CARTESIAN_POINT ( 'NONE',  ( 11.24974104459727009, 17.28524465445085667, -28.08974055294966732 ) ) ;
#30442=CARTESIAN_POINT ( 'NONE',  ( 18.33234679620570873, 10.26058583535126267, -24.41653352660923204 ) ) ;
#30443=CARTESIAN_POINT ( 'NONE',  ( -17.34253826607186966, 27.32041144404027122, -5.000000000000000000 ) ) ;
#30444=CARTESIAN_POINT ( 'NONE',  ( -3.989573575045165743, 23.25966083313679889, -21.92851973090041184 ) ) ;
#30446=EDGE_CURVE ( 'NONE', #32040, #6084, #37833, .T. ) ;
#30451=CARTESIAN_POINT ( 'NONE',  ( -30.51074951646900857, 0.1921439302265571525, -6.888518465258303358 ) ) ;
#30453=CARTESIAN_POINT ( 'NONE',  ( 35.15679305665209142, -10.61876882962838486, -7.156232860489364356 ) ) ;
#30460=PLANE ( 'NONE',  #38502 ) ;
#30467=CARTESIAN_POINT ( 'NONE',  ( 16.64356867624101000, -11.98442300389733539, -29.21688973832524994 ) ) ;
#30469=CARTESIAN_POINT ( 'NONE',  ( 19.25847470691681096, 15.64464181457198322, -9.379364711887674844 ) ) ;
#30470=CARTESIAN_POINT ( 'NONE',  ( 6.931030674386980728, 19.37776282368324487, -28.55341591256747691 ) ) ;
#30472=CARTESIAN_POINT ( 'NONE',  ( -20.09127696847111366, 8.941272172551848030, -20.10129515931187072 ) ) ;
#30475=CARTESIAN_POINT ( 'NONE',  ( 15.16669826860400150, -26.03282984618214968, -9.229254182688153563 ) ) ;
#30477=CARTESIAN_POINT ( 'NONE',  ( 33.62187204924162387, 0.04418559750794539415, -5.000000000000000000 ) ) ;
#30478=CARTESIAN_POINT ( 'NONE',  ( -15.32703306334495785, 26.65709472084694909, -6.887131183944945612 ) ) ;
#30480=CARTESIAN_POINT ( 'NONE',  ( -23.88751137688053561, -26.63245304365073807, -5.000000000000000888 ) ) ;
#30481=CARTESIAN_POINT ( 'NONE',  ( 14.29043209799990777, -26.44292502402198863, -5.474004566143001682 ) ) ;
#30486=CARTESIAN_POINT ( 'NONE',  ( -10.82977346427968435, 32.86428370503693941, -8.960981340570279841 ) ) ;
#30487=CARTESIAN_POINT ( 'NONE',  ( 30.90412082983257136, -0.04211290444282138334, 0.000000000000000000 ) ) ;
#30492=CARTESIAN_POINT ( 'NONE',  ( 28.86207495170819826, 0.1351350256458582755, -11.60025332016630450 ) ) ;
#30497=CARTESIAN_POINT ( 'NONE',  ( -26.50117175307022421, 0.2815291374478115505, -15.45087338150947609 ) ) ;
#30499=ORIENTED_EDGE ( 'NONE', *, *, #115, .T. ) ;
#30500=CARTESIAN_POINT ( 'NONE',  ( 33.02287403607468264, -4.040597451033075771, -8.593868954784237957 ) ) ;
#30508=AXIS2_PLACEMENT_3D ( 'NONE', #26814, #33125, #39400 ) ;
#30513=VECTOR ( 'NONE', #21846, 1000.000000000000000 ) ;
#30516=CARTESIAN_POINT ( 'NONE',  ( 8.151676898411890804, 36.26115058741275732, -5.869408836369663263 ) ) ;
#30519=CARTESIAN_POINT ( 'NONE',  ( 12.21416419421548660, -19.63058848957433256, -21.43431398639220831 ) ) ;
#30520=SURFACE_STYLE_USAGE ( .BOTH. , #11822 ) ;
#30522=DIRECTION ( 'NONE',  ( 0.000000000000000000, 0.000000000000000000, 1.000000000000000000 ) ) ;
#30524=CARTESIAN_POINT ( 'NONE',  ( 14.81250384572173395, 25.69514127254151603, -10.17503788168345302 ) ) ;
#30526=CARTESIAN_POINT ( 'NONE',  ( -15.37753457773980870, 26.65290648949110874, -6.417023895753770191 ) ) ;
#30529=CARTESIAN_POINT ( 'NONE',  ( 10.79086491057129393, -20.00149296152361345, -21.62300246481197874 ) ) ;
#30531=CARTESIAN_POINT ( 'NONE',  ( 13.55580735823829208, 22.69008329597610540, -15.45968526880065141 ) ) ;
#30534=CARTESIAN_POINT ( 'NONE',  ( -15.19527047305266443, 27.50996873332976378, -5.470726252303037995 ) ) ;
#30536=CARTESIAN_POINT ( 'NONE',  ( -18.50146268769051261, -26.05940927080308001, -9.995050714716832374 ) ) ;
#30540=CARTESIAN_POINT ( 'NONE',  ( -21.26011989971568994, -8.067792608035599500, -23.06233089094039101 ) ) ;
#30541=CARTESIAN_POINT ( 'NONE',  ( -12.74073895253298616, -23.07826477149550826, -15.46828449374485892 ) ) ;
#30544=CARTESIAN_POINT ( 'NONE',  ( 20.64171730712855535, 2.398676254270919017, -26.94157980996323687 ) ) ;
#30550=CARTESIAN_POINT ( 'NONE',  ( -30.25321886983080333, -0.06122810112208476596, -8.763529956286015832 ) ) ;
#30552=CARTESIAN_POINT ( 'NONE',  ( 20.49959133494802543, 0.2219702378425628120, -29.33667080960374562 ) ) ;
#30555=CARTESIAN_POINT ( 'NONE',  ( -20.68010352585984535, 2.885225430730191221, -26.38554717714988129 ) ) ;
#30565=CARTESIAN_POINT ( 'NONE',  ( -21.17445498011162996, 7.452892634864654475, -18.99389871435994337 ) ) ;
#30568=CARTESIAN_POINT ( 'NONE',  ( 22.95814010875989197, -22.53209843378533606, -12.99612941548552492 ) ) ;
#30572=CARTESIAN_POINT ( 'NONE',  ( 14.83882917549554037, 26.09951300090577320, -9.692528519113288610 ) ) ;
#30575=CARTESIAN_POINT ( 'NONE',  ( -12.39465856751968609, 16.66586351761176843, -26.93958671274752348 ) ) ;
#30578=CARTESIAN_POINT ( 'NONE',  ( 12.94545362548832124, 21.62528871782362216, -17.44060035758700522 ) ) ;
#30583=CARTESIAN_POINT ( 'NONE',  ( -14.95596380865394970, 26.16937309837150138, -9.228359069169592033 ) ) ;
#30585=CARTESIAN_POINT ( 'NONE',  ( -13.40009855081921053, -23.62524794187952892, -14.47403050587199225 ) ) ;
#30588=CARTESIAN_POINT ( 'NONE',  ( -17.63393726088407121, -10.64200091597105846, -28.44387009623618212 ) ) ;
#30589=CARTESIAN_POINT ( 'NONE',  ( -12.39553123186617611, -23.97331200851148125, -13.57268788837447637 ) ) ;
#30591=CARTESIAN_POINT ( 'NONE',  ( 16.25725326718474406, 23.79337420548043980, -6.422359314754682025 ) ) ;
#30593=CARTESIAN_POINT ( 'NONE',  ( 23.36873701481537680, 7.189358073232670954, -12.82796446375462551 ) ) ;
#30599=CARTESIAN_POINT ( 'NONE',  ( -28.28993293699624090, -0.5497182594458693838, -13.43537464208401033 ) ) ;
#30600=CARTESIAN_POINT ( 'NONE',  ( 30.76969935483850804, -0.1781414310780859711, -7.352071795213825922 ) ) ;
#30603=CARTESIAN_POINT ( 'NONE',  ( 33.62187204924162387, 0.04418559750795045954, -13.79123840944733992 ) ) ;
#30610=CARTESIAN_POINT ( 'NONE',  ( 2.163616898793370602, 30.08412298609989222, -15.68737937765401291 ) ) ;
#30619=CARTESIAN_POINT ( 'NONE',  ( 14.77611408087021694, 27.12164188139913534, -8.725285341602761591 ) ) ;
#30622=CARTESIAN_POINT ( 'NONE',  ( -19.20284012471338642, 16.64839643360665633, -5.480717218555573034 ) ) ;
#30627=CARTESIAN_POINT ( 'NONE',  ( 14.36179435970547402, -25.07121135651426869, -11.59890311405379748 ) ) ;
#30629=CARTESIAN_POINT ( 'NONE',  ( -22.42780984720763371, -26.55233249316436428, -7.652769933138617198 ) ) ;
#30631=CARTESIAN_POINT ( 'NONE',  ( 14.51908200401363302, 25.00878969398502960, -11.59620987194703012 ) ) ;
#30636=CARTESIAN_POINT ( 'NONE',  ( -28.98287275701582644, -24.11882464604644127, -5.863716236549250560 ) ) ;
#30637=CARTESIAN_POINT ( 'NONE',  ( -0.3811350534766741460, -24.48451870251001594, -8.900403566480946438 ) ) ;
#30638=CARTESIAN_POINT ( 'NONE',  ( 11.51224750557763699, 17.87894272431910991, -25.04142208898249677 ) ) ;
#30639=CARTESIAN_POINT ( 'NONE',  ( 17.89753197511066674, 10.02670602479014228, -29.99999999999999645 ) ) ;
#30641=CARTESIAN_POINT ( 'NONE',  ( -4.212426069905327530, 37.97930161814787198, -5.436632083248686520 ) ) ;
#30643=CARTESIAN_POINT ( 'NONE',  ( -33.92430155621369892, -6.368002694854169476, -8.531665187152857044 ) ) ;
#30650=CARTESIAN_POINT ( 'NONE',  ( -20.46571904345125148, 1.196608941699672357, -30.00000000000000000 ) ) ;
#30651=CARTESIAN_POINT ( 'NONE',  ( 34.48754613114789436, -12.67185989539148849, -8.433237745870078683 ) ) ;
#30661=CARTESIAN_POINT ( 'NONE',  ( -2.340242103211412239, 21.29936263313340206, -25.60352335172182947 ) ) ;
#30666=CARTESIAN_POINT ( 'NONE',  ( 28.95584039848980140, -23.67695839038157857, -7.136634946781046374 ) ) ;
#30667=CARTESIAN_POINT ( 'NONE',  ( 16.46100146899417993, 13.93030935198141229, -22.17668661662577279 ) ) ;
#30668=CARTESIAN_POINT ( 'NONE',  ( 7.299606265389828152, 20.47042108248343695, -24.54268700408873372 ) ) ;
#30670=CARTESIAN_POINT ( 'NONE',  ( -21.80410373500361487, 11.76501844773795824, -5.967298349106835431 ) ) ;
#30673=CARTESIAN_POINT ( 'NONE',  ( 12.80584978270169394, -22.56157762115984866, -16.42713908487053587 ) ) ;
#30676=CARTESIAN_POINT ( 'NONE',  ( -15.40119896161133006, 26.83624744099596171, -5.000000000000001776 ) ) ;
#30677=CARTESIAN_POINT ( 'NONE',  ( -22.86303537443307476, -25.58751383834528070, -9.408386063524703857 ) ) ;
#30678=CARTESIAN_POINT ( 'NONE',  ( 10.74915096743506027, -25.64641579889018885, -5.950130972811642494 ) ) ;
#30683=CARTESIAN_POINT ( 'NONE',  ( -10.96238246107026626, 33.32429186611522454, -8.073152806041559160 ) ) ;
#30688=CARTESIAN_POINT ( 'NONE',  ( 27.73864469095863683, 0.1886746684874264501, -13.51343220089273167 ) ) ;
#30693=CARTESIAN_POINT ( 'NONE',  ( -20.48057623381365033, 0.8922431241703840943, -29.34897116163656960 ) ) ;
#30697=CARTESIAN_POINT ( 'NONE',  ( 31.61045151917019069, -6.540495618978702907, -12.13482048140255287 ) ) ;
#30701=DIRECTION ( 'NONE',  ( 1.000000000000000000, 0.000000000000000000, -0.000000000000000000 ) ) ;
#30711=CARTESIAN_POINT ( 'NONE',  ( 8.159785424745114923, 36.31054560068550785, -5.440753753161995832 ) ) ;
#30716=CARTESIAN_POINT ( 'NONE',  ( 12.51578678884064466, -18.90026018402930674, -22.47850626938384266 ) ) ;
#30717=( NAMED_UNIT ( * ) PLANE_ANGLE_UNIT ( ) SI_UNIT ( $, .RADIAN. ) );
#30722=CARTESIAN_POINT ( 'NONE',  ( -13.34174550214330957, 22.00054098145283277, -16.46453111791931079 ) ) ;
#30725=CARTESIAN_POINT ( 'NONE',  ( 15.16712867651880003, -26.63505783696666640, -5.946131006634350236 ) ) ;
#30729=CARTESIAN_POINT ( 'NONE',  ( -11.09811852199402082, 22.05552288639037073, -19.25227300847279110 ) ) ;
#30730=CARTESIAN_POINT ( 'NONE',  ( -13.36679029698933086, -19.22344594692958708, -21.28930016379315404 ) ) ;
#30731=CARTESIAN_POINT ( 'NONE',  ( -1.485571585149978668, -11.24999999999982236, 3.000000000000000000 ) ) ;
#30732=ORIENTED_EDGE ( 'NONE', *, *, #32717, .T. ) ;
#30733=CARTESIAN_POINT ( 'NONE',  ( -35.47307300072858283, -9.938437602308624719, -5.442375005290738699 ) ) ;
#30734=CARTESIAN_POINT ( 'NONE',  ( -9.245064759184387526, -18.29713783020200424, -30.00000000000000000 ) ) ;
#30737=CARTESIAN_POINT ( 'NONE',  ( 20.51663963794920065, 1.053696994703543055, -28.71375515118313970 ) ) ;
#30743=CARTESIAN_POINT ( 'NONE',  ( -23.97549446410291552, 0.4047595829504309628, -19.48518163238001577 ) ) ;
#30746=CARTESIAN_POINT ( 'NONE',  ( 30.19373506806564933, -1.611421832312862179, -11.45916374511738489 ) ) ;
#30748=CARTESIAN_POINT ( 'NONE',  ( 13.80182853280054900, -15.17292971133294444, -30.00000000000000355 ) ) ;
#30751=CARTESIAN_POINT ( 'NONE',  ( -27.53998928449781047, 3.518557584072389943, -6.903689457210364644 ) ) ;
#30752=CARTESIAN_POINT ( 'NONE',  ( -30.90412082983255715, -0.04211290444283005696, -5.000000000000000000 ) ) ;
#30755=CARTESIAN_POINT ( 'NONE',  ( -18.00000000000000000, 22.50000000000001066, 6.000000000000000000 ) ) ;
#30763=CARTESIAN_POINT ( 'NONE',  ( -24.79671477329043228, 7.114048960549892442, -6.442296327763719965 ) ) ;
#30766=CARTESIAN_POINT ( 'NONE',  ( 14.27600272946170890, -15.79691008733334634, -25.79950180772068080 ) ) ;
#30767=CARTESIAN_POINT ( 'NONE',  ( 0.000000000000000000, 22.50000000000000355, 6.000000000000000000 ) ) ;
#30768=CARTESIAN_POINT ( 'NONE',  ( 15.29414933734400428, 26.94219312171647118, -6.412878494969166177 ) ) ;
#30771=CARTESIAN_POINT ( 'NONE',  ( -12.27438659830399104, 16.41897796854597047, -29.37404837115920131 ) ) ;
#30774=CARTESIAN_POINT ( 'NONE',  ( 13.22333277151671105, 22.21094483373017425, -16.44622722129113512 ) ) ;
#30775=ORIENTED_EDGE ( 'NONE', *, *, #17882, .T. ) ;
#30778=CARTESIAN_POINT ( 'NONE',  ( -15.25716400807983142, 26.89584191905160537, -6.881959249777203524 ) ) ;
#30780=CARTESIAN_POINT ( 'NONE',  ( -14.49768878875645051, -25.09694979747337484, -11.58902682695292441 ) ) ;
#30782=CARTESIAN_POINT ( 'NONE',  ( -31.54497719551462609, -17.75878470093167039, -10.17196054166158348 ) ) ;
#30784=CARTESIAN_POINT ( 'NONE',  ( -12.10239668256580003, -23.52241704728540128, -14.54534583956947102 ) ) ;
#30786=CARTESIAN_POINT ( 'NONE',  ( 15.11671161907844585, 23.43369355923603337, -11.64535646599357577 ) ) ;
#30788=CARTESIAN_POINT ( 'NONE',  ( 25.58814899322283409, 5.549420531236951781, -8.847774912381147772 ) ) ;
#30793=CARTESIAN_POINT ( 'NONE',  ( -24.35468204290444660, -0.5538618444963721021, -19.35839232206769367 ) ) ;
#30796=CARTESIAN_POINT ( 'NONE',  ( 20.48413544616686011, 0.8063757131868728445, -29.34740462186751486 ) ) ;
#30800=CARTESIAN_POINT ( 'NONE',  ( 17.34253826539385201, 27.32041144647958575, -5.000000000000000000 ) ) ;
#30807=CARTESIAN_POINT ( 'NONE',  ( 1.613298393356113136, 22.76613432878109222, -22.99758612101997102 ) ) ;
#30816=CARTESIAN_POINT ( 'NONE',  ( 11.93556763155846134, 21.07774700547179236, -19.40385465495243977 ) ) ;
#30819=CARTESIAN_POINT ( 'NONE',  ( -17.32349603665394966, 15.91288547668971631, -15.86201918625455853 ) ) ;
#30822=CARTESIAN_POINT ( 'NONE',  ( 9.704060306507821920, -18.43476937023081419, -26.82927739930571320 ) ) ;
#30823=CARTESIAN_POINT ( 'NONE',  ( -12.79957064338231554, -17.39491785756841935, -24.68155700860378232 ) ) ;
#30824=CARTESIAN_POINT ( 'NONE',  ( 14.93529390890676822, 25.79829262747118790, -9.709001792061668468 ) ) ;
#30825=CARTESIAN_POINT ( 'NONE',  ( 14.02229904730994292, 23.95306976838152480, -13.51159946331490147 ) ) ;
#30828=CARTESIAN_POINT ( 'NONE',  ( -15.43577743098634159, -26.72909887300547283, -5.000000000000000888 ) ) ;
#30831=CARTESIAN_POINT ( 'NONE',  ( -28.07145589138256270, -22.01881091388684197, -10.19667367662031054 ) ) ;
#30832=CARTESIAN_POINT ( 'NONE',  ( -0.2799713375976506380, -20.99526500827598596, -24.41369975650612645 ) ) ;
#30833=CARTESIAN_POINT ( 'NONE',  ( 12.95423034502591442, 20.61663634441624993, -18.50330793998235990 ) ) ;
#30834=CARTESIAN_POINT ( 'NONE',  ( 20.50834976286951772, 11.43410818086181280, -13.90707920088669702 ) ) ;
#30836=CARTESIAN_POINT ( 'NONE',  ( -5.213701606270112698, 36.61873165587430634, -8.423533786119408617 ) ) ;
#30838=CARTESIAN_POINT ( 'NONE',  ( -23.49268708087237201, -3.611016997205812373, -21.11844712770017907 ) ) ;
#30841=FACE_BOUND ( 'NONE', #12369, .T. ) ;
#30844=CARTESIAN_POINT ( 'NONE',  ( -30.25911448991262276, 0.6236314785230308022, -5.000000000000000000 ) ) ;
#30845=CARTESIAN_POINT ( 'NONE',  ( 30.88550645483323009, -11.32616882505672784, -12.93498916185149028 ) ) ;
#30848=ORIENTED_EDGE ( 'NONE', *, *, #16868, .F. ) ;
#30859=CARTESIAN_POINT ( 'NONE',  ( -4.123717629018512021, 36.95811013929738920, -8.415836676720722664 ) ) ;
#30863=CARTESIAN_POINT ( 'NONE',  ( 28.01677963356848622, -22.94489307428302993, -9.311317233667166349 ) ) ;
#30864=CARTESIAN_POINT ( 'NONE',  ( 19.75473557947194436, 14.68794674279743795, -9.387208291950921435 ) ) ;
#30865=CARTESIAN_POINT ( 'NONE',  ( 11.34888309589563882, 25.00279730542691325, -16.12364529934884771 ) ) ;
#30867=CARTESIAN_POINT ( 'NONE',  ( -17.90340069958895697, 10.65400709177240302, -25.51243598403177870 ) ) ;
#30870=CARTESIAN_POINT ( 'NONE',  ( 11.63721313908758681, -20.96583099751724077, -19.48517461635267267 ) ) ;
#30872=CARTESIAN_POINT ( 'NONE',  ( -3.859759734048395785E-14, -22.74351282448223799, -30.00000000000000355 ) ) ;
#30874=CARTESIAN_POINT ( 'NONE',  ( -14.72734366533763506, 25.42720644217061832, -10.65114164413067677 ) ) ;
#30875=CARTESIAN_POINT ( 'NONE',  ( -13.61442942725709315, -16.31983737738216433, -25.85608801652313460 ) ) ;
#30876=CARTESIAN_POINT ( 'NONE',  ( 12.98099092732498683, -25.97363603336197357, -7.367975789372572137 ) ) ;
#30879=CARTESIAN_POINT ( 'NONE',  ( -6.485893174894165725, 19.45725460019876252, -29.99999999999998224 ) ) ;
#30885=CARTESIAN_POINT ( 'NONE',  ( 30.68637370779745055, 0.009861439750234452309, -6.888001205752280143 ) ) ;
#30890=CARTESIAN_POINT ( 'NONE',  ( -29.96087079451076818, 0.06295573032941799430, -9.238980554428115610 ) ) ;
#30894=CARTESIAN_POINT ( 'NONE',  ( 30.54975010973276994, -5.406317539725979948, -13.10619709277712985 ) ) ;
#30908=CARTESIAN_POINT ( 'NONE',  ( 4.496862015843432481, 20.00989232716073118, -30.00000000000000000 ) ) ;
#30914=CARTESIAN_POINT ( 'NONE',  ( 15.14693761635412983, -23.74175418701464579, -14.31586175695692020 ) ) ;
#30919=CARTESIAN_POINT ( 'NONE',  ( -14.14736404216506571, 23.66099997246980635, -13.52656865009267406 ) ) ;
#30921=CARTESIAN_POINT ( 'NONE',  ( 13.13573601262098478, -23.60207374655375645, -14.48926436058232881 ) ) ;
#30925=CARTESIAN_POINT ( 'NONE',  ( -13.81624380675895836, 30.37090005602236431, -6.364651089629193237 ) ) ;
#30926=CARTESIAN_POINT ( 'NONE',  ( -20.14086777909864168, -26.69671822894133228, -8.145045410496569716 ) ) ;
#30930=CARTESIAN_POINT ( 'NONE',  ( -22.56600422072800782, -6.300902944093242475, -22.03183368421533928 ) ) ;
#30931=CARTESIAN_POINT ( 'NONE',  ( -15.18562876168915565, -26.54301761587689867, -6.888309856460237413 ) ) ;
#30934=CARTESIAN_POINT ( 'NONE',  ( 30.54320699650084947, 0.2260830151874697325, -6.417392023155034764 ) ) ;
#30938=CARTESIAN_POINT ( 'NONE',  ( -29.83105174024096229, 0.01200203450569401441, -9.707336131520873934 ) ) ;
#30941=CARTESIAN_POINT ( 'NONE',  ( 22.47524216860800195, -0.4976999769275546881, -22.58728816505331949 ) ) ;
#30943=CYLINDRICAL_SURFACE ( 'NONE', #34964, 18.00000000000000000 ) ;
#30946=CARTESIAN_POINT ( 'NONE',  ( -26.88094701073862325, 3.517601285915260334, -9.781306404757943440 ) ) ;
#30948=CYLINDRICAL_SURFACE ( 'NONE', #23898, 18.00000000000002487 ) ;
#30953=CARTESIAN_POINT ( 'NONE',  ( -22.10669899577159825, 7.630206710036005369, -15.88546095289416016 ) ) ;
#30956=CARTESIAN_POINT ( 'NONE',  ( 15.60359587640040679, -17.23679362701221152, -22.13449739431376884 ) ) ;
#30959=CARTESIAN_POINT ( 'NONE',  ( 14.94231797702671471, 26.21208174917623523, -9.226265064744874067 ) ) ;
#30961=EDGE_LOOP ( 'NONE', ( #2559, #30499, #31955, #26347, #33188, #27363, #31637 ) ) ;
#30962=CARTESIAN_POINT ( 'NONE',  ( -15.94479093369340106, 23.58249151255476406, -8.795490714381706709 ) ) ;
#30965=CARTESIAN_POINT ( 'NONE',  ( 15.44165670342503205, 26.69129292160669920, -5.474180254959668090 ) ) ;
#30970=CARTESIAN_POINT ( 'NONE',  ( -14.65347711145498444, 25.64673223685113612, -10.63691246398533430 ) ) ;
#30972=CARTESIAN_POINT ( 'NONE',  ( -12.01613607123918648, -21.47750082395870663, -18.43867415038402768 ) ) ;
#30976=CARTESIAN_POINT ( 'NONE',  ( -24.72872997693725949, -12.95474267484971698, -17.60025526371827098 ) ) ;
#30977=CARTESIAN_POINT ( 'NONE',  ( -13.85493750717612471, -26.22870991353853753, -6.891751044494506928 ) ) ;
#30979=CARTESIAN_POINT ( 'NONE',  ( 15.59579652599576782, 23.45568014046210337, -10.22222026387747107 ) ) ;
#30981=CARTESIAN_POINT ( 'NONE',  ( 26.01521168343815305, 5.578082495604143709, -5.477568960753655958 ) ) ;
#30984=FACE_OUTER_BOUND ( 'NONE', #21942, .T. ) ;
#30986=CARTESIAN_POINT ( 'NONE',  ( -30.25735003896744857, -0.2604941155819015530, -9.220310513660999518 ) ) ;
#30987=ADVANCED_FACE ( 'NONE', ( #36750, #15008 ), #30460, .T. ) ;
#30988=CARTESIAN_POINT ( 'NONE',  ( 20.70339734419210131, 0.6992704487685735826, -27.43878474189266115 ) ) ;
#30993=CARTESIAN_POINT ( 'NONE',  ( 37.49625565938770677, -14.69322820095495530, -14.45070082761205832 ) ) ;
#31001=AXIS2_PLACEMENT_3D ( 'NONE', #21449, #25091, #40131 ) ;
#31005=CARTESIAN_POINT ( 'NONE',  ( 2.666049144303739293, 36.98651336572240922, -8.847562779496046304 ) ) ;
#31006=FACE_OUTER_BOUND ( 'NONE', #30307, .T. ) ;
#31014=CARTESIAN_POINT ( 'NONE',  ( 13.93706817763407457, 25.34829717239110991, -12.47786359530666900 ) ) ;
#31017=CARTESIAN_POINT ( 'NONE',  ( -17.52995626189967737, 16.16943778198609749, -14.84323570916496493 ) ) ;
#31020=CARTESIAN_POINT ( 'NONE',  ( 15.38694898889602136, -26.59324455761997896, -6.887897242969529543 ) ) ;
#31021=CARTESIAN_POINT ( 'NONE',  ( -21.59438778490832789, -27.03632430179366963, -6.341461391377428924 ) ) ;
#31022=CARTESIAN_POINT ( 'NONE',  ( 14.73787879266531853, 25.39503920881752208, -10.65324680268566127 ) ) ;
#31023=CARTESIAN_POINT ( 'NONE',  ( 10.98733276423893201, 17.36017109950246251, -28.70617518134429602 ) ) ;
#31026=CARTESIAN_POINT ( 'NONE',  ( -11.45863972089735405, -20.98773559138341227, -19.50614846912421996 ) ) ;
#31030=CARTESIAN_POINT ( 'NONE',  ( -29.70672294952053250, -21.88546735577168789, -8.854887924351043438 ) ) ;
#31031=CARTESIAN_POINT ( 'NONE',  ( -2.582945274031032579, -24.71752041314383774, -6.939050857786467574 ) ) ;
#31032=CARTESIAN_POINT ( 'NONE',  ( 12.38854343360681654, 19.61926878829738996, -20.58590829373904540 ) ) ;
#31033=CARTESIAN_POINT ( 'NONE',  ( 22.57201939060207252, 10.08208122992440003, -8.403798546843612272 ) ) ;
#31035=CARTESIAN_POINT ( 'NONE',  ( -2.937749330471188358, 20.92723910012711031, -26.29585176386288126 ) ) ;
#31039=CARTESIAN_POINT ( 'NONE',  ( -34.60931334941528803, -6.532660442264273115, -6.767915967295159874 ) ) ;
#31047=CARTESIAN_POINT ( 'NONE',  ( -22.56602591100718769, 1.155315371689267012, -21.68362715205212155 ) ) ;
#31048=CARTESIAN_POINT ( 'NONE',  ( 32.45817255219479591, -13.02753558049290561, -11.09164157653418847 ) ) ;
#31057=CARTESIAN_POINT ( 'NONE',  ( -3.698881800131589070, 33.04102055638166746, -12.90738243435495747 ) ) ;
#31062=CARTESIAN_POINT ( 'NONE',  ( 16.59050531452238175, -12.72231626870975774, -26.99548381761250937 ) ) ;
#31063=CARTESIAN_POINT ( 'NONE',  ( 15.77861697390694395, 13.11959191132365099, -28.84590463088538570 ) ) ;
#31064=CARTESIAN_POINT ( 'NONE',  ( 11.41068916750651674, 27.22167306763704175, -14.12609294827662154 ) ) ;
#31066=CARTESIAN_POINT ( 'NONE',  ( -19.48170590106686717, 10.58249606826150035, -19.06244706679226297 ) ) ;
#31068=CARTESIAN_POINT ( 'NONE',  ( 14.53923885275054495, -25.10454186404201238, -11.58604102348432896 ) ) ;
#31071=CARTESIAN_POINT ( 'NONE',  ( 7.289639608743136989, -27.06962010326278545, -13.42901749168595593 ) ) ;
#31073=CARTESIAN_POINT ( 'NONE',  ( -15.32247945677889334, 26.67302399322529283, -6.886783351072488735 ) ) ;
#31074=CARTESIAN_POINT ( 'NONE',  ( -19.96046382237359751, -23.75384511009722033, -13.10646546221969544 ) ) ;
#31075=CARTESIAN_POINT ( 'NONE',  ( 8.289791691739285540, -18.78981145098772387, -28.75044738397058808 ) ) ;
#31076=CARTESIAN_POINT ( 'NONE',  ( 18.89841941734945152, -12.77170018320259182, -23.00035857315318921 ) ) ;
#31079=CARTESIAN_POINT ( 'NONE',  ( -11.13950323990193603, 33.98129016598238650, -5.885180931403255933 ) ) ;
#31086=CARTESIAN_POINT ( 'NONE',  ( 28.33402286304662709, 0.1460920933068121652, -12.55056911448999379 ) ) ;
#31087=CARTESIAN_POINT ( 'NONE',  ( 15.41558956984165363, 26.78481017248027740, -5.000000000000000000 ) ) ;
#31088=CARTESIAN_POINT ( 'NONE',  ( -1.829593030691901284E-15, 22.50000000000001066, 0.000000000000000000 ) ) ;
#31092=CARTESIAN_POINT ( 'NONE',  ( -30.56608372293882780, 0.03382379541455289573, -7.358089190805260138 ) ) ;
#31095=CARTESIAN_POINT ( 'NONE',  ( 21.32230761661163143, -4.380135932481430849, -24.50474909882916918 ) ) ;
#31108=CARTESIAN_POINT ( 'NONE',  ( 8.739825649919259476, 33.88938738370909931, -9.801802266497743332 ) ) ;
#31111=CARTESIAN_POINT ( 'NONE',  ( 17.32315637682313536, -26.79968999324490753, -7.764865353756197131 ) ) ;
#31116=CARTESIAN_POINT ( 'NONE',  ( -12.41574746403112073, 20.45786098935373687, -19.50078492736341573 ) ) ;
#31118=CARTESIAN_POINT ( 'NONE',  ( 13.78902572764358503, -24.57398664863276139, -12.55976489257005646 ) ) ;
#31124=CARTESIAN_POINT ( 'NONE',  ( -9.599378963044831181, 18.58950176588487224, -26.68917543542165305 ) ) ;
#31125=CARTESIAN_POINT ( 'NONE',  ( -12.96962488765257859, -18.70490450770867596, -22.42242649434588486 ) ) ;
#31128=CARTESIAN_POINT ( 'NONE',  ( -31.02555858839200553, -8.613196645477771085, -12.99421017137874479 ) ) ;
#31129=CARTESIAN_POINT ( 'NONE',  ( -9.680704677217148557, -18.61067064102984148, -26.23473070599376911 ) ) ;
#31132=CARTESIAN_POINT ( 'NONE',  ( 30.24006331749171039, 0.2466258206598069269, -7.829658031761377757 ) ) ;
#31136=CARTESIAN_POINT ( 'NONE',  ( -20.81788500015936805, 0.8029186697791972360, -26.82846150896363469 ) ) ;
#31138=CARTESIAN_POINT ( 'NONE',  ( 23.12890676149806168, -0.9096562629385716026, -21.41733200613340315 ) ) ;
#31140=APPLICATION_CONTEXT ( 'automotive_design' ) ;
#31145=CARTESIAN_POINT ( 'NONE',  ( -25.89993925104446504, 4.384403972809999495, -10.77364034502635093 ) ) ;
#31154=CARTESIAN_POINT ( 'NONE',  ( -20.37168883225173843, 6.509893064140952923, -23.23508475207167834 ) ) ;
#31155=DIRECTION ( 'NONE',  ( 0.000000000000000000, 0.000000000000000000, 1.000000000000000000 ) ) ;
#31157=CARTESIAN_POINT ( 'NONE',  ( 23.01790674491153155, -26.73296861964898241, -6.329011521549396946 ) ) ;
#31160=CARTESIAN_POINT ( 'NONE',  ( 11.49726645599677077, 19.09130336471316980, -22.70238085401357253 ) ) ;
#31162=CARTESIAN_POINT ( 'NONE',  ( -15.60095462958403978, 23.83721962407788908, -9.740729558853310266 ) ) ;
#31165=CARTESIAN_POINT ( 'NONE',  ( 11.06517245712214859, 17.40842300371218698, -28.07890772714004868 ) ) ;
#31169=CARTESIAN_POINT ( 'NONE',  ( -15.33616239741719234, 27.06134930142311745, -5.000000000000000888 ) ) ;
#31171=CARTESIAN_POINT ( 'NONE',  ( -15.68099505712324060, -26.76486360534729414, -5.943857969596352042 ) ) ;
#31174=CARTESIAN_POINT ( 'NONE',  ( -34.19171386303132465, -16.60390462771976416, -7.120391363458460354 ) ) ;
#31175=CARTESIAN_POINT ( 'NONE',  ( -8.172265125310115508, -20.22694128226171273, -23.00038051252499116 ) ) ;
#31177=CARTESIAN_POINT ( 'NONE',  ( 16.47653236464018889, 23.28601002705642742, -5.949066710759219667 ) ) ;
#31179=CARTESIAN_POINT ( 'NONE',  ( 25.05645393585312064, 4.615297387997106426, -12.74457131153767619 ) ) ;
#31184=CARTESIAN_POINT ( 'NONE',  ( -29.60645268812572084, -0.2125446482488342892, -10.63052326569164663 ) ) ;
#31185=CARTESIAN_POINT ( 'NONE',  ( 30.41973907439335534, -0.2412478344116361639, -8.753233025701321779 ) ) ;
#31191=CARTESIAN_POINT ( 'NONE',  ( -17.81784622497958281, -13.85677843414106292, -19.80438750953545579 ) ) ;
#31198=CARTESIAN_POINT ( 'NONE',  ( 1.827785273732315696, 25.64871398411360559, -19.64121285127799865 ) ) ;
#31204=EDGE_CURVE ( 'NONE', #20904, #19280, #22290, .T. ) ;
#31206=CARTESIAN_POINT ( 'NONE',  ( 14.98678706335186028, 28.02796269202450929, -5.933300154731170117 ) ) ;
#31210=CARTESIAN_POINT ( 'NONE',  ( -15.63638767905510463, 15.05447610871748232, -22.11642785074873174 ) ) ;
#31215=CARTESIAN_POINT ( 'NONE',  ( 12.25532247806346930, -22.02373625454399786, -17.44060027023390091 ) ) ;
#31216=CARTESIAN_POINT ( 'NONE',  ( -15.74452436455642967, -19.93752133503633317, -19.02658665625699896 ) ) ;
#31217=CARTESIAN_POINT ( 'NONE',  ( 11.12593219165437652, 17.61232244839224492, -26.83050114061178704 ) ) ;
#31218=CARTESIAN_POINT ( 'NONE',  ( 11.29390759324882509, 18.05061880014659792, -25.01236529811382781 ) ) ;
#31221=CARTESIAN_POINT ( 'NONE',  ( -13.27830748821643425, -23.61430804126850092, -14.48142061928604818 ) ) ;
#31224=CARTESIAN_POINT ( 'NONE',  ( -30.48519299957962048, -21.05274509396561555, -8.849016827759179193 ) ) ;
#31225=CARTESIAN_POINT ( 'NONE',  ( -0.3766544288610457758, -24.32970240761073555, -9.889122670036343266 ) ) ;
#31226=CARTESIAN_POINT ( 'NONE',  ( 14.91791411132470380, 23.94192138950630877, -11.62984915953536458 ) ) ;
#31227=CARTESIAN_POINT ( 'NONE',  ( 18.31926634591793501, 9.392207553935453035, -27.73388598276786965 ) ) ;
#31231=CARTESIAN_POINT ( 'NONE',  ( -31.10576488114211102, -3.143594509563115924, -11.36259591356684062 ) ) ;
#31237=CARTESIAN_POINT ( 'NONE',  ( -20.57568126879977299, 1.353978323836376507, -28.10186790039112026 ) ) ;
#31239=CARTESIAN_POINT ( 'NONE',  ( 20.00198754538222445, -6.713423164100702500, -26.34058677862946851 ) ) ;
#31250=VERTEX_POINT ( 'NONE', #35498 ) ;
#31251=CARTESIAN_POINT ( 'NONE',  ( -3.459042231567057257, 30.96747855261283178, -14.75290876766932335 ) ) ;
#31253=DIRECTION ( 'NONE',  ( 1.000000000000000000, 0.000000000000000000, 0.000000000000000000 ) ) ;
#31259=CARTESIAN_POINT ( 'NONE',  ( 10.45266244534071021, 24.84435709915603852, -17.03677774345998230 ) ) ;
#31261=CARTESIAN_POINT ( 'NONE',  ( -20.65776629622001082, 13.64123596302417241, -6.939388818800391157 ) ) ;
#31264=CARTESIAN_POINT ( 'NONE',  ( 11.31736706274068460, -20.44517872681216986, -20.52400851952886285 ) ) ;
#31266=CARTESIAN_POINT ( 'NONE',  ( 13.99558646605622414, 24.01852084437423684, -13.50539560667067107 ) ) ;
#31267=CARTESIAN_POINT ( 'NONE',  ( 37.62663912510992503, -8.659558992827964374, -5.000000000000018652 ) ) ;
#31269=CARTESIAN_POINT ( 'NONE',  ( -17.19550777949286768, -18.19888545701767768, -19.88174267863434608 ) ) ;
#31270=CARTESIAN_POINT ( 'NONE',  ( 12.41040698953132448, -25.06815925899662645, -10.70177142058002140 ) ) ;
#31271=CARTESIAN_POINT ( 'NONE',  ( 11.10914253955145448, 17.37933916143984447, -28.08151274450654711 ) ) ;
#31272=CARTESIAN_POINT ( 'NONE',  ( 31.02556648718628196, -22.39342206112319289, -5.436432259396653421 ) ) ;
#31277=CARTESIAN_POINT ( 'NONE',  ( -11.05743542808008506, 33.66909318204464086, -7.195062545379004249 ) ) ;
#31281=ORIENTED_EDGE ( 'NONE', *, *, #39802, .T. ) ;
#31282=CARTESIAN_POINT ( 'NONE',  ( 29.79977705054515269, 0.04608879464290485672, -9.709215146590867818 ) ) ;
#31283=CARTESIAN_POINT ( 'NONE',  ( -11.06069781764612081, 34.19033620402620954, -4.999999999999999112 ) ) ;
#31287=CARTESIAN_POINT ( 'NONE',  ( -26.48491323965393462, 0.3066557059962052301, -15.45283448520972769 ) ) ;
#31289=VERTEX_POINT ( 'NONE', #4208 ) ;
#31290=CARTESIAN_POINT ( 'NONE',  ( 35.04727437832835335, -7.360793022001182351, -5.000000000000008882 ) ) ;
#31302=CARTESIAN_POINT ( 'NONE',  ( -5.728515882982030405, 19.68564878121862094, -29.99999999999996803 ) ) ;
#31304=CARTESIAN_POINT ( 'NONE',  ( 17.03483695331121339, 19.02378625293593473, -11.77568025449220457 ) ) ;
#31305=CARTESIAN_POINT ( 'NONE',  ( 4.514778716083354126, 20.08757060652311921, -28.49112518072664813 ) ) ;
#31306=CARTESIAN_POINT ( 'NONE',  ( 10.66098508067554995, -17.52284468788354843, -30.00000000000000000 ) ) ;
#31310=CARTESIAN_POINT ( 'NONE',  ( -14.54807450344172892, 24.92773171820151035, -11.60025354066594794 ) ) ;
#31313=CARTESIAN_POINT ( 'NONE',  ( 14.47253599967204529, -25.59814919913764442, -10.18550332105856349 ) ) ;
#31317=CARTESIAN_POINT ( 'NONE',  ( -10.81309686280113525, 19.72027827561758428, -22.58649785105329499 ) ) ;
#31318=CARTESIAN_POINT ( 'NONE',  ( -15.34191545795870404, -23.11243443870917602, -15.23041013548281697 ) ) ;
#31321=CARTESIAN_POINT ( 'NONE',  ( -20.55867917417221591, -5.738195990446767425, -25.72316019435383438 ) ) ;
#31322=CARTESIAN_POINT ( 'NONE',  ( -14.71730574774288058, -25.79995879924697633, -9.711345329922794534 ) ) ;
#31325=CARTESIAN_POINT ( 'NONE',  ( 30.52654454056548872, 0.1756249017533851042, -6.888467937754702675 ) ) ;
#31329=CARTESIAN_POINT ( 'NONE',  ( -29.38226363743932978, 0.04289305711785689618, -10.65132950999735151 ) ) ;
#31331=CARTESIAN_POINT ( 'NONE',  ( 27.98788956557562813, -1.032887576452447886, -14.33963790881665368 ) ) ;
#31338=CARTESIAN_POINT ( 'NONE',  ( -26.32076408150614455, 4.396639818092925367, -9.315417411894323152 ) ) ;
#31348=CARTESIAN_POINT ( 'NONE',  ( -24.48289593984599932, 7.070685527441074925, -8.868132332187178335 ) ) ;
#31350=CARTESIAN_POINT ( 'NONE',  ( 22.28594499719783784, -24.59284248905922254, -11.20638719456909804 ) ) ;
#31352=CARTESIAN_POINT ( 'NONE',  ( 12.77624441107838038, 21.90293805066523092, -17.40359543253437380 ) ) ;
#31355=CARTESIAN_POINT ( 'NONE',  ( -15.51521182627543105, 23.67341184179000990, -10.21785028279580310 ) ) ;
#31361=CARTESIAN_POINT ( 'NONE',  ( 15.43643446434663069, 26.70998168114506299, -5.474185214589514459 ) ) ;
#31363=CARTESIAN_POINT ( 'NONE',  ( 19.48557158514982746, -11.25000000000009415, 3.000000000000000000 ) ) ;
#31365=CARTESIAN_POINT ( 'NONE',  ( -11.00725108063220681, 17.69432998924965261, -26.81932462650155102 ) ) ;
#31367=CARTESIAN_POINT ( 'NONE',  ( -15.57539791909990257, -26.68962352245197778, -6.414612666884428549 ) ) ;
#31371=CARTESIAN_POINT ( 'NONE',  ( -33.62363858789468196, -16.31856935978158418, -8.408815523728231156 ) ) ;
#31372=CARTESIAN_POINT ( 'NONE',  ( -14.18466236126857716, -26.34951843640821423, -6.418711051328147121 ) ) ;
#31374=CARTESIAN_POINT ( 'NONE',  ( 14.35173073918922704, 19.39993939583603222, -17.65283020193257002 ) ) ;
#31376=CARTESIAN_POINT ( 'NONE',  ( 24.13344123527126683, 5.447041238337571478, -13.77537616045479574 ) ) ;
#31381=CARTESIAN_POINT ( 'NONE',  ( -21.77226783765452822, 0.3831960823903834967, -23.81190093888698556 ) ) ;
#31382=CARTESIAN_POINT ( 'NONE',  ( 20.53334354118885585, 0.7178733630065357030, -28.70205288258643250 ) ) ;
#31387=CARTESIAN_POINT ( 'NONE',  ( -3.859759734048395785E-14, -22.74351282448223799, -30.00000000000000355 ) ) ;
#31396=CARTESIAN_POINT ( 'NONE',  ( 1.491327628155283636, 21.09632261899129801, -26.26494682969926941 ) ) ;
#31403=CARTESIAN_POINT ( 'NONE',  ( 14.96927680770918911, 27.53662669054819290, -7.330861191698205381 ) ) ;
#31406=CARTESIAN_POINT ( 'NONE',  ( -18.27253818691323062, 18.69021931283398530, -5.000000000000000000 ) ) ;
#31411=CARTESIAN_POINT ( 'NONE',  ( 15.31235917916896128, -26.57453613593431285, -6.888046241755874100 ) ) ;
#31413=CARTESIAN_POINT ( 'NONE',  ( -13.16997831943846364, -17.85564823066885154, -23.48525575126764764 ) ) ;
#31414=CARTESIAN_POINT ( 'NONE',  ( 15.23754071310550096, 26.38830581798780983, -7.827869159341425132 ) ) ;
#31415=CARTESIAN_POINT ( 'NONE',  ( 11.10861966544563728, 17.62435334769741857, -26.82886945948915525 ) ) ;
#31419=CARTESIAN_POINT ( 'NONE',  ( -14.24588017709789156, -25.05103694589206142, -11.60217997011687530 ) ) ;
#31422=CARTESIAN_POINT ( 'NONE',  ( -27.56419008223693368, -20.32132774350781546, -11.98953026114993214 ) ) ;
#31423=CARTESIAN_POINT ( 'NONE',  ( -4.514867549693919457, -24.02565271312832351, -11.85143917347367370 ) ) ;
#31424=CARTESIAN_POINT ( 'NONE',  ( 15.67016653301135243, 25.89419373281741343, -4.999999999999999112 ) ) ;
#31426=CARTESIAN_POINT ( 'NONE',  ( 18.71476311508316925, 8.734133638284580670, -27.16947995569030283 ) ) ;
#31430=CARTESIAN_POINT ( 'NONE',  ( -20.35866630304074221, -2.409458700188494618, -30.00000000000000000 ) ) ;
#31436=CARTESIAN_POINT ( 'NONE',  ( -29.53879188788242516, 0.8751376573578146800, -8.306695801703410709 ) ) ;
#31438=CARTESIAN_POINT ( 'NONE',  ( 34.91094743763966335, -15.30826278171658927, -5.859126002197243110 ) ) ;
#31443=B_SPLINE_CURVE_WITH_KNOTS ( 'NONE', 3,
 ( #26539, #2161, #35883, #33251 ),
 .UNSPECIFIED., .F., .F.,
 ( 4, 4 ),
 ( 0.000000000000000000, 1.000000000000000000 ),
 .UNSPECIFIED. ) ;
#31449=CARTESIAN_POINT ( 'NONE',  ( -2.937369183556012509, 36.26184006374910496, -9.732975961863635561 ) ) ;
#31455=CARTESIAN_POINT ( 'NONE',  ( 13.49628937919752936, 30.16421895756228011, -8.163569957728929793 ) ) ;
#31456=AXIS2_PLACEMENT_3D ( 'NONE', #31846, #6651, #19059 ) ;
#31458=CARTESIAN_POINT ( 'NONE',  ( -18.27861351387878486, 9.971955297741459390, -25.50930699828377257 ) ) ;
#31460=CARTESIAN_POINT ( 'NONE',  ( 9.732651874096569955, -18.42127846640838484, -26.82682959031351189 ) ) ;
#31462=CARTESIAN_POINT ( 'NONE',  ( 15.34082215761350731, 26.78240229728934807, -6.415436508019739748 ) ) ;
#31464=CARTESIAN_POINT ( 'NONE',  ( -31.47283671532261806, -25.12609584734821766, -14.45070082761205477 ) ) ;
#31466=EDGE_CURVE ( 'NONE', #18645, #32074, #21060, .T. ) ;
#31467=CARTESIAN_POINT ( 'NONE',  ( -22.06585941720839017, -22.05058654489405967, -13.92938651405431649 ) ) ;
#31468=CARTESIAN_POINT ( 'NONE',  ( 10.76261159742561802, -25.66954346325781700, -5.474903014184794969 ) ) ;
#31469=CARTESIAN_POINT ( 'NONE',  ( 15.18929233869975803, 25.85343093234575562, -8.770441219456733606 ) ) ;
#31470=CARTESIAN_POINT ( 'NONE',  ( 29.20799977545595638, -19.79325530109120379, -11.07381889372395456 ) ) ;
#31474=CARTESIAN_POINT ( 'NONE',  ( -5.905911943458037605, 19.71813378021714769, -28.52406569151924742 ) ) ;
#31479=CARTESIAN_POINT ( 'NONE',  ( 30.94149296799522020, -0.08026563842153495998, -4.999999999999999112 ) ) ;
#31482=ORIENTED_EDGE ( 'NONE', *, *, #3827, .T. ) ;
#31484=CARTESIAN_POINT ( 'NONE',  ( -28.84883529782520384, 0.1510037028947092130, -11.60082923936701782 ) ) ;
#31485=CARTESIAN_POINT ( 'NONE',  ( -18.54826650170510760, -24.72227203249315863, -12.26027862771963228 ) ) ;
#31488=CARTESIAN_POINT ( 'NONE',  ( 20.61284349087890178, -4.224483801661988558, -26.46532051397237595 ) ) ;
#31497=EDGE_CURVE ( 'NONE', #6388, #648, #26879, .T. ) ;
#31501=CARTESIAN_POINT ( 'NONE',  ( -18.94584503392242425, -7.857761768003762803, -30.00000000000000000 ) ) ;
#31504=CARTESIAN_POINT ( 'NONE',  ( 14.00978157989841932, 15.66612192722645780, -25.31855382825745693 ) ) ;
#31505=CARTESIAN_POINT ( 'NONE',  ( 5.567050714568646974, 24.71546371777111517, -19.77525644353581669 ) ) ;
#31507=CARTESIAN_POINT ( 'NONE',  ( 14.98429054056425791, -24.74230029465469372, -12.47804673543034681 ) ) ;
#31514=CARTESIAN_POINT ( 'NONE',  ( -11.32195743957676726, 18.02873052150704325, -25.01618100487094409 ) ) ;
#31517=CARTESIAN_POINT ( 'NONE',  ( 15.03800791059918396, -26.62802654356141119, -5.000000000000000888 ) ) ;
#31521=CARTESIAN_POINT ( 'NONE',  ( -9.991501677813444005, 23.11176406337531120, -19.09605641320739267 ) ) ;
#31524=CARTESIAN_POINT ( 'NONE',  ( -34.93438416866315066, -9.757236910605460167, -7.597984259234436877 ) ) ;
#31525=CARTESIAN_POINT ( 'NONE',  ( -9.861416007139599316, -18.85607788447654443, -25.02649126457271223 ) ) ;
#31528=CARTESIAN_POINT ( 'NONE',  ( 28.14739292305172924, 0.3821647062335758460, -12.56146095346657532 ) ) ;
#31532=CARTESIAN_POINT ( 'NONE',  ( -23.95715816398616127, 0.4476729911382093530, -19.49109017648843789 ) ) ;
#31534=CARTESIAN_POINT ( 'NONE',  ( 20.50115022911059270, -0.2752137519716085223, -29.32748844547824163 ) ) ;
#31547=CARTESIAN_POINT ( 'NONE',  ( -22.69387413952485488, 8.732923056282277940, -11.85621800793260405 ) ) ;
#31548=CARTESIAN_POINT ( 'NONE',  ( 21.16136169972589443, -23.36689248179594713, -13.05645000173869441 ) ) ;
#31550=CARTESIAN_POINT ( 'NONE',  ( 12.85423046086276777, 21.77606881879581024, -17.42081002309879167 ) ) ;
#31552=CARTESIAN_POINT ( 'NONE',  ( -15.50946703677032268, 25.48995504883554375, -7.833083979528388419 ) ) ;
#31555=CARTESIAN_POINT ( 'NONE',  ( 12.67586314470820419, 21.02061172028682989, -18.45614634320944702 ) ) ;
#31560=CARTESIAN_POINT ( 'NONE',  ( -15.28843509798326750, 26.96128135507572310, -6.412575688757890191 ) ) ;
#31562=CARTESIAN_POINT ( 'NONE',  ( -15.97359574264618409, -26.56429016778576369, -7.804459717415208608 ) ) ;
#31566=CARTESIAN_POINT ( 'NONE',  ( -20.21266914523116043, -10.59870367858544071, -22.98988714542691625 ) ) ;
#31567=CARTESIAN_POINT ( 'NONE',  ( -8.977629974610007224, -18.64362841147424632, -27.49153544992771359 ) ) ;
#31569=CARTESIAN_POINT ( 'NONE',  ( 15.70302840757942953, 22.76320954772178240, -10.71404650329602326 ) ) ;
#31571=CARTESIAN_POINT ( 'NONE',  ( 19.71254563347552846, 5.914222174241564822, -28.25527075934179067 ) ) ;
#31574=CARTESIAN_POINT ( 'NONE',  ( -13.16997832219843545, -17.85564823411818836, -23.48525574308021646 ) ) ;
#31576=CARTESIAN_POINT ( 'NONE',  ( -31.07115740369864199, -0.3229936248456179992, -6.410853627256240195 ) ) ;
#31577=CARTESIAN_POINT ( 'NONE',  ( 27.38313135976468260, -0.1050505738281504176, -14.43771228336784063 ) ) ;
#31580=CARTESIAN_POINT ( 'NONE',  ( 13.28992586503610163, -18.25382200079949513, -20.55760979252977094 ) ) ;
#31584=CARTESIAN_POINT ( 'NONE',  ( -5.049784273262889478, -26.77689918168220018, -5.000000000000000888 ) ) ;
#31588=CARTESIAN_POINT ( 'NONE',  ( 2.668841116913945211, 20.33496311051875693, -30.00000000000001066 ) ) ;
#31589=FACE_OUTER_BOUND ( 'NONE', #32372, .T. ) ;
#31596=CARTESIAN_POINT ( 'NONE',  ( 15.03773630625828517, 27.03340586037365867, -7.807355954524350494 ) ) ;
#31600=CARTESIAN_POINT ( 'NONE',  ( -17.24705954285015963, 17.28840653234623659, -13.80911451859712358 ) ) ;
#31604=CARTESIAN_POINT ( 'NONE',  ( 13.70278808041313034, -24.11633286913983909, -13.51357506480354154 ) ) ;
#31606=CARTESIAN_POINT ( 'NONE',  ( 14.53734341128950014, 24.95703585460324803, -11.59938498087787195 ) ) ;
#31608=CARTESIAN_POINT ( 'NONE',  ( 12.12399539440989393, 19.93227742869169816, -20.53953816727202408 ) ) ;
#31612=CARTESIAN_POINT ( 'NONE',  ( -9.739536567210267393, -18.58453973594571451, -26.22921015961444979 ) ) ;
#31614=CARTESIAN_POINT ( 'NONE',  ( -30.65860538206566588, -22.55701637896913070, -6.281012731829498819 ) ) ;
#31615=CARTESIAN_POINT ( 'NONE',  ( -3.609577435699458547, -21.27339400844680384, -22.19980166077412065 ) ) ;
#31616=CARTESIAN_POINT ( 'NONE',  ( 11.46030064407786675, 17.14133356389085350, -28.10178865267953441 ) ) ;
#31617=EDGE_CURVE ( 'NONE', #19220, #14160, #12068, .T. ) ;
#31619=CARTESIAN_POINT ( 'NONE',  ( 22.50594045486629469, 10.05894777106499838, -8.895335536218450301 ) ) ;
#31625=CARTESIAN_POINT ( 'NONE',  ( -27.32938361780223957, -2.673874545957628079, -16.12352731284545726 ) ) ;
#31631=FACE_OUTER_BOUND ( 'NONE', #35211, .T. ) ;
#31633=CARTESIAN_POINT ( 'NONE',  ( -28.60302894850194022, 1.758667520871832757, -8.791322179575384865 ) ) ;
#31634=CARTESIAN_POINT ( 'NONE',  ( 20.37979243436083010, -8.235259509822993707, -24.27245371426751674 ) ) ;
#31637=ORIENTED_EDGE ( 'NONE', *, *, #25378, .F. ) ;
#31640=EDGE_CURVE ( 'NONE', #39512, #1450, #37882, .T. ) ;
#31642=CARTESIAN_POINT ( 'NONE',  ( -15.42150907995254983, 26.76352410258160930, -5.000000000000001776 ) ) ;
#31645=CARTESIAN_POINT ( 'NONE',  ( -1.130164101217176365, 22.80556646834144630, -22.98960577978414577 ) ) ;
#31654=CARTESIAN_POINT ( 'NONE',  ( 8.928096088923819451, 19.18392227192688182, -25.99240570989386256 ) ) ;
#31658=CARTESIAN_POINT ( 'NONE',  ( -19.04214505569463967, 11.35732863687608152, -19.06679702495384277 ) ) ;
#31661=CARTESIAN_POINT ( 'NONE',  ( 15.49155713431803960, -26.66867858187293550, -6.415952216431528576 ) ) ;
#31663=CARTESIAN_POINT ( 'NONE',  ( 11.13181036404293067, 17.79423202622817968, -26.21918479596937601 ) ) ;
#31664=CARTESIAN_POINT ( 'NONE',  ( 13.28992586503610163, -18.25382200079949513, -20.55760979252977094 ) ) ;
#31667=CARTESIAN_POINT ( 'NONE',  ( -21.80867257259097514, -23.11172725429855390, -13.03247554641362349 ) ) ;
#31668=CARTESIAN_POINT ( 'NONE',  ( 8.497644768481743327, -25.32189558139016228, -5.000000000000002665 ) ) ;
#31669=CARTESIAN_POINT ( 'NONE',  ( 11.07485645340150171, 17.25102576792224340, -29.99999999999999289 ) ) ;
#31670=CARTESIAN_POINT ( 'NONE',  ( 25.87580467091643399, -17.52732614752431672, -14.74065523776432052 ) ) ;
#31674=CARTESIAN_POINT ( 'NONE',  ( -6.253143773029494312, 26.59490657384560208, -17.73706128625773459 ) ) ;
#31677=CARTESIAN_POINT ( 'NONE',  ( 30.92038317698504457, -0.05869178374276579069, -5.000000000000000000 ) ) ;
#31681=CARTESIAN_POINT ( 'NONE',  ( -20.68821937854897541, 0.9221346313300146091, -27.45318776198465471 ) ) ;
#31684=CARTESIAN_POINT ( 'NONE',  ( 33.80886038580988640, -8.069990905591543751, -9.383811014428410147 ) ) ;
#31698=CARTESIAN_POINT ( 'NONE',  ( 6.245935934162172742, 19.56982954529273400, -30.00000000000000711 ) ) ;
#31701=CARTESIAN_POINT ( 'NONE',  ( 13.75357712579410574, 15.21937127477098350, -30.00000000000000711 ) ) ;
#31702=CARTESIAN_POINT ( 'NONE',  ( 10.02000509642858361, 34.97447782610390732, -4.999999999999999112 ) ) ;
#31704=CARTESIAN_POINT ( 'NONE',  ( 15.84394465367380178, -26.31127309132897452, -8.735524027787771928 ) ) ;
#31710=CARTESIAN_POINT ( 'NONE',  ( -13.21411722169975711, 22.22692963839663705, -16.44518550108498189 ) ) ;
#31713=CARTESIAN_POINT ( 'NONE',  ( 10.26885880249883165, -19.65294855164837884, -22.76732940879269051 ) ) ;
#31719=CARTESIAN_POINT ( 'NONE',  ( -12.40929423282409694, 26.94941001123947544, -13.25802102404320060 ) ) ;
#31720=CARTESIAN_POINT ( 'NONE',  ( -75.15099915297791711, 43.38844959084113384, 0.000000000000000000 ) ) ;
#31723=CARTESIAN_POINT ( 'NONE',  ( -33.27180366187747751, -8.208870852378092664, -10.27506301637745167 ) ) ;
#31725=ORIENTED_EDGE ( 'NONE', *, *, #35131, .F. ) ;
#31726=CARTESIAN_POINT ( 'NONE',  ( 30.75747790117273794, 0.1077116562829361218, -4.999999999999999112 ) ) ;
#31729=ORIENTED_EDGE ( 'NONE', *, *, #3997, .F. ) ;
#31730=CARTESIAN_POINT ( 'NONE',  ( -30.20906327819625048, -0.01427245983082933191, -8.766269380263043587 ) ) ;
#31731=CARTESIAN_POINT ( 'NONE',  ( 75.15099915297797395, 43.38844959084117647, -5.000000000000000000 ) ) ;
#31733=CARTESIAN_POINT ( 'NONE',  ( 32.71662871600790368, -3.117337333226495755, -8.171977234651780719 ) ) ;
#31751=CARTESIAN_POINT ( 'NONE',  ( -21.91354840350972211, 9.539350162456797122, -12.87506386756524179 ) ) ;
#31752=CARTESIAN_POINT ( 'NONE',  ( 15.40455633798288204, -19.17866944239923299, -20.04336763641729036 ) ) ;
#31755=CARTESIAN_POINT ( 'NONE',  ( 14.45110082695830833, 25.20033142108280089, -11.58180078429156090 ) ) ;
#31757=CARTESIAN_POINT ( 'NONE',  ( -15.85862229823199776, 25.25472105652747246, -5.000000000000000000 ) ) ;
#31761=CARTESIAN_POINT ( 'NONE',  ( 12.68336450221132417, 21.00970290476725211, -18.45743704410757857 ) ) ;
#31763=CARTESIAN_POINT ( 'NONE',  ( 22.90052353346136371, -11.74428243424502760, -19.63336109330355228 ) ) ;
#31766=CARTESIAN_POINT ( 'NONE',  ( -14.75109696978639029, 26.35784808731213857, -9.678683898009220243 ) ) ;
#31768=CARTESIAN_POINT ( 'NONE',  ( -15.44690521824878537, -25.79975055938752604, -10.14031905184057791 ) ) ;
#31772=CARTESIAN_POINT ( 'NONE',  ( -34.54285066864272835, -16.78341526201209533, -5.435878295993979314 ) ) ;
#31773=CARTESIAN_POINT ( 'NONE',  ( -10.69804542477608855, -21.08478606119448884, -19.58466021002672974 ) ) ;
#31775=CARTESIAN_POINT ( 'NONE',  ( 15.90807616341559338, 22.25326793540537906, -10.72615760417953013 ) ) ;
#31777=CARTESIAN_POINT ( 'NONE',  ( 26.66934055787902835, 2.909074036114203121, -11.70011843583559497 ) ) ;
#31779=LINE ( 'NONE', #22420, #6302 ) ;
#31782=CARTESIAN_POINT ( 'NONE',  ( -20.50193171233730993, 0.1922071591807814339, -29.33613531814199149 ) ) ;
#31783=CARTESIAN_POINT ( 'NONE',  ( 20.99165470567395175, 0.5836903346832758022, -26.20505728122213895 ) ) ;
#31785=VERTEX_POINT ( 'NONE', #21451 ) ;
#31786=CARTESIAN_POINT ( 'NONE',  ( -12.33616729053609795, -27.99489201236593061, -4.999999999999999112 ) ) ;
#31788=VERTEX_POINT ( 'NONE', #6005 ) ;
#31797=CARTESIAN_POINT ( 'NONE',  ( 26.92080679176510571, -24.85520046368381131, -7.585400692263990940 ) ) ;
#31801=CARTESIAN_POINT ( 'NONE',  ( 10.55968626961773360, 17.57118088696260827, -29.33920240098544951 ) ) ;
#31804=CARTESIAN_POINT ( 'NONE',  ( -17.73668911492254807, 19.59045636488301767, -7.397010546184955793 ) ) ;
#31807=CARTESIAN_POINT ( 'NONE',  ( 15.41329945644580413, -26.72332452139117720, -5.000000000000000000 ) ) ;
#31809=CARTESIAN_POINT ( 'NONE',  ( 11.07256710390407051, 17.50279746095970523, -27.44776494551608792 ) ) ;
#31811=CARTESIAN_POINT ( 'NONE',  ( 14.73787879266534873, 25.39503920881744392, -10.65324680268567725 ) ) ;
#31813=CARTESIAN_POINT ( 'NONE',  ( -11.43760958252774884, 18.47761077602904223, -23.84654567625729626 ) ) ;
#31815=CARTESIAN_POINT ( 'NONE',  ( -12.97980758920870592, -23.09007905854067744, -15.45264339162509515 ) ) ;
#31818=CARTESIAN_POINT ( 'NONE',  ( -18.79189612092352135, -12.94303005244327132, -23.00170733529830258 ) ) ;
#31819=CARTESIAN_POINT ( 'NONE',  ( -1.766708854211077595, -20.47917438257665879, -30.00000000000000355 ) ) ;
#31820=CARTESIAN_POINT ( 'NONE',  ( 13.81705425458364722, 22.18564081078588046, -15.49648774365130244 ) ) ;
#31822=CARTESIAN_POINT ( 'NONE',  ( 18.53824370654135478, 9.487311751210160793, -25.50586965412942320 ) ) ;
#31826=CARTESIAN_POINT ( 'NONE',  ( -20.28315073442723460, -3.046437751679770933, -30.00000000000000000 ) ) ;
#31833=CARTESIAN_POINT ( 'NONE',  ( 34.73373506214407769, -15.22407143656519679, -6.703790208019304586 ) ) ;
#31839=CARTESIAN_POINT ( 'NONE',  ( -15.41558956984166251, 26.78481017248024898, -5.000000000000000000 ) ) ;
#31844=CARTESIAN_POINT ( 'NONE',  ( -1.517615944522816118, 30.16442793585677862, -15.68169713778068441 ) ) ;
#31846=CARTESIAN_POINT ( 'NONE',  ( -1.829593030691901284E-15, 22.50000000000001066, -5.000000000000000000 ) ) ;
#31852=CARTESIAN_POINT ( 'NONE',  ( 9.367770739272080149, 18.53333684161963646, -27.31848943577234934 ) ) ;
#31854=VERTEX_POINT ( 'NONE', #31989 ) ;
#31855=CARTESIAN_POINT ( 'NONE',  ( -18.38058839721481874, 11.97145855736538245, -20.11878731179081825 ) ) ;
#31858=CARTESIAN_POINT ( 'NONE',  ( 13.42465078840814918, -23.62789290738457382, -14.47165382363914787 ) ) ;
#31860=CARTESIAN_POINT ( 'NONE',  ( 10.94214493613176664, 17.33550160327741096, -29.99999999999999289 ) ) ;
#31861=CARTESIAN_POINT ( 'NONE',  ( -13.47223693944937040, 18.09844039693852125, -29.99999999999999645 ) ) ;
#31863=CARTESIAN_POINT ( 'NONE',  ( -22.97994382251033585, -24.34209009305979166, -11.18594617276381697 ) ) ;
#31864=CARTESIAN_POINT ( 'NONE',  ( 8.487318810465147578, -25.30172221365172192, -5.955506841159929010 ) ) ;
#31865=CARTESIAN_POINT ( 'NONE',  ( 11.26119111163083630, 17.51761337186505685, -26.84302999491309194 ) ) ;
#31866=CARTESIAN_POINT ( 'NONE',  ( 30.53998965538356103, -22.06133822602150474, -7.552213228032163883 ) ) ;
#31873=CARTESIAN_POINT ( 'NONE',  ( -5.884614315209530488, 19.64670892508010169, -29.99999999999997868 ) ) ;
#31877=CARTESIAN_POINT ( 'NONE',  ( 22.74115952922136330, 0.5763562226926195464, -21.61272164397127682 ) ) ;
#31882=CARTESIAN_POINT ( 'NONE',  ( -29.50026895737458688, 0.1576476882857581474, -10.18295560989503734 ) ) ;
#31885=CARTESIAN_POINT ( 'NONE',  ( 35.30405009085131240, -9.553221813830631959, -6.305931249553304418 ) ) ;
#31895=CARTESIAN_POINT ( 'NONE',  ( -4.448583892168122667, 20.01379199642233075, -29.99999999999998579 ) ) ;
#31898=CARTESIAN_POINT ( 'NONE',  ( 18.12927444247487685, 18.97622154095044777, -5.957654057152589999 ) ) ;
#31899=CARTESIAN_POINT ( 'NONE',  ( 5.857883788898597288, 20.22416296293512872, -26.42044690542252638 ) ) ;
#31903=CARTESIAN_POINT ( 'NONE',  ( 16.28181498793477999, -26.61367711139261161, -7.795649509280883294 ) ) ;
#31907=CARTESIAN_POINT ( 'NONE',  ( -15.29470497349542235, 26.51477255901613361, -7.358185202849431228 ) ) ;
#31909=CARTESIAN_POINT ( 'NONE',  ( 9.392528018862558170, -18.45111944239248913, -27.46388755805442372 ) ) ;
#31915=CARTESIAN_POINT ( 'NONE',  ( -12.65601555930210509, 32.35306062433939900, -5.452413821557709817 ) ) ;
#31918=CARTESIAN_POINT ( 'NONE',  ( -30.08318636280791125, -7.404603725954973292, -13.95201704139118526 ) ) ;
#31921=CARTESIAN_POINT ( 'NONE',  ( 30.04993021256226626, 0.1566486852560641796, -8.769524174311651876 ) ) ;
#31925=CARTESIAN_POINT ( 'NONE',  ( -21.71042592863056342, 0.7213194707694018382, -23.85327911821731206 ) ) ;
#31928=CARTESIAN_POINT ( 'NONE',  ( 33.32260079917540452, -3.210191908071163169, -5.911986766794023573 ) ) ;
#31932=VERTEX_POINT ( 'NONE', #16764 ) ;
#31945=CARTESIAN_POINT ( 'NONE',  ( -19.39911238771444246, 7.131629512367122281, -27.14147998049999444 ) ) ;
#31946=CARTESIAN_POINT ( 'NONE',  ( 21.24144353091755733, -26.22539287217877657, -9.006437966444934773 ) ) ;
#31948=VERTEX_POINT ( 'NONE', #14665 ) ;
#31949=CARTESIAN_POINT ( 'NONE',  ( 11.17207643027059305, 18.14497318590918695, -24.99559416334685835 ) ) ;
#31951=CARTESIAN_POINT ( 'NONE',  ( -14.10408248735370407, 22.68866825637624274, -14.51867820061998060 ) ) ;
#31954=CARTESIAN_POINT ( 'NONE',  ( 11.22661243547084453, 17.72572647685119307, -26.22939125915132053 ) ) ;
#31955=ORIENTED_EDGE ( 'NONE', *, *, #12343, .F. ) ;
#31956=CARTESIAN_POINT ( 'NONE',  ( 29.30039860399171303, -16.15247984952398141, -12.89021756677838226 ) ) ;
#31960=CARTESIAN_POINT ( 'NONE',  ( -10.79835490039502410, 17.42544872524608479, -29.99999999999999289 ) ) ;
#31963=CARTESIAN_POINT ( 'NONE',  ( -12.44748226125696711, -21.44593556856202810, -18.38580773262598456 ) ) ;
#31968=CARTESIAN_POINT ( 'NONE',  ( -26.66261548401102743, -11.00715225274686482, -16.66819200665372946 ) ) ;
#31969=CARTESIAN_POINT ( 'NONE',  ( -14.06843317319044928, -25.79384935331063744, -9.249739353774602435 ) ) ;
#31971=CARTESIAN_POINT ( 'NONE',  ( 14.59202647793683738, 19.84686743550333432, -16.64054136931479633 ) ) ;
#31973=CARTESIAN_POINT ( 'NONE',  ( 25.22259539243878024, 3.759474034095959372, -13.70306588605936327 ) ) ;
#31974=DIRECTION ( 'NONE',  ( -1.000000000000000000, 0.000000000000000000, 0.000000000000000000 ) ) ;
#31978=CARTESIAN_POINT ( 'NONE',  ( -21.31112166252114903, 0.5185946039941641272, -24.98634476583432829 ) ) ;
#31979=CARTESIAN_POINT ( 'NONE',  ( 21.33889498998111378, 0.2955338563558915776, -24.96187165485871162 ) ) ;
#31982=CARTESIAN_POINT ( 'NONE',  ( -26.31271763591399804, -28.25584584496044727, -14.26382729546507555 ) ) ;
#31989=CARTESIAN_POINT ( 'NONE',  ( -15.48853125999098701, -26.74269726803709446, 0.000000000000000000 ) ) ;
#31999=CARTESIAN_POINT ( 'NONE',  ( 15.55596413789349342, -13.49028823909393893, -28.47924180414970863 ) ) ;
#32002=CARTESIAN_POINT ( 'NONE',  ( 15.14367636855533483, 27.25780052973253476, -6.874303053600053559 ) ) ;
#32006=CARTESIAN_POINT ( 'NONE',  ( -17.83076603928403969, 19.73132804355285685, -4.999999999999999112 ) ) ;
#32008=CARTESIAN_POINT ( 'NONE',  ( 14.02069553749537789, -24.60808805636505880, -12.55129267140057081 ) ) ;
#32010=CARTESIAN_POINT ( 'NONE',  ( 14.03024999042850496, 23.93342408826297074, -13.51346792333798241 ) ) ;
#32012=CARTESIAN_POINT ( 'NONE',  ( 10.99616811907620395, 17.35450030463652737, -28.70654324492396725 ) ) ;
#32014=CARTESIAN_POINT ( 'NONE',  ( -12.60536492748955517, 21.12509647135009772, -18.44162819889032789 ) ) ;
#32016=CARTESIAN_POINT ( 'NONE',  ( -14.34991748541630230, -25.06893485500494378, -11.59976961054102240 ) ) ;
#32020=CARTESIAN_POINT ( 'NONE',  ( -19.17385361915705033, -12.37337734071081563, -22.99238475705470819 ) ) ;
#32022=CARTESIAN_POINT ( 'NONE',  ( -7.043788095933357418, -25.16102598387571376, -5.958356067281301627 ) ) ;
#32023=CARTESIAN_POINT ( 'NONE',  ( 15.68203584040330334, 25.45105541600625187, -6.890715696209627872 ) ) ;
#32025=CARTESIAN_POINT ( 'NONE',  ( 23.69351461785554136, 8.239566554881321281, -8.880179489987360952 ) ) ;
#32026=CARTESIAN_POINT ( 'NONE',  ( 27.27781358227127129, -25.27706179178272450, -4.999999999999999112 ) ) ;
#32030=CARTESIAN_POINT ( 'NONE',  ( -33.19333159104881048, -3.445792630615724050, -7.261352220591662743 ) ) ;
#32035=CARTESIAN_POINT ( 'NONE',  ( 33.73785410275350216, -15.99653540799024931, -8.410072970351906818 ) ) ;
#32040=VERTEX_POINT ( 'NONE', #39639 ) ;
#32042=CARTESIAN_POINT ( 'NONE',  ( -24.10033869720827227, 8.113510326755614344, -5.000000000000002665 ) ) ;
#32043=CARTESIAN_POINT ( 'NONE',  ( 19.48557158514988075, -11.24999999999998224, 0.000000000000000000 ) ) ;
#32046=CARTESIAN_POINT ( 'NONE',  ( -0.3989805618741724125, 20.59240739012455990, -28.44384999149225379 ) ) ;
#32049=CARTESIAN_POINT ( 'NONE',  ( 17.00000000000000000, 22.50000000000000711, 10.00000000000000000 ) ) ;
#32052=CARTESIAN_POINT ( 'NONE',  ( 9.263407132367138530, 18.28842304576874156, -29.31195371305176067 ) ) ;
#32054=ORIENTED_EDGE ( 'NONE', *, *, #38076, .F. ) ;
#32055=CARTESIAN_POINT ( 'NONE',  ( -19.69150485828470920, 15.64879689043717192, -4.999999999999998224 ) ) ;
#32059=CARTESIAN_POINT ( 'NONE',  ( 15.45120705166009678, -26.60939779128311500, -6.886503721798920452 ) ) ;
#32061=CARTESIAN_POINT ( 'NONE',  ( 11.28132746819896504, 18.06042462519475933, -25.01062990606723346 ) ) ;
#32062=CARTESIAN_POINT ( 'NONE',  ( -22.45323650136969462, -2.382502413133420038, -20.55760979252980647 ) ) ;
#32065=CARTESIAN_POINT ( 'NONE',  ( -14.31376830907703557, -15.17370222568340488, -27.11184809475398438 ) ) ;
#32066=CARTESIAN_POINT ( 'NONE',  ( 5.958427663799773732, -24.34613153426185761, -10.83339736943976028 ) ) ;
#32067=CARTESIAN_POINT ( 'NONE',  ( 13.29387873628312633, 22.08577950255929778, -16.45709539392367660 ) ) ;
#32068=CARTESIAN_POINT ( 'NONE',  ( 20.55850455995617310, 13.96709772207984557, -5.966656640325017413 ) ) ;
#32073=CARTESIAN_POINT ( 'NONE',  ( -9.173595147271331740, 34.50490541566588121, -8.476194683046836431 ) ) ;
#32074=VERTEX_POINT ( 'NONE', #9168 ) ;
#32078=CARTESIAN_POINT ( 'NONE',  ( 30.38638613626090645, -0.03985804923669677979, -8.295769245405898218 ) ) ;
#32084=CARTESIAN_POINT ( 'NONE',  ( -20.60809083734462277, 0.8890292739548594225, -28.07942971103104313 ) ) ;
#32085=CARTESIAN_POINT ( 'NONE',  ( -20.54949622337250403, -27.17849093743868849, -5.904791858790468417 ) ) ;
#32087=CARTESIAN_POINT ( 'NONE',  ( 25.26093265137713573, -6.803277765801289512, -18.80458527437446747 ) ) ;
#32099=CARTESIAN_POINT ( 'NONE',  ( -15.31690239355500971, 13.64047066522845242, -30.00000000000001776 ) ) ;
#32103=CARTESIAN_POINT ( 'NONE',  ( 15.80069108502425301, 17.14170230956324303, -17.82616030926931927 ) ) ;
#32104=CARTESIAN_POINT ( 'NONE',  ( 5.706445963761893836, 19.68930810918331531, -29.25141939363317078 ) ) ;
#32108=CARTESIAN_POINT ( 'NONE',  ( 9.965926242692308534, -17.97018614680934689, -28.68921181318054892 ) ) ;
#32112=AXIS2_PLACEMENT_3D ( 'NONE', #15377, #18633, #40156 ) ;
#32114=CARTESIAN_POINT ( 'NONE',  ( -14.94540916678409559, 25.76695089328861599, -9.709480485754761858 ) ) ;
#32116=CARTESIAN_POINT ( 'NONE',  ( 9.271440805881887570, -18.28379014461920349, -30.00000000000000000 ) ) ;
#32121=CARTESIAN_POINT ( 'NONE',  ( -10.24063254661171918, 21.86334665591954618, -20.21485189711300379 ) ) ;
#32126=CARTESIAN_POINT ( 'NONE',  ( -31.82304104356865793, -7.834543439184518121, -12.09424007204980711 ) ) ;
#32130=CARTESIAN_POINT ( 'NONE',  ( 30.52903303563438797, 0.07247293852937149172, -7.358272049610939725 ) ) ;
#32132=CARTESIAN_POINT ( 'NONE',  ( 11.05997879105324877, 17.47350834465349578, -27.43542404371585164 ) ) ;
#32136=CARTESIAN_POINT ( 'NONE',  ( -28.34239771388248030, 0.1355473793836993457, -12.55008231272072194 ) ) ;
#32139=CARTESIAN_POINT ( 'NONE',  ( 28.83559650784853545, -2.623511950590506014, -14.20132271218602149 ) ) ;
#32145=FACE_OUTER_BOUND ( 'NONE', #35434, .T. ) ;
#32149=EDGE_CURVE ( 'NONE', #6084, #2291, #15222, .T. ) ;
#32157=CARTESIAN_POINT ( 'NONE',  ( -23.57137302209975260, 8.956611734839530214, -5.963979942565353909 ) ) ;
#32158=CARTESIAN_POINT ( 'NONE',  ( 20.69337408919974663, -25.59025939823920481, -10.36400023151281324 ) ) ;
#32159=CARTESIAN_POINT ( 'NONE',  ( -24.54956740501959800, -26.55910502559106590, -5.000000000000000000 ) ) ;
#32161=CARTESIAN_POINT ( 'NONE',  ( 12.31018467675442096, 20.59829060042622828, -19.47928546867396093 ) ) ;
#32163=CARTESIAN_POINT ( 'NONE',  ( -15.63234325287015558, 24.80996185906289853, -8.309407532411428932 ) ) ;
#32166=CARTESIAN_POINT ( 'NONE',  ( 15.39960304625618726, 26.57504432316893883, -6.417109345100691975 ) ) ;
#32168=CARTESIAN_POINT ( 'NONE',  ( 32.80197066822268681, -18.08580508125842101, -8.405041325730369550 ) ) ;
#32171=CARTESIAN_POINT ( 'NONE',  ( -10.85232944982509373, 17.54704845259137969, -28.06621872721026278 ) ) ;
#32173=CARTESIAN_POINT ( 'NONE',  ( -14.44323513478368426, -23.70972000048200812, -14.37742332914230659 ) ) ;
#32177=CARTESIAN_POINT ( 'NONE',  ( -21.63092173904548332, -9.727850427649963549, -21.86719485504245952 ) ) ;
#32178=CARTESIAN_POINT ( 'NONE',  ( -9.124714416476436440, -18.84963008713028287, -26.28455564130669941 ) ) ;
#32180=CARTESIAN_POINT ( 'NONE',  ( 13.28607726706187364, 15.81902776886276385, -27.59724186177722416 ) ) ;
#32182=CARTESIAN_POINT ( 'NONE',  ( 27.65851975983521527, 2.896154268494189665, -8.808624792320287611 ) ) ;
#32186=EDGE_LOOP ( 'NONE', ( #12237, #10184 ) ) ;
#32187=CARTESIAN_POINT ( 'NONE',  ( -30.81597363132232914, -0.1242289339610933435, -6.885118092463035744 ) ) ;
#32188=CARTESIAN_POINT ( 'NONE',  ( 20.49250884496040115, 0.5553618484168656444, -29.34280755129132245 ) ) ;
#32194=CARTESIAN_POINT ( 'NONE',  ( 6.023418944065110914, 39.81932404830325112, -14.45070082761206365 ) ) ;
#32198=EDGE_CURVE ( 'NONE', #8093, #3398, #38562, .T. ) ;
#32200=CARTESIAN_POINT ( 'NONE',  ( 22.71238962388145310, 10.21442836349894456, -4.999999999999998224 ) ) ;
#32205=CARTESIAN_POINT ( 'NONE',  ( 26.77741691842820870, -24.73292702398819642, -8.017675451830744038 ) ) ;
#32208=CARTESIAN_POINT ( 'NONE',  ( 15.05466390046562886, 27.28512766916796295, -7.337438985496051558 ) ) ;
#32210=CARTESIAN_POINT ( 'NONE',  ( -14.00996106472373270, 15.24814236169682147, -27.05129743250489938 ) ) ;
#32214=CARTESIAN_POINT ( 'NONE',  ( 14.68419454952205072, -25.64123961583407763, -10.18168563382398162 ) ) ;
#32216=CARTESIAN_POINT ( 'NONE',  ( 15.37856327759776320, 26.64927617434213047, -6.417027871434891395 ) ) ;
#32218=CARTESIAN_POINT ( 'NONE',  ( 13.76661467574962394, 23.40248112065825836, -14.47560752045292709 ) ) ;
#32220=CARTESIAN_POINT ( 'NONE',  ( -14.99409613481703651, 26.04743989974285867, -9.234380414057861586 ) ) ;
#32222=CARTESIAN_POINT ( 'NONE',  ( -15.37461277948404614, -26.63904247529195146, -6.417043597033281088 ) ) ;
#32225=CARTESIAN_POINT ( 'NONE',  ( -21.60462512834099869, -13.94959705066216493, -19.63613014917582689 ) ) ;
#32226=CARTESIAN_POINT ( 'NONE',  ( -4.583136480692052039, -24.23512553185321750, -10.85810497518859030 ) ) ;
#32227=CARTESIAN_POINT ( 'NONE',  ( 13.66344759430295674, 21.43633434956417716, -16.51270124952114671 ) ) ;
#32230=CARTESIAN_POINT ( 'NONE',  ( 24.02933105728603991, 8.309275822838595005, -5.480673643475639345 ) ) ;
#32235=CARTESIAN_POINT ( 'NONE',  ( -28.11566308881036846, -1.264383335452437418, -14.31890013009667939 ) ) ;
#32237=EDGE_CURVE ( 'NONE', #23669, #1290, #23146, .T. ) ;
#32243=CARTESIAN_POINT ( 'NONE',  ( 24.46249166291341126, -10.72823817068293728, -18.64685341546218211 ) ) ;
#32249=CARTESIAN_POINT ( 'NONE',  ( -16.10728771989144903, 24.44770348874625299, -4.999999999999999112 ) ) ;
#32254=CARTESIAN_POINT ( 'NONE',  ( -1.915298613502000036, 38.17830312701165241, -6.697546018672553281 ) ) ;
#32260=CARTESIAN_POINT ( 'NONE',  ( 11.22822495210109395, 22.89591416269367841, -18.18872776029335014 ) ) ;
#32263=CARTESIAN_POINT ( 'NONE',  ( -17.49499888782854384, 11.31808902454676335, -25.50841800900462886 ) ) ;
#32266=CARTESIAN_POINT ( 'NONE',  ( 15.24043722059125017, -26.29847216020535683, -8.295283855862736644 ) ) ;
#32268=CARTESIAN_POINT ( 'NONE',  ( 12.62672847796949505, 21.09324721752569332, -18.44634832236629407 ) ) ;
#32269=CARTESIAN_POINT ( 'NONE',  ( -23.06249103411543544, 13.31513540672989926, -4.999999999999996447 ) ) ;
#32271=EDGE_CURVE ( 'NONE', #19280, #30187, #28844, .T. ) ;
#32274=CARTESIAN_POINT ( 'NONE',  ( -27.94687998398240225, -24.71358538153085149, -6.293495900045230407 ) ) ;
#32275=CARTESIAN_POINT ( 'NONE',  ( 5.399542109131928669, -22.95868181222395066, -15.85264200238205312 ) ) ;
#32276=CARTESIAN_POINT ( 'NONE',  ( 11.09252425524408459, 17.23965631597926418, -29.35067692373401016 ) ) ;
#32278=CARTESIAN_POINT ( 'NONE',  ( 16.75470528484330046, 11.98919836256815330, -27.72802603258947229 ) ) ;
#32282=CARTESIAN_POINT ( 'NONE',  ( -8.724803901531640093, 32.67470959390297480, -11.16207224700029776 ) ) ;
#32285=CARTESIAN_POINT ( 'NONE',  ( -15.32303194119059420, -26.70022385808693954, -5.474162114618875030 ) ) ;
#32289=CARTESIAN_POINT ( 'NONE',  ( 23.32290838231767438, 0.5357531857212454174, -20.54009308810276124 ) ) ;
#32292=EDGE_LOOP ( 'NONE', ( #14886, #30034, #7123, #10054, #26320, #7929, #19435, #17672 ) ) ;
#32293=CARTESIAN_POINT ( 'NONE',  ( -30.74131631141073129, 0.1242922002067066989, -4.999999999999999112 ) ) ;
#32295=CARTESIAN_POINT ( 'NONE',  ( 35.21367278186023952, -9.523108846389430227, -6.737064075858604006 ) ) ;
#32306=FILL_AREA_STYLE_COLOUR ( '', #20997 ) ;
#32312=CARTESIAN_POINT ( 'NONE',  ( 17.18224089502211882, 16.15582687960090524, -15.85542385682627753 ) ) ;
#32314=CARTESIAN_POINT ( 'NONE',  ( 11.71220820147315500, 33.45731985618542836, -5.448922514974672282 ) ) ;
#32318=CARTESIAN_POINT ( 'NONE',  ( 13.47515517589329903, -22.56152428954667144, -16.35616346769606722 ) ) ;
#32322=CARTESIAN_POINT ( 'NONE',  ( -13.77105083670779173, 23.39240968089663397, -14.47666898018377779 ) ) ;
#32324=CARTESIAN_POINT ( 'NONE',  ( 12.54367332990374173, -23.06920662023509294, -15.48107427365479261 ) ) ;
#32328=CARTESIAN_POINT ( 'NONE',  ( -13.31194575400795443, 31.44560903785412265, -5.455421079577211785 ) ) ;
#32329=CARTESIAN_POINT ( 'NONE',  ( -12.11431924477676425, -16.53859993892360336, -29.29246340206837473 ) ) ;
#32332=CIRCLE ( 'NONE', #32982, 21.00000000000002842 ) ;
#32333=CARTESIAN_POINT ( 'NONE',  ( -34.62559140834917315, -8.582204632672675970, -8.048554430461706488 ) ) ;
#32336=CARTESIAN_POINT ( 'NONE',  ( 30.34379296090365941, 0.1366719566521715779, -7.828841148755459223 ) ) ;
#32343=CARTESIAN_POINT ( 'NONE',  ( -20.69487421836006291, 0.8272276961458596700, -27.44708463700338541 ) ) ;
#32346=CARTESIAN_POINT ( 'NONE',  ( 21.97238824968331627, -1.114103264437971808, -23.63409279004794072 ) ) ;
#32359=CARTESIAN_POINT ( 'NONE',  ( 3.957996558887789451, 29.70837811692673469, -15.71455925150293176 ) ) ;
#32361=CARTESIAN_POINT ( 'NONE',  ( 17.34253826607186255, 27.32041144404028543, -5.000000000000000000 ) ) ;
#32365=CARTESIAN_POINT ( 'NONE',  ( -19.26428189677079317, 7.107870580791990633, -28.84674469903880123 ) ) ;
#32367=CARTESIAN_POINT ( 'NONE',  ( 18.47528072167350643, -21.61393943133635531, -15.95044983778787895 ) ) ;
#32371=CARTESIAN_POINT ( 'NONE',  ( 10.89890768951664946, 17.41657833809615141, -28.70249223529265947 ) ) ;
#32372=EDGE_LOOP ( 'NONE', ( #640, #22477, #38861, #23312 ) ) ;
#32373=CARTESIAN_POINT ( 'NONE',  ( -15.78519146989449951, 25.10981109001613731, -6.891642859120278963 ) ) ;
#32376=CARTESIAN_POINT ( 'NONE',  ( 14.05944288250579888, 23.86579217215976101, -13.51649411389087696 ) ) ;
#32378=CARTESIAN_POINT ( 'NONE',  ( 33.04045786196795120, -19.54937996555464963, -6.275779577593939784 ) ) ;
#32380=CARTESIAN_POINT ( 'NONE',  ( -14.99270781980373179, 26.86396254207275547, -8.275605574745005910 ) ) ;
#32383=CARTESIAN_POINT ( 'NONE',  ( -16.22334360803714404, -26.92298677526160233, -5.470646933448687577 ) ) ;
#32386=CARTESIAN_POINT ( 'NONE',  ( -33.38192493758457857, -13.76034026150677647, -9.745630752933474028 ) ) ;
#32387=CARTESIAN_POINT ( 'NONE',  ( -14.54159974610060502, -26.13620151684259341, -8.302464661525958078 ) ) ;
#32389=CARTESIAN_POINT ( 'NONE',  ( 14.48425105757694276, 16.48989445216367500, -21.99809950758036337 ) ) ;
#32391=CARTESIAN_POINT ( 'NONE',  ( 25.79239026209233288, 2.921625702708928962, -13.66086306012633500 ) ) ;
#32397=CARTESIAN_POINT ( 'NONE',  ( -20.98656222130776072, 0.6382380030884662325, -26.20988820701830946 ) ) ;
#32399=CARTESIAN_POINT ( 'NONE',  ( 21.31785039509857782, 0.4639204330908863749, -24.98034756807314238 ) ) ;
#32403=CARTESIAN_POINT ( 'NONE',  ( -25.99398016003019762, 1.074985532622513063, -15.51177067371635587 ) ) ;
#32405=CARTESIAN_POINT ( 'NONE',  ( -13.47223693944937040, 18.09844039693852125, -29.99999999999999645 ) ) ;
#32415=CARTESIAN_POINT ( 'NONE',  ( 21.63954851288776382, -20.01129605949122592, -15.78715110015275691 ) ) ;
#32418=CARTESIAN_POINT ( 'NONE',  ( 13.19794165967893740, 23.39120655137475779, -15.38553023868800196 ) ) ;
#32422=CARTESIAN_POINT ( 'NONE',  ( -16.78065708880074425, 18.17327365419953011, -13.77701268753624753 ) ) ;
#32424=CARTESIAN_POINT ( 'NONE',  ( 14.97653007950890469, -26.12221433204903320, -8.768684533753454247 ) ) ;
#32426=CARTESIAN_POINT ( 'NONE',  ( 11.13469544420071067, 17.60622615329656071, -26.83131557681828383 ) ) ;
#32428=CARTESIAN_POINT ( 'NONE',  ( 14.83827637938750321, 25.61447254529330664, -10.18026005582235527 ) ) ;
#32431=CARTESIAN_POINT ( 'NONE',  ( -12.34392958471658730, 20.55351014499400364, -19.48636728564961373 ) ) ;
#32433=CARTESIAN_POINT ( 'NONE',  ( -9.686854926055254111, -18.44287383492480714, -26.83074955385285421 ) ) ;
#32435=CARTESIAN_POINT ( 'NONE',  ( -17.65620682731983848, -12.15726045169065550, -25.58993171772528541 ) ) ;
#32436=CARTESIAN_POINT ( 'NONE',  ( -6.928215406011057453, -24.90100025669732631, -8.373177299821190189 ) ) ;
#32437=CARTESIAN_POINT ( 'NONE',  ( 15.72808583165933172, 25.07803225150221493, -7.363722881524870090 ) ) ;
#32439=CARTESIAN_POINT ( 'NONE',  ( 22.02868513814706830, 8.851876989647921690, -13.87910646370428580 ) ) ;
#32440=CARTESIAN_POINT ( 'NONE',  ( 20.30751140574952629, -27.27504018040222533, -4.999999999999999112 ) ) ;
#32445=CARTESIAN_POINT ( 'NONE',  ( -20.64083728193717349, -1.144092991643025359, -27.97724812587252785 ) ) ;
#32451=CARTESIAN_POINT ( 'NONE',  ( 18.74042788058114795, -8.920399457985654479, -27.71296284416046518 ) ) ;
#32463=CARTESIAN_POINT ( 'NONE',  ( -1.397011542984961219, 27.89542180380697189, -17.59998838210181660 ) ) ;
#32467=LINE ( 'NONE', #26357, #13033 ) ;
#32470=CARTESIAN_POINT ( 'NONE',  ( 9.263407132367138530, 18.28842304576874156, -29.99999999999999645 ) ) ;
#32475=CARTESIAN_POINT ( 'NONE',  ( -19.66039451765587387, 12.90996750491107115, -13.90270306263754030 ) ) ;
#32478=CARTESIAN_POINT ( 'NONE',  ( 13.41104112211880128, -23.62643484690040907, -14.47296996873020092 ) ) ;
#32480=CARTESIAN_POINT ( 'NONE',  ( 10.95101281418289219, 17.32990059288363582, -30.00000000000000355 ) ) ;
#32481=CARTESIAN_POINT ( 'NONE',  ( -20.90924525106831666, -8.502318254486386451, -19.80438750953543803 ) ) ;
#32483=CARTESIAN_POINT ( 'NONE',  ( -18.43289261102269450, -17.30365355162674135, -19.79000791179135632 ) ) ;
#32484=CARTESIAN_POINT ( 'NONE',  ( 3.713915702903541227, -23.75747772264873348, -12.86660365504189407 ) ) ;
#32485=CARTESIAN_POINT ( 'NONE',  ( 13.89868614485595621, 23.12070620105854601, -14.49265882329358313 ) ) ;
#32486=CARTESIAN_POINT ( 'NONE',  ( 21.08270858168392792, 12.99488455910146278, -5.967554639584160547 ) ) ;
#32491=CARTESIAN_POINT ( 'NONE',  ( -6.053964587434877309, 34.92638846911022910, -10.20850310494260782 ) ) ;
#32499=ORIENTED_EDGE ( 'NONE', *, *, #33684, .T. ) ;
#32500=CARTESIAN_POINT ( 'NONE',  ( -30.61700640880846791, 0.08162764009042081104, -6.888198014876335762 ) ) ;
#32502=CARTESIAN_POINT ( 'NONE',  ( 20.02039722198771088, -4.740659622082477931, -28.52478632098719658 ) ) ;
#32508=VERTEX_POINT ( 'NONE', #24559 ) ;
#32511=ADVANCED_FACE ( 'NONE', ( #12165 ), #14817, .T. ) ;
#32521=CARTESIAN_POINT ( 'NONE',  ( 15.35486525779784728, 13.76085684245165552, -27.69159219027432783 ) ) ;
#32522=CARTESIAN_POINT ( 'NONE',  ( 7.493380996195920574, 25.92983308932212339, -17.81133628007513892 ) ) ;
#32526=CARTESIAN_POINT ( 'NONE',  ( 10.39272730050880789, -19.10536722629138140, -23.83256194882331869 ) ) ;
#32530=CARTESIAN_POINT ( 'NONE',  ( -14.28250818835134872, 24.49381330739200990, -12.54868123938283375 ) ) ;
#32533=CARTESIAN_POINT ( 'NONE',  ( 11.58908824346749178, -21.50996719514929723, -18.48308237374000029 ) ) ;
#32538=CARTESIAN_POINT ( 'NONE',  ( -7.847358392957297646, 19.47655254888744736, -26.54680820890942883 ) ) ;
#32541=CARTESIAN_POINT ( 'NONE',  ( -34.16618095875499250, -7.443595052282137914, -8.509874465049289682 ) ) ;
#32544=CARTESIAN_POINT ( 'NONE',  ( 25.75329700475152706, 0.5046424211543979466, -16.46013763815398789 ) ) ;
#32549=CARTESIAN_POINT ( 'NONE',  ( -29.99827651847404297, 0.02216799781674966274, -9.238322543644144957 ) ) ;
#32552=CARTESIAN_POINT ( 'NONE',  ( 26.14237992437378466, -1.587135967906720291, -17.20498952483474042 ) ) ;
#32563=CARTESIAN_POINT ( 'NONE',  ( 2.292311336812923095, 22.67302623323931243, -23.01638908516527238 ) ) ;
#32564=CARTESIAN_POINT ( 'NONE',  ( -14.23945615837876311, -31.58416516429889853, 0.000000000000000000 ) ) ;
#32567=CARTESIAN_POINT ( 'NONE',  ( 16.07137580887406969, -18.82834282195213405, -19.98174329064899979 ) ) ;
#32568=DIRECTION ( 'NONE',  ( -1.000000000000000000, 0.000000000000000000, 0.000000000000000000 ) ) ;
#32572=CARTESIAN_POINT ( 'NONE',  ( 11.23935683279430364, 18.09303880744939619, -25.00484586747397842 ) ) ;
#32574=CARTESIAN_POINT ( 'NONE',  ( -11.42515256197113693, 17.40157771485680627, -26.85803077672003525 ) ) ;
#32577=CARTESIAN_POINT ( 'NONE',  ( 12.96728218553863954, 21.59012440819528322, -17.44419411314543567 ) ) ;
#32579=CARTESIAN_POINT ( 'NONE',  ( 32.16900669001064728, -16.47211036377505167, -10.17477865279244043 ) ) ;
#32581=CARTESIAN_POINT ( 'NONE',  ( -11.12826152366268850, 18.17846884760333381, -24.98958924420576722 ) ) ;
#32583=CARTESIAN_POINT ( 'NONE',  ( -17.02243939560907648, -26.72822735494350965, -7.774529914931894936 ) ) ;
#32587=CARTESIAN_POINT ( 'NONE',  ( -19.77651789229256352, -8.197028377600723559, -25.61779185879715115 ) ) ;
#32588=CARTESIAN_POINT ( 'NONE',  ( -11.55200745323391764, -21.51294090668309167, -18.48664492717743713 ) ) ;
#32590=CARTESIAN_POINT ( 'NONE',  ( 16.82875782630935291, 20.37066115841360059, -10.28574066425471933 ) ) ;
#32592=CARTESIAN_POINT ( 'NONE',  ( 25.33665828877437320, 2.928795514553437673, -14.64692555173594357 ) ) ;
#32597=CARTESIAN_POINT ( 'NONE',  ( -30.95948536022075359, -0.1350361458710127027, -5.944726679833734373 ) ) ;
#32598=CARTESIAN_POINT ( 'NONE',  ( 20.85121071602917553, 0.3501234034299393616, -26.79320176925520514 ) ) ;
#32603=CARTESIAN_POINT ( 'NONE',  ( -28.85560228327580390, 1.748727845287112448, -7.841872307111799500 ) ) ;
#32605=CARTESIAN_POINT ( 'NONE',  ( -18.07620401364299667, 24.68088026512193167, -13.58461195433497082 ) ) ;
#32614=CARTESIAN_POINT ( 'NONE',  ( -25.53096875586516390, 6.216240356532259703, -5.000000000000001776 ) ) ;
#32619=CARTESIAN_POINT ( 'NONE',  ( 27.75063338421220749, -24.13809418093133274, -8.005686737521594765 ) ) ;
#32622=CARTESIAN_POINT ( 'NONE',  ( 14.77821352920928177, 26.27987808421032057, -9.682826709401501475 ) ) ;
#32626=CARTESIAN_POINT ( 'NONE',  ( -15.52764069369276889, 16.28833658513694260, -19.93923883857963375 ) ) ;
#32629=CARTESIAN_POINT ( 'NONE',  ( 9.636746047937265303, -18.46635915234381997, -26.83497180128339110 ) ) ;
#32631=CARTESIAN_POINT ( 'NONE',  ( 14.84964465211067441, 25.58025656879111054, -10.18089330217375910 ) ) ;
#32633=CARTESIAN_POINT ( 'NONE',  ( 15.41298789278284964, 26.79417030376202291, -5.474208755804808035 ) ) ;
#32635=CARTESIAN_POINT ( 'NONE',  ( -11.63031588870816257, 18.96513858619488602, -22.72542786189888986 ) ) ;
#32636=DIRECTION ( 'NONE',  ( 0.000000000000000000, 0.000000000000000000, 1.000000000000000000 ) ) ;
#32637=CARTESIAN_POINT ( 'NONE',  ( -14.61166790280883099, -25.45836085479211164, -10.65401685762440387 ) ) ;
#32640=CARTESIAN_POINT ( 'NONE',  ( -31.61852543657527903, -20.43336672873744675, -7.973887691128377142 ) ) ;
#32641=CARTESIAN_POINT ( 'NONE',  ( -6.215971932975158154, -23.28253663301664389, -14.81238128996371195 ) ) ;
#32642=CARTESIAN_POINT ( 'NONE',  ( 12.34902707657751186, 18.26588438466833608, -22.83901375834292224 ) ) ;
#32644=CARTESIAN_POINT ( 'NONE',  ( 20.46894310308663734, 7.564869913809710411, -21.11451722641894690 ) ) ;
#32649=CARTESIAN_POINT ( 'NONE',  ( -24.71030582546459442, -1.630746468800712279, -19.22827620953929184 ) ) ;
#32656=CARTESIAN_POINT ( 'NONE',  ( 18.51815053109030629, -8.815588134695456546, -29.21493728961338476 ) ) ;
#32658=ORIENTED_EDGE ( 'NONE', *, *, #11589, .T. ) ;
#32664=CARTESIAN_POINT ( 'NONE',  ( 0.2270303117876434351, 21.43481588860569076, -25.57708852813776801 ) ) ;
#32667=DIRECTION ( 'NONE',  ( 1.000000000000000000, 0.000000000000000000, 0.000000000000000000 ) ) ;
#32673=CARTESIAN_POINT ( 'NONE',  ( 14.35878712486879039, 29.02377999103498496, -7.294375021701867468 ) ) ;
#32676=CARTESIAN_POINT ( 'NONE',  ( -17.19661888337742184, 12.08206334730271791, -24.39846010520068731 ) ) ;
#32679=CARTESIAN_POINT ( 'NONE',  ( 9.990270308899361851, -18.80412660014683013, -25.01178681032867956 ) ) ;
#32681=CARTESIAN_POINT ( 'NONE',  ( 14.92120918266745733, 25.84352239596041301, -9.706504909383646407 ) ) ;
#32682=CARTESIAN_POINT ( 'NONE',  ( -19.54664213359414404, -11.28525909758381829, -30.00000000000000711 ) ) ;
#32684=CARTESIAN_POINT ( 'NONE',  ( -23.72267846501879518, -21.04549334238744507, -13.87629623305566007 ) ) ;
#32685=CARTESIAN_POINT ( 'NONE',  ( 3.569601909448802513, -23.23944431787124643, -14.89441082719224596 ) ) ;
#32686=CARTESIAN_POINT ( 'NONE',  ( 11.47796835573551988, 17.90614830826391923, -25.03692986855586256 ) ) ;
#32687=CARTESIAN_POINT ( 'NONE',  ( 20.05787158664475101, 13.58148755638892169, -10.87997266152090781 ) ) ;
#32691=CARTESIAN_POINT ( 'NONE',  ( -7.446792957322618811, 36.70800515527383823, -4.999999999999999112 ) ) ;
#32700=CARTESIAN_POINT ( 'NONE',  ( -21.25873018001586701, 0.9006927932260392344, -25.02786347552343926 ) ) ;
#32702=CARTESIAN_POINT ( 'NONE',  ( 34.75575196650723342, -11.62799908373506419, -8.009968735996103817 ) ) ;
#32717=EDGE_CURVE ( 'NONE', #34673, #860, #838, .T. ) ;
#32718=CARTESIAN_POINT ( 'NONE',  ( 15.43899379198432165, 13.87320894201425858, -26.55943958658228254 ) ) ;
#32719=CARTESIAN_POINT ( 'NONE',  ( 11.64958443988100711, 33.23480978958207999, -6.767891074995996625 ) ) ;
#32720=AXIS2_PLACEMENT_3D ( 'NONE', #8468, #20867, #33268 ) ;
#32724=CARTESIAN_POINT ( 'NONE',  ( 15.64462842542821797, -26.65633373546051743, -6.882370998507620463 ) ) ;
#32728=CARTESIAN_POINT ( 'NONE',  ( -14.28759343413927674, 24.48013941304578367, -12.54985307008666418 ) ) ;
#32730=CARTESIAN_POINT ( 'NONE',  ( 13.61137063728712349, -26.17156308209870019, -6.892411826510384643 ) ) ;
#32733=ORIENTED_EDGE ( 'NONE', *, *, #23505, .T. ) ;
#32734=CARTESIAN_POINT ( 'NONE',  ( -8.174017679424943950, 22.40856258689699843, -21.07428364536496446 ) ) ;
#32739=CARTESIAN_POINT ( 'NONE',  ( -31.44780373369627924, -5.846625527196687599, -12.15987862009057707 ) ) ;
#32742=CARTESIAN_POINT ( 'NONE',  ( 30.80134931806678722, 0.02728179087148215054, -5.946091737772539076 ) ) ;
#32746=CARTESIAN_POINT ( 'NONE',  ( -1.485571585149857210, -11.24999999999982236, 6.000000000000000000 ) ) ;
#32748=CARTESIAN_POINT ( 'NONE',  ( -23.93868645767142311, 0.4905013439724816293, -19.49701671461600938 ) ) ;
#32751=CARTESIAN_POINT ( 'NONE',  ( 31.41098121239500784, -3.786779113504257221, -11.32952589658759024 ) ) ;
#32763=ADVANCED_FACE ( 'NONE', ( #22296 ), #12562, .T. ) ;
#32766=CARTESIAN_POINT ( 'NONE',  ( 4.894819805308785909, 36.72758954802892362, -8.421019001303848839 ) ) ;
#32769=CARTESIAN_POINT ( 'NONE',  ( 18.34994596701333691, -24.10411726525174458, -13.18475438623739926 ) ) ;
#32772=CARTESIAN_POINT ( 'NONE',  ( -35.10501578368283049, -15.25571008401125717, -4.999999999999999112 ) ) ;
#32774=ORIENTED_EDGE ( 'NONE', *, *, #35196, .T. ) ;
#32775=CARTESIAN_POINT ( 'NONE',  ( 15.36283324375265025, 26.87922326031363340, -5.944726108962296252 ) ) ;
#32778=CARTESIAN_POINT ( 'NONE',  ( -15.55253742554085150, 26.04285000535905681, -6.417767331807119113 ) ) ;
#32781=CARTESIAN_POINT ( 'NONE',  ( 15.13424392241500804, 26.03117488544685187, -8.768685094158927384 ) ) ;
#32783=CARTESIAN_POINT ( 'NONE',  ( 25.05307922697820189, -14.82438956320695667, -16.62383189019713825 ) ) ;
#32785=CARTESIAN_POINT ( 'NONE',  ( -14.53593441609714532, 27.81463984687436408, -8.695921198377391192 ) ) ;
#32787=CARTESIAN_POINT ( 'NONE',  ( -16.45245987805732923, -25.93375551561933179, -10.08876688787445097 ) ) ;
#32788=EDGE_CURVE ( 'NONE', #1089, #10807, #13944, .T. ) ;
#32790=ORIENTED_EDGE ( 'NONE', *, *, #10166, .T. ) ;
#32791=CARTESIAN_POINT ( 'NONE',  ( -19.15932531068841982, -7.943154726143056621, -27.72915435580758015 ) ) ;
#32792=CARTESIAN_POINT ( 'NONE',  ( -14.25497869358564706, -25.70370180133969384, -9.718373509854576042 ) ) ;
#32794=CARTESIAN_POINT ( 'NONE',  ( 13.97033939041524597, 17.09349275497558196, -21.93499464288763079 ) ) ;
#32795=EDGE_LOOP ( 'NONE', ( #6578, #19247 ) ) ;
#32796=CARTESIAN_POINT ( 'NONE',  ( 20.47381378144825703, 2.410701076763831718, -28.14891251935899774 ) ) ;
#32801=CARTESIAN_POINT ( 'NONE',  ( -24.68539487710851787, 0.1722238459068671235, -18.41696137871380046 ) ) ;
#32803=CARTESIAN_POINT ( 'NONE',  ( 28.26373143719677472, -0.5205252554743069471, -13.43917560083705887 ) ) ;
#32806=CARTESIAN_POINT ( 'NONE',  ( -27.50575908014011972, 1.800164312645714082, -11.66087879572743446 ) ) ;
#32808=CARTESIAN_POINT ( 'NONE',  ( 2.927345865710861972E-15, 22.57051819516765789, -30.00000000000001421 ) ) ;
#32814=CARTESIAN_POINT ( 'NONE',  ( 16.00000000000000000, 22.50000000000000711, 0.000000000000000000 ) ) ;
#32817=CARTESIAN_POINT ( 'NONE',  ( -25.29540831655226185, 6.194354954019752668, -7.886033299896356930 ) ) ;
#32820=CARTESIAN_POINT ( 'NONE',  ( 16.10474936713543315, -14.84555984040918553, -24.35669833423021302 ) ) ;
#32824=CARTESIAN_POINT ( 'NONE',  ( 14.94663361625261189, 26.63105489887620081, -8.746052331878477304 ) ) ;
#32827=CARTESIAN_POINT ( 'NONE',  ( -16.02262695881562848, 21.94564375748138474, -10.73340876258623844 ) ) ;
#32829=CARTESIAN_POINT ( 'NONE',  ( 15.23784189583742865, -26.55597465737094609, -6.888200020279732882 ) ) ;
#32831=CARTESIAN_POINT ( 'NONE',  ( 14.03714680842188756, 23.91771073391425517, -13.51393999334652207 ) ) ;
#32836=CARTESIAN_POINT ( 'NONE',  ( -12.56505670423899446, 21.18481041280805144, -18.43279161028919333 ) ) ;
#32838=CARTESIAN_POINT ( 'NONE',  ( -11.92035180994863097, -21.48388645554785725, -18.45049858032665924 ) ) ;
#32842=CARTESIAN_POINT ( 'NONE',  ( -32.28394191823594639, -20.85172211888466620, -5.000000000000000888 ) ) ;
#32843=CARTESIAN_POINT ( 'NONE',  ( -6.188423164013283184, -19.73497389761912046, -27.63864133075322016 ) ) ;
#32844=CARTESIAN_POINT ( 'NONE',  ( 12.01968976909422260, 17.96829324440782827, -23.93304672575846581 ) ) ;
#32846=CARTESIAN_POINT ( 'NONE',  ( 19.85109443489771408, 8.256135034430100106, -22.21491113497751613 ) ) ;
#32852=CARTESIAN_POINT ( 'NONE',  ( -31.51724108361762688, -1.592384348128919935, -8.686465100392110728 ) ) ;
#32857=CARTESIAN_POINT ( 'NONE',  ( 33.54263992596453647, -17.18436309121399574, -7.973046152344251070 ) ) ;
#32864=CARTESIAN_POINT ( 'NONE',  ( 0.8942644845752143468, 22.01017621520333378, -24.22054542436852742 ) ) ;
#32873=CARTESIAN_POINT ( 'NONE',  ( 13.45995091351214690, 25.18522299110997764, -13.40001028691244400 ) ) ;
#32876=CARTESIAN_POINT ( 'NONE',  ( -18.48907582165858798, 14.46313849928662165, -14.89271776214601140 ) ) ;
#32880=CARTESIAN_POINT ( 'NONE',  ( 14.77006329367439896, -25.65908439595070334, -10.17951868138070992 ) ) ;
#32883=CARTESIAN_POINT ( 'NONE',  ( 15.40660648310854164, 26.81700542816128063, -5.474045217557533149 ) ) ;
#32884=CARTESIAN_POINT ( 'NONE',  ( 17.34253826539385201, 27.32041144647958575, -5.000000000000000000 ) ) ;
#32886=CARTESIAN_POINT ( 'NONE',  ( -19.16391196221957571, -17.99803450724484222, -18.76479932701361975 ) ) ;
#32887=CARTESIAN_POINT ( 'NONE',  ( 1.817969461173305490, -24.76413945269762351, -5.483170422348042194 ) ) ;
#32888=CARTESIAN_POINT ( 'NONE',  ( 14.87733101683222614, 24.99273381504638891, -10.66221022678619867 ) ) ;
#32889=CARTESIAN_POINT ( 'NONE',  ( 19.10285424782163233, 12.84828869033409049, -15.93831158563282102 ) ) ;
#32892=CARTESIAN_POINT ( 'NONE',  ( -5.072650811858919973, 29.32414667381679863, -15.74330015237563529 ) ) ;
#32904=CARTESIAN_POINT ( 'NONE',  ( -28.54007740871540122, 0.5227748155925792117, -11.61433878387980378 ) ) ;
#32906=CARTESIAN_POINT ( 'NONE',  ( 20.95614885317017695, -6.336004544166005559, -24.36784054283095458 ) ) ;
#32917=EDGE_CURVE ( 'NONE', #3398, #8093, #22366, .T. ) ;
#32918=CARTESIAN_POINT ( 'NONE',  ( 15.32941689225309112, 13.72693657690245672, -28.26505645429302405 ) ) ;
#32920=CARTESIAN_POINT ( 'NONE',  ( 12.35192597829481009, 32.37184802151152496, -6.781871780508718750 ) ) ;
#32923=DIRECTION ( 'NONE',  ( 0.000000000000000000, 0.000000000000000000, 1.000000000000000000 ) ) ;
#32925=CARTESIAN_POINT ( 'NONE',  ( 15.10869851544610931, -25.55731746936413629, -10.62300024995772318 ) ) ;
#32930=CARTESIAN_POINT ( 'NONE',  ( -14.02126489188123060, 23.95563206446321303, -13.51135549859506746 ) ) ;
#32932=CARTESIAN_POINT ( 'NONE',  ( 10.32640477728945072, -21.13211831446180611, -19.62180369577067296 ) ) ;
#32936=CARTESIAN_POINT ( 'NONE',  ( -12.37123995031714863, 31.49198740136808539, -8.565043564655828945 ) ) ;
#32939=CARTESIAN_POINT ( 'NONE',  ( -20.77014107886579808, -3.131800453615022573, -26.53419280964595117 ) ) ;
#32942=CARTESIAN_POINT ( 'NONE',  ( 23.91506835619285809, 0.5469039752616722261, -19.50346979283914450 ) ) ;
#32948=CARTESIAN_POINT ( 'NONE',  ( -20.48147506303724441, 0.8713082578521275101, -29.34858951695225571 ) ) ;
#32952=CARTESIAN_POINT ( 'NONE',  ( 33.38598080700936066, -4.103730722464701053, -7.695482771259642973 ) ) ;
#32968=CARTESIAN_POINT ( 'NONE',  ( 3.380733272816430546, 20.85284384237622746, -26.30940457203467275 ) ) ;
#32972=CARTESIAN_POINT ( 'NONE',  ( 19.71634060764898067, -27.14742637253563373, -6.361116528107567447 ) ) ;
#32978=CARTESIAN_POINT ( 'NONE',  ( 14.98081254870050039, 26.09019376164257409, -9.232264583633339683 ) ) ;
#32981=CARTESIAN_POINT ( 'NONE',  ( -12.66284596178592459, 20.13327502018258031, -19.54334862798365080 ) ) ;
#32982=AXIS2_PLACEMENT_3D ( 'NONE', #35833, #29535, #17956 ) ;
#32986=CARTESIAN_POINT ( 'NONE',  ( 14.79573094385063037, 25.22704658224830254, -10.65696934714573985 ) ) ;
#32988=CARTESIAN_POINT ( 'NONE',  ( 31.85050647178360705, -20.18765053876312265, -7.972301957832756969 ) ) ;
#32991=CARTESIAN_POINT ( 'NONE',  ( -14.79259077307489889, 26.65558470197620267, -9.204917952329308761 ) ) ;
#32993=CARTESIAN_POINT ( 'NONE',  ( -18.29333439512888759, -27.14906503354761824, -6.376644952967080116 ) ) ;
#32997=CARTESIAN_POINT ( 'NONE',  ( -29.92619010456159856, -11.28214714606756175, -13.85028604681554754 ) ) ;
#32998=CARTESIAN_POINT ( 'NONE',  ( -14.15683454941679464, -25.37115389201304438, -10.66325925726328272 ) ) ;
#33001=CARTESIAN_POINT ( 'NONE',  ( 29.14407284010881227, 1.139970232528481953, -8.782330516724952574 ) ) ;
#33006=EDGE_CURVE ( 'NONE', #31948, #7370, #12004, .T. ) ;
#33007=CARTESIAN_POINT ( 'NONE',  ( -24.60177868520493050, 0.3453315261475468634, -18.44044427177923851 ) ) ;
#33009=CARTESIAN_POINT ( 'NONE',  ( 20.63866867332527022, 0.2073280320569168000, -28.04521516201818443 ) ) ;
#33012=CARTESIAN_POINT ( 'NONE',  ( -27.90312125966312351, 1.785194626332250234, -10.70166145795786150 ) ) ;
#33013=CARTESIAN_POINT ( 'NONE',  ( -11.31392148919591811, 36.91540483778867099, -5.000000000000009770 ) ) ;
#33025=CARTESIAN_POINT ( 'NONE',  ( -22.35010935049834657, 5.092895750971690561, -18.86795456680612304 ) ) ;
#33028=CARTESIAN_POINT ( 'NONE',  ( 15.24051681827566718, -14.92785667918263925, -25.72502823181857323 ) ) ;
#33031=CARTESIAN_POINT ( 'NONE',  ( 15.28661535835308349, 27.13569895802415388, -5.942075632022802090 ) ) ;
#33034=CARTESIAN_POINT ( 'NONE',  ( -16.73766650064135320, 21.43861104905754189, -8.822088556755165456 ) ) ;
#33037=CARTESIAN_POINT ( 'NONE',  ( 12.66086287625040541, 21.04242839094937167, -18.45356328166587900 ) ) ;
#33041=CARTESIAN_POINT ( 'NONE',  ( -12.03858661653558748, 20.03409609272645397, -20.52224590143303828 ) ) ;
#33043=CARTESIAN_POINT ( 'NONE',  ( -15.41099496508465982, -26.52696749137851384, -7.355554215977166521 ) ) ;
#33045=CIRCLE ( 'NONE', #10963, 62.00000000000014211 ) ;
#33047=CARTESIAN_POINT ( 'NONE',  ( -33.23797450146873445, -18.71509596241817164, -7.116742953870333288 ) ) ;
#33048=CARTESIAN_POINT ( 'NONE',  ( -6.760112097234737050, -24.51974927990703179, -10.32779609532193454 ) ) ;
#33050=CARTESIAN_POINT ( 'NONE',  ( 11.67910349775616652, 17.21656688193314366, -26.88047951749153341 ) ) ;
#33052=CARTESIAN_POINT ( 'NONE',  ( 25.32158894843077945, 6.480252874148680675, -5.478621571544178614 ) ) ;
#33053=CARTESIAN_POINT ( 'NONE',  ( -17.34253826607186966, 27.32041144404027122, 0.000000000000000000 ) ) ;
#33058=CARTESIAN_POINT ( 'NONE',  ( -30.86022713980213794, -1.524650393404385129, -10.07426524678920821 ) ) ;
#33059=CARTESIAN_POINT ( 'NONE',  ( 29.65047528457347426, -0.01023675481382509654, -10.17575680121469262 ) ) ;
#33070=CARTESIAN_POINT ( 'NONE',  ( 0.3375428170692008623, 31.33837579149849262, -14.73082907740201009 ) ) ;
#33074=AXIS2_PLACEMENT_3D ( 'NONE', #424, #620, #12406 ) ;
#33078=CARTESIAN_POINT ( 'NONE',  ( 14.90467518106525269, 28.31725849260483585, -5.467169310882759703 ) ) ;
#33081=CARTESIAN_POINT ( 'NONE',  ( -19.04904607429094554, 15.01394467124153564, -11.86198345635079932 ) ) ;
#33084=CARTESIAN_POINT ( 'NONE',  ( 13.73281793707762155, -24.12020055917744799, -13.51159965186342404 ) ) ;
#33086=CARTESIAN_POINT ( 'NONE',  ( 10.95987886464238059, 17.32429135621979555, -30.00000000000000355 ) ) ;
#33089=CARTESIAN_POINT ( 'NONE',  ( -17.11419722955264433, -16.05889537474196516, -22.00308921696831632 ) ) ;
#33090=CARTESIAN_POINT ( 'NONE',  ( 1.732327452010537616, -24.13709212142373062, -10.88692373186505336 ) ) ;
#33091=CARTESIAN_POINT ( 'NONE',  ( 13.62424208523637859, 22.55708696713261929, -15.46943763161296559 ) ) ;
#33092=CARTESIAN_POINT ( 'NONE',  ( 18.69607909436101423, 11.44394688062264009, -20.12350778403434504 ) ) ;
#33095=CARTESIAN_POINT ( 'NONE',  ( -5.707447616493412923, 27.97779256337231146, -16.72301236455337303 ) ) ;
#33096=VERTEX_POINT ( 'NONE', #27753 ) ;
#33101=EDGE_CURVE ( 'NONE', #26001, #27435, #11524, .T. ) ;
#33105=CARTESIAN_POINT ( 'NONE',  ( -20.95165138070167998, 0.9770979443023026789, -26.23948052383034479 ) ) ;
#33107=CARTESIAN_POINT ( 'NONE',  ( 34.27195656595002760, -11.45219146868936910, -8.887004270612056445 ) ) ;
#33120=CARTESIAN_POINT ( 'NONE',  ( 14.89366125532731822, 14.36502201557359193, -27.10073944775506760 ) ) ;
#33121=CARTESIAN_POINT ( 'NONE',  ( 11.88982892552273007, 30.98811914902011111, -9.910042724562915240 ) ) ;
#33123=CARTESIAN_POINT ( 'NONE',  ( -19.59276562800022248, 8.779838875553902966, -22.22895676643048191 ) ) ;
#33125=DIRECTION ( 'NONE',  ( -0.000000000000000000, -0.000000000000000000, -1.000000000000000000 ) ) ;
#33128=CARTESIAN_POINT ( 'NONE',  ( 10.70129962474131879, -19.52760334584666069, -22.71333977806620297 ) ) ;
#33132=CARTESIAN_POINT ( 'NONE',  ( -13.48068414432812645, 22.83747268959859511, -15.44824800343550919 ) ) ;
#33134=CARTESIAN_POINT ( 'NONE',  ( 11.05990709802074257, -21.55257169122715410, -18.53364441852212252 ) ) ;
#33138=CARTESIAN_POINT ( 'NONE',  ( -7.322902666698219321, 19.93973914737491526, -25.85775467558311647 ) ) ;
#33144=CARTESIAN_POINT ( 'NONE',  ( 20.52456465525489193, 0.9065716826278377161, -28.70867527313039602 ) ) ;
#33146=CYLINDRICAL_SURFACE ( 'NONE', #35556, 21.00000000000002842 ) ;
#33150=CARTESIAN_POINT ( 'NONE',  ( -29.58395905627514821, 0.06330276854539861053, -10.18073491376308404 ) ) ;
#33155=CARTESIAN_POINT ( 'NONE',  ( 25.01210607124402685, -2.904145798682293389, -19.09601541136637337 ) ) ;
#33168=CARTESIAN_POINT ( 'NONE',  ( 6.754942957401739889, 34.60620598615416554, -10.21839231443158980 ) ) ;
#33170=CARTESIAN_POINT ( 'NONE',  ( 20.66458278928015702, 17.76169105511801050, -4.999999999999998224 ) ) ;
#33174=CARTESIAN_POINT ( 'NONE',  ( 11.78077084959020482, -16.85122407151366986, -28.61443936225239426 ) ) ;
#33179=CARTESIAN_POINT ( 'NONE',  ( 13.44109819990983290, 22.91835836550887606, -15.43893112778157217 ) ) ;
#33181=CARTESIAN_POINT ( 'NONE',  ( -15.49750644015885115, 26.39995258097018649, -5.946129726914544555 ) ) ;
#33183=DIRECTION ( 'NONE',  ( 0.000000000000000000, 0.000000000000000000, 1.000000000000000000 ) ) ;
#33184=CARTESIAN_POINT ( 'NONE',  ( 11.26998537048577909, 17.69417195558794376, -26.23399489620831915 ) ) ;
#33186=CARTESIAN_POINT ( 'NONE',  ( 32.49036733324588511, -19.22569735934472135, -7.970791907112693586 ) ) ;
#33188=ORIENTED_EDGE ( 'NONE', *, *, #485, .F. ) ;
#33189=CARTESIAN_POINT ( 'NONE',  ( -12.07266892161228355, 20.90528892331724720, -19.43091586989769226 ) ) ;
#33191=CARTESIAN_POINT ( 'NONE',  ( -18.36895873238599108, -27.24750037505589262, -5.462138457986313256 ) ) ;
#33194=CARTESIAN_POINT ( 'NONE',  ( -29.06794499706158419, -9.974587258729167516, -14.80302332772542506 ) ) ;
#33195=CARTESIAN_POINT ( 'NONE',  ( -10.03238663440694189, -19.23125872514161117, -23.87728478131429100 ) ) ;
#33198=CARTESIAN_POINT ( 'NONE',  ( 23.21163472181913434, 2.226247987215279167, -19.68527219316008114 ) ) ;
#33201=VERTEX_POINT ( 'NONE', #5222 ) ;
#33202=CARTESIAN_POINT ( 'NONE',  ( -29.89510730381624271, -0.05789195541120888133, -9.702364829962164094 ) ) ;
#33205=CARTESIAN_POINT ( 'NONE',  ( 30.37910132873993874, -0.8766162490441101740, -10.11428594850108631 ) ) ;
#33212=CARTESIAN_POINT ( 'NONE',  ( -20.18092276982249444, 3.603208870470906433, -29.99999999999999645 ) ) ;
#33222=CARTESIAN_POINT ( 'NONE',  ( -19.92127511057237754, 5.002871685069139929, -28.81673539866426026 ) ) ;
#33225=CARTESIAN_POINT ( 'NONE',  ( 22.69918949349588289, -23.64247662620741153, -12.09428551148041997 ) ) ;
#33230=CARTESIAN_POINT ( 'NONE',  ( 15.21602949246752878, 27.19738721321897046, -6.408861906063099134 ) ) ;
#33234=CARTESIAN_POINT ( 'NONE',  ( -16.49044098933246971, 22.78194265982236999, -7.375859867825446337 ) ) ;
#33237=CARTESIAN_POINT ( 'NONE',  ( 15.24558589560055921, 26.36101825730073500, -7.828016443727952023 ) ) ;
#33241=CARTESIAN_POINT ( 'NONE',  ( -13.12858674853676533, 22.38440377439352247, -16.42546611361683162 ) ) ;
#33243=CARTESIAN_POINT ( 'NONE',  ( -15.27160128745916978, -26.39939704235120033, -7.827145747842149781 ) ) ;
#33245=CARTESIAN_POINT ( 'NONE',  ( -20.71396996789364309, -11.66691485040002618, -21.83546244019694171 ) ) ;
#33246=CARTESIAN_POINT ( 'NONE',  ( -5.633083642327312290, -21.97579894125815514, -18.92636197450212165 ) ) ;
#33248=CARTESIAN_POINT ( 'NONE',  ( 16.04266474709265466, 24.30463473437875876, -6.894355676570810054 ) ) ;
#33250=CARTESIAN_POINT ( 'NONE',  ( 22.76663162612608815, 7.095554964298814049, -14.84575477948635047 ) ) ;
#33251=CARTESIAN_POINT ( 'NONE',  ( 12.05833259093393117, 18.99598562053712314, -30.00000000000000000 ) ) ;
#33256=CARTESIAN_POINT ( 'NONE',  ( -27.65556173257783712, -0.4991889210311690195, -14.39343928979999454 ) ) ;
#33258=CARTESIAN_POINT ( 'NONE',  ( 30.96479225765983045, -0.1042645752839200801, -4.999999999999999112 ) ) ;
#33268=DIRECTION ( 'NONE',  ( -1.000000000000000000, 0.000000000000000000, 0.000000000000000000 ) ) ;
#33271=CARTESIAN_POINT ( 'NONE',  ( 1.495161097472319733, 36.13038531284369981, -10.17381497340915253 ) ) ;
#33280=CARTESIAN_POINT ( 'NONE',  ( 9.553997640115609258, 18.14112040201965925, -29.31786277955754016 ) ) ;
#33284=CARTESIAN_POINT ( 'NONE',  ( -19.20284012471338642, 16.64839643360665633, -4.999999999999998224 ) ) ;
#33287=CARTESIAN_POINT ( 'NONE',  ( 11.20545772873020773, -20.46486250540106155, -20.53879684372101266 ) ) ;
#33289=CARTESIAN_POINT ( 'NONE',  ( 15.22079284100554020, 26.44578639166762812, -7.826464274378870378 ) ) ;
#33290=CARTESIAN_POINT ( 'NONE',  ( -18.69487370500357670, 22.45507383323637995, -5.000000000000000000 ) ) ;
#33292=CARTESIAN_POINT ( 'NONE',  ( -26.67886893852930541, -22.27379109059698337, -11.10442598990957208 ) ) ;
#33293=CARTESIAN_POINT ( 'NONE',  ( 1.787030523841364404, -24.53966749997911379, -8.409682478326351074 ) ) ;
#33294=CARTESIAN_POINT ( 'NONE',  ( 11.24783307583270542, 17.38369397674119909, -27.46121733726331016 ) ) ;
#33295=CARTESIAN_POINT ( 'NONE',  ( 17.97214472351401326, 10.06683318593142396, -27.73766613656769309 ) ) ;
#33297=CARTESIAN_POINT ( 'NONE',  ( -4.351811147998932761, 21.49055966318188382, -24.33120353158464155 ) ) ;
#33305=CYLINDRICAL_SURFACE ( 'NONE', #16761, 18.00000000000002842 ) ;
#33306=CARTESIAN_POINT ( 'NONE',  ( -30.43551396330494185, 0.4041362800276669942, -5.946213268253427664 ) ) ;
#33307=CARTESIAN_POINT ( 'NONE',  ( 32.74700643712070303, -9.834764673945183944, -11.13845360772282511 ) ) ;
#33322=CARTESIAN_POINT ( 'NONE',  ( 16.34210300462141774, 12.63939967215257276, -27.15615485920570649 ) ) ;
#33324=CARTESIAN_POINT ( 'NONE',  ( 8.877500795550918866, 25.05368196378992351, -17.91181479415199718 ) ) ;
#33326=CARTESIAN_POINT ( 'NONE',  ( -18.72697364270403497, 8.503055164644706565, -28.29311283217969830 ) ) ;
#33331=CARTESIAN_POINT ( 'NONE',  ( 11.91525068712948254, -20.93073338464350641, -19.44990459973941910 ) ) ;
#33334=CARTESIAN_POINT ( 'NONE',  ( 22.40982762235196901, 2.618079236896951656, -30.00000000000000355 ) ) ;
#33335=CARTESIAN_POINT ( 'NONE',  ( -15.09589218995242099, 26.15653917439733434, -8.766821195319815629 ) ) ;
#33337=CARTESIAN_POINT ( 'NONE',  ( -23.49851162867760834, -26.24496101125836489, -7.634993703461408820 ) ) ;
#33338=CARTESIAN_POINT ( 'NONE',  ( 9.722871408072341737, -20.24786012184059203, -21.74715278292957521 ) ) ;
#33343=CARTESIAN_POINT ( 'NONE',  ( -7.187532856906145184, 19.54428593781422663, -27.17658705043585954 ) ) ;
#33349=CARTESIAN_POINT ( 'NONE',  ( 20.60629022519899323, 0.9185454123476016752, -28.08089029072296228 ) ) ;
#33353=CARTESIAN_POINT ( 'NONE',  ( -24.54801195516354184, 0.4553628621481798922, -18.45485564081276664 ) ) ;
#33356=CARTESIAN_POINT ( 'NONE',  ( 22.04779665452936044, -3.160493293077858201, -23.41725161139969558 ) ) ;
#33359=ORIENTED_EDGE ( 'NONE', *, *, #8910, .F. ) ;
#33361=ADVANCED_FACE ( 'NONE', ( #31589 ), #12314, .T. ) ;
#33363=CARTESIAN_POINT ( 'NONE',  ( -31.47283671532259675, -25.12609584734821411, -5.000000000000013323 ) ) ;
#33370=CARTESIAN_POINT ( 'NONE',  ( 8.094956495243176064, 35.93012217760205118, -7.153226857005175354 ) ) ;
#33375=CARTESIAN_POINT ( 'NONE',  ( 17.41019067503492579, -24.19678871709856338, -13.24119691528997578 ) ) ;
#33381=CARTESIAN_POINT ( 'NONE',  ( 10.93429579500015159, 17.39409148898324986, -28.70396595981947385 ) ) ;
#33384=CARTESIAN_POINT ( 'NONE',  ( -14.25035268484812079, 23.42487517527639795, -13.53819545498157240 ) ) ;
#33386=ADVANCED_FACE ( 'NONE', ( #10060, #31006 ), #34055, .T. ) ;
#33388=CARTESIAN_POINT ( 'NONE',  ( 11.56427562401083797, 18.36828347780292958, -23.86608368699767979 ) ) ;
#33391=CARTESIAN_POINT ( 'NONE',  ( 32.30856083864753714, -20.47190428664634609, -6.697067119202526619 ) ) ;
#33393=CARTESIAN_POINT ( 'NONE',  ( -12.40092118849391589, 21.42237501319575443, -18.39783089657061055 ) ) ;
#33395=CARTESIAN_POINT ( 'NONE',  ( -10.20341636066711288, -17.78360352085077878, -29.99999999999999645 ) ) ;
#33396=DIRECTION ( 'NONE',  ( -0.000000000000000000, -0.000000000000000000, -1.000000000000000000 ) ) ;
#33398=CARTESIAN_POINT ( 'NONE',  ( -30.84121824956582714, -11.62399599295376973, -12.93016321018791892 ) ) ;
#33399=PRODUCT_DEFINITION_CONTEXT ( 'detailed design', #31140, 'design' ) ;
#33400=CARTESIAN_POINT ( 'NONE',  ( -9.442374748160709430, -18.42736121383703463, -27.46044148871083124 ) ) ;
#33403=CARTESIAN_POINT ( 'NONE',  ( 22.88331890279000547, 2.992971246632968096, -19.75484460905745365 ) ) ;
#33407=CARTESIAN_POINT ( 'NONE',  ( -30.95087757567503672, -0.08989953764334650266, -5.473884744044031692 ) ) ;
#33409=CARTESIAN_POINT ( 'NONE',  ( 31.81105852766241071, -1.386432505721455044, -7.313011137699476194 ) ) ;
#33413=CARTESIAN_POINT ( 'NONE',  ( -24.03416057413138063, 3.517989641964785363, -16.69879147254576424 ) ) ;
#33426=CARTESIAN_POINT ( 'NONE',  ( -25.12800499762355599, 6.178422606789070848, -8.856332134561709424 ) ) ;
#33429=CARTESIAN_POINT ( 'NONE',  ( 25.25565081207486884, -26.17063864068946444, -5.878154196310728885 ) ) ;
#33432=CARTESIAN_POINT ( 'NONE',  ( 15.07890253828262672, 26.90834617882325830, -7.811347429530628439 ) ) ;
#33435=CARTESIAN_POINT ( 'NONE',  ( -14.97475431996716466, 18.42973550644392233, -17.73616635726436286 ) ) ;
#33437=CARTESIAN_POINT ( 'NONE',  ( 19.48557158514975285, -11.24999999999995737, 10.00000000000000000 ) ) ;
#33438=CARTESIAN_POINT ( 'NONE',  ( 15.35012758518023723, 26.57588627132344783, -6.887990273041626921 ) ) ;
#33440=CARTESIAN_POINT ( 'NONE',  ( 11.68691289177315085, 18.91070414389386656, -22.73532874761467326 ) ) ;
#33442=CARTESIAN_POINT ( 'NONE',  ( -15.03952492485649550, 26.34161984541752588, -8.758635656526267965 ) ) ;
#33444=CARTESIAN_POINT ( 'NONE',  ( -9.744066905365848186, -18.41592494163657889, -26.82585431338213411 ) ) ;
#33447=CARTESIAN_POINT ( 'NONE',  ( -33.58157224492879322, -18.91014262129728962, -5.435336751253355025 ) ) ;
#33448=CARTESIAN_POINT ( 'NONE',  ( -11.53315257097601254, -25.74693630043225667, -6.423746070632376792 ) ) ;
#33450=CARTESIAN_POINT ( 'NONE',  ( 13.89352154402242334, 21.03800918229289252, -16.54585482098419646 ) ) ;
#33452=CARTESIAN_POINT ( 'NONE',  ( 19.65936727364617198, 6.642930537632695476, -26.56611033146918999 ) ) ;
#33458=CARTESIAN_POINT ( 'NONE',  ( -20.49507156785942641, -0.4678258087238867380, -29.32393442354705471 ) ) ;
#33459=CARTESIAN_POINT ( 'NONE',  ( 30.54358385272748677, -0.07321200605768496406, -7.825060034502334894 ) ) ;
#33471=CARTESIAN_POINT ( 'NONE',  ( 1.533581810152732761, 37.14075507769783258, -8.844061256007341498 ) ) ;
#33479=CARTESIAN_POINT ( 'NONE',  ( 9.864563461025730007, 18.03425384675588816, -28.65979497051309721 ) ) ;
#33483=CARTESIAN_POINT ( 'NONE',  ( -15.97641923477408454, 13.01946753566105919, -27.71082971353359170 ) ) ;
#33488=CARTESIAN_POINT ( 'NONE',  ( 15.44845846858325267, -26.70665584896979183, -5.946081595203406955 ) ) ;
#33489=CARTESIAN_POINT ( 'NONE',  ( 14.84111742463143813, 25.60591702902538813, -10.18041830445565843 ) ) ;
#33490=CARTESIAN_POINT ( 'NONE',  ( 11.05073784553093219, 17.51747009666078725, -27.44606399619430448 ) ) ;
#33495=CARTESIAN_POINT ( 'NONE',  ( -26.00859912514732741, -20.40482213449253379, -12.92116335214409162 ) ) ;
#33496=CARTESIAN_POINT ( 'NONE',  ( -2.510360893402116655, -24.33974617660730289, -9.887043164262214745 ) ) ;
#33497=CARTESIAN_POINT ( 'NONE',  ( 14.77156457488188934, 24.32677381516164061, -11.61821993547884802 ) ) ;
#33498=CARTESIAN_POINT ( 'NONE',  ( 21.63088251164382214, 12.03979545591979772, -5.967650224983321650 ) ) ;
#33500=B_SPLINE_CURVE_WITH_KNOTS ( 'NONE', 3,
 ( #27632, #3647, #24984, #28230, #31283, #28426, #18497, #9946, #9351, #5896, #18299, #34138, #40015, #12594, #12193, #9149, #6289, #31087 ),
 .UNSPECIFIED., .F., .F.,
 ( 4, 2, 2, 2, 2, 2, 2, 2, 4 ),
 ( 0.000000000000000000, 0.1250000000000001943, 0.2500000000000001665, 0.3750000000000001110, 0.5000000000000001110, 0.6250000000000001110, 0.7500000000000000000, 0.8750000000000000000, 1.000000000000000000 ),
 .UNSPECIFIED. ) ;
#33501=CARTESIAN_POINT ( 'NONE',  ( -3.299821718920390001, 23.43477659572061711, -21.89659664273044370 ) ) ;
#33507=CARTESIAN_POINT ( 'NONE',  ( -20.80513200209605884, 0.9511744672526275535, -26.83982028479031356 ) ) ;
#33509=CARTESIAN_POINT ( 'NONE',  ( 30.13983096139770979, -9.052337329862529813, -13.90091081929475081 ) ) ;
#33523=CARTESIAN_POINT ( 'NONE',  ( 21.99787872679462808, -16.91788285020105675, -17.63963683105944824 ) ) ;
#33525=CARTESIAN_POINT ( 'NONE',  ( 19.91164419919741846, 14.82880737701476548, -7.913098018804059386 ) ) ;
#33526=CARTESIAN_POINT ( 'NONE',  ( 11.10948248300046082, 31.49357332391675968, -10.33061176195978170 ) ) ;
#33527=ORIENTED_EDGE ( 'NONE', *, *, #26093, .T. ) ;
#33528=CARTESIAN_POINT ( 'NONE',  ( -21.41702733524243030, 11.56821114029789754, -9.888691875779725748 ) ) ;
#33530=CARTESIAN_POINT ( 'NONE',  ( -36.48557158514989140, -11.24999999999987743, 10.00000000000000000 ) ) ;
#33532=CARTESIAN_POINT ( 'NONE',  ( 10.96665850233910966, -19.96023790109854090, -21.59991616212109733 ) ) ;
#33534=CARTESIAN_POINT ( 'NONE',  ( 19.69645987729881043, 11.37175641224107814, -21.56489709563629376 ) ) ;
#33535=CARTESIAN_POINT ( 'NONE',  ( -14.51563583855034878, 25.01866666866954603, -11.59546205423767873 ) ) ;
#33536=CIRCLE ( 'NONE', #3642, 18.00000000000000355 ) ;
#33537=CARTESIAN_POINT ( 'NONE',  ( -14.90132355581796730, -16.76330623373688411, -23.29508989526930662 ) ) ;
#33538=CARTESIAN_POINT ( 'NONE',  ( 13.35370518262597983, -25.77141642152969325, -8.785306460286980368 ) ) ;
#33542=CARTESIAN_POINT ( 'NONE',  ( -6.109668991155474238, 20.41692942102680419, -25.77087616168875783 ) ) ;
#33547=CARTESIAN_POINT ( 'NONE',  ( 24.53203630004508184, 0.4888770433563241480, -18.45847561789426550 ) ) ;
#33551=CARTESIAN_POINT ( 'NONE',  ( -27.73675306567175269, 0.1912042389513601559, -13.51357499948137963 ) ) ;
#33554=CARTESIAN_POINT ( 'NONE',  ( 20.45176271469480866, -2.234166952769147230, -28.59864995799237164 ) ) ;
#33560=CARTESIAN_POINT ( 'NONE',  ( 0.000000000000000000, 22.50000000000000355, 10.00000000000000000 ) ) ;
#33567=CARTESIAN_POINT ( 'NONE',  ( 3.279674764711696611, 20.24540435116753301, -30.00000000000000000 ) ) ;
#33570=CARTESIAN_POINT ( 'NONE',  ( 13.78700921972296811, -18.31297507672437774, -22.32604137707055969 ) ) ;
#33573=DIRECTION ( 'NONE',  ( -1.000000000000000000, 0.000000000000000000, 0.000000000000000000 ) ) ;
#33574=VERTEX_POINT ( 'NONE', #22844 ) ;
#33575=CARTESIAN_POINT ( 'NONE',  ( 15.20466363552954014, 26.50075720148702985, -7.824641958460332170 ) ) ;
#33577=CARTESIAN_POINT ( 'NONE',  ( -12.53910291074082295, 20.29581086541950441, -19.52226377206912034 ) ) ;
#33579=CARTESIAN_POINT ( 'NONE',  ( 13.62263039894608774, -24.10683431214565431, -13.51722375663292830 ) ) ;
#33581=CARTESIAN_POINT ( 'NONE',  ( 14.09135169103296725, 23.79168831276296103, -13.52014011376467373 ) ) ;
#33583=CARTESIAN_POINT ( 'NONE',  ( 21.28379295669234139, -14.39448103213696228, -19.64396054145414183 ) ) ;
#33584=ORIENTED_EDGE ( 'NONE', *, *, #3997, .T. ) ;
#33585=CARTESIAN_POINT ( 'NONE',  ( -14.77784559536929443, 28.35253144409951176, -6.851657844549249532 ) ) ;
#33587=CARTESIAN_POINT ( 'NONE',  ( -13.11275354201897692, -20.03949469003612904, -20.29527925755206752 ) ) ;
#33592=CARTESIAN_POINT ( 'NONE',  ( -20.01100984268285288, -7.597414617152628225, -25.63648934281255976 ) ) ;
#33593=CARTESIAN_POINT ( 'NONE',  ( -14.74418213917750364, -26.06945053339236296, -8.770932666061078464 ) ) ;
#33596=CARTESIAN_POINT ( 'NONE',  ( 28.51836663967885599, 2.011535347156353737, -8.319471814027734169 ) ) ;
#33601=CARTESIAN_POINT ( 'NONE',  ( -20.69976415826234373, 0.7537836665104515887, -27.44232068374074274 ) ) ;
#33603=CARTESIAN_POINT ( 'NONE',  ( 23.54702740617528178, -0.1080853855451005679, -20.45226996084934257 ) ) ;
#33608=CARTESIAN_POINT ( 'NONE',  ( -22.64987897201472933, 3.535174575633820204, -19.80251213055704440 ) ) ;
#33609=DIRECTION ( 'NONE',  ( -1.000000000000000000, 0.000000000000000000, 0.000000000000000000 ) ) ;
#33621=CARTESIAN_POINT ( 'NONE',  ( -23.68415675949719557, 7.936142738517225403, -9.861203543945475047 ) ) ;
#33624=CARTESIAN_POINT ( 'NONE',  ( 23.74789423688137546, -24.71003432651541587, -10.27501004622590131 ) ) ;
#33627=CARTESIAN_POINT ( 'NONE',  ( 15.34186426957387184, 27.04214388478009923, -5.000000000000000888 ) ) ;
#33631=CARTESIAN_POINT ( 'NONE',  ( -16.18955875647491993, 22.24348330894682135, -9.768321104223245399 ) ) ;
#33636=CARTESIAN_POINT ( 'NONE',  ( 11.32363492297296759, 18.02741897415885930, -25.01640571929745605 ) ) ;
#33640=CARTESIAN_POINT ( 'NONE',  ( -15.37369053509020667, 26.93276585663874556, -5.473472025586896272 ) ) ;
#33642=CARTESIAN_POINT ( 'NONE',  ( -15.16696621437007764, -26.16659013829510627, -8.764073972218964670 ) ) ;
#33644=CARTESIAN_POINT ( 'NONE',  ( -33.54211376200377259, -17.56714898150389104, -7.545851557378520980 ) ) ;
#33645=CARTESIAN_POINT ( 'NONE',  ( -7.605472735516510596, -19.34647446169307727, -26.98872577642229587 ) ) ;
#33647=CARTESIAN_POINT ( 'NONE',  ( 16.29902410653496148, 23.87181549541910641, -5.000000000000001776 ) ) ;
#33649=CARTESIAN_POINT ( 'NONE',  ( 24.29960814844372408, 7.334394940551312025, -8.871400124960164391 ) ) ;
#33654=CARTESIAN_POINT ( 'NONE',  ( -20.74261079067644786, -0.4953610022129137924, -27.36091918602213013 ) ) ;
#33655=CARTESIAN_POINT ( 'NONE',  ( 30.92694434159519901, -0.1013669071028381469, -5.945198762247071222 ) ) ;
#33657=DIRECTION ( 'NONE',  ( 1.000000000000000000, 0.000000000000000000, 0.000000000000000000 ) ) ;
#33661=CARTESIAN_POINT ( 'NONE',  ( 19.79815887584821610, 19.84782313723624370, -13.42901749168597192 ) ) ;
#33668=CARTESIAN_POINT ( 'NONE',  ( 3.867670317776020994, 37.97392467330134735, -5.858600071952766442 ) ) ;
#33674=CARTESIAN_POINT ( 'NONE',  ( 14.23945615837883949, -31.58416516429907972, 0.000000000000000000 ) ) ;
#33675=AXIS2_PLACEMENT_3D ( 'NONE', #29016, #29420, #13572 ) ;
#33676=CARTESIAN_POINT ( 'NONE',  ( 11.27257766325769239, 20.01675547985872683, -21.50247975293300584 ) ) ;
#33680=CARTESIAN_POINT ( 'NONE',  ( -19.16847334494743649, 16.60965121416508339, -6.446626008538204111 ) ) ;
#33683=CARTESIAN_POINT ( 'NONE',  ( 14.85648237307818498, -25.82965647359291950, -9.709266928100928951 ) ) ;
#33684=EDGE_CURVE ( 'NONE', #31289, #6084, #13296, .T. ) ;
#33685=CARTESIAN_POINT ( 'NONE',  ( -17.96239324037909668, -22.68179410725907275, -15.04167774667985569 ) ) ;
#33686=FACE_OUTER_BOUND ( 'NONE', #685, .T. ) ;
#33688=CARTESIAN_POINT ( 'NONE',  ( 12.11672168374641956, 19.94100266206895711, -20.53805629048271797 ) ) ;
#33692=CARTESIAN_POINT ( 'NONE',  ( -20.97423577176458309, -16.41428094411201499, -18.66848081662921999 ) ) ;
#33693=CARTESIAN_POINT ( 'NONE',  ( -0.3884064831159054210, -24.73345553465953017, -6.453633902575101722 ) ) ;
#33694=CARTESIAN_POINT ( 'NONE',  ( 15.46285928058480152, 25.94289359300809750, -7.360000718803358488 ) ) ;
#33695=CARTESIAN_POINT ( 'NONE',  ( 18.90977336216788629, 11.58301458159701092, -19.06584539304483528 ) ) ;
#33697=CARTESIAN_POINT ( 'NONE',  ( -3.891894238164187225, 27.44735175141750716, -17.64614778283444352 ) ) ;
#33699=CARTESIAN_POINT ( 'NONE',  ( -32.83126665819848711, -6.129261575006776930, -10.33078432171702055 ) ) ;
#33704=CARTESIAN_POINT ( 'NONE',  ( -29.22879574628063182, 0.6855083203516167956, -9.721972840624630408 ) ) ;
#33706=CARTESIAN_POINT ( 'NONE',  ( 20.07302653732184439, -7.417995268840763323, -25.64353969630302998 ) ) ;
#33720=CARTESIAN_POINT ( 'NONE',  ( -3.059748728390603745, 38.05383510088704213, -6.278958135869814328 ) ) ;
#33724=CARTESIAN_POINT ( 'NONE',  ( 24.61464500862492244, -18.95959619293818577, -14.76315794208474053 ) ) ;
#33725=CARTESIAN_POINT ( 'NONE',  ( 18.72885360190822368, 15.10340418431515097, -12.86103651079863930 ) ) ;
#33726=CARTESIAN_POINT ( 'NONE',  ( 6.972563247160245226, 19.50015755702453291, -27.85944964339131857 ) ) ;
#33728=CARTESIAN_POINT ( 'NONE',  ( -18.87236092649526142, 8.549343831987949116, -26.60993495225021732 ) ) ;
#33730=CARTESIAN_POINT ( 'NONE',  ( 14.16900449820494678, -24.63218968044553847, -12.54074064262510291 ) ) ;
#33734=CARTESIAN_POINT ( 'NONE',  ( 12.05832241004688399, 18.99596958976722760, -30.00000000000000000 ) ) ;
#33736=CARTESIAN_POINT ( 'NONE',  ( -11.05339688301675594, 17.51568747190060904, -27.44627114179852256 ) ) ;
#33738=CARTESIAN_POINT ( 'NONE',  ( -13.46176099346681809, -16.14434513549814909, -26.50464527480163213 ) ) ;
#33739=CARTESIAN_POINT ( 'NONE',  ( 11.40532025035704677, -23.47631050763437344, -14.58224395303332699 ) ) ;
#33744=CARTESIAN_POINT ( 'NONE',  ( -6.672699392047024780, 22.34245898429709598, -22.09591057274325365 ) ) ;
#33749=CARTESIAN_POINT ( 'NONE',  ( 25.84101663196772947, 0.3562117509880242672, -16.44710462539339346 ) ) ;
#33751=CARTESIAN_POINT ( 'NONE',  ( 19.48557158514982746, -11.25000000000009415, 0.000000000000000000 ) ) ;
#33753=CARTESIAN_POINT ( 'NONE',  ( -20.52702548769616442, 0.8561983801584475140, -28.70691147235546836 ) ) ;
#33757=CARTESIAN_POINT ( 'NONE',  ( 29.73061004676158348, -5.254439166030093311, -14.04169227091120042 ) ) ;
#33762=DIRECTION ( 'NONE',  ( 0.000000000000000000, 0.000000000000000000, 1.000000000000000000 ) ) ;
#33770=CARTESIAN_POINT ( 'NONE',  ( 4.056192851408421340, 20.98781719672311397, -25.66352865187444365 ) ) ;
#33772=CARTESIAN_POINT ( 'NONE',  ( 16.51452683366346363, -26.94346954434094243, -5.935747864356960335 ) ) ;
#33773=CARTESIAN_POINT ( 'NONE',  ( 75.15099915297797395, 43.38844959084117647, 0.000000000000000000 ) ) ;
#33777=CARTESIAN_POINT ( 'NONE',  ( -15.42498320908520704, 26.75103934920171511, -5.474196440071953162 ) ) ;
#33780=CARTESIAN_POINT ( 'NONE',  ( 12.42243934462404553, -22.55512267161180517, -16.46144506859675261 ) ) ;
#33782=EDGE_LOOP ( 'NONE', ( #23890, #2963, #37661, #5970 ) ) ;
#33784=CARTESIAN_POINT ( 'NONE',  ( -14.15606045317429462, 26.98637277077674312, -10.55315924151954121 ) ) ;
#33786=CARTESIAN_POINT ( 'NONE',  ( -18.79972725875673234, -26.44331049119935173, -9.081311273665734873 ) ) ;
#33790=CARTESIAN_POINT ( 'NONE',  ( -20.21455581687538228, -6.984773374644928978, -25.66161433552150584 ) ) ;
#33791=CARTESIAN_POINT ( 'NONE',  ( -14.53915841217452787, -25.76227397208802117, -9.714023261601081316 ) ) ;
#33794=CARTESIAN_POINT ( 'NONE',  ( 30.59650344009811462, 0.1707353974115741191, -6.417298568035493034 ) ) ;
#33799=CARTESIAN_POINT ( 'NONE',  ( -22.23634261291865855, 0.6022514368306863819, -22.72707163159650534 ) ) ;
#33801=CARTESIAN_POINT ( 'NONE',  ( 31.01104622761054230, -0.9322571436193676231, -8.717104344044161124 ) ) ;
#33805=CARTESIAN_POINT ( 'NONE',  ( -26.85005620991422859, 2.655769742037339398, -11.69190580713203964 ) ) ;
#33806=CARTESIAN_POINT ( 'NONE',  ( 17.34253826539385201, 27.32041144647958575, -13.70816084473008800 ) ) ;
#33815=CARTESIAN_POINT ( 'NONE',  ( -21.57472102895474109, 6.664260218504890254, -18.95869221603280153 ) ) ;
#33818=CARTESIAN_POINT ( 'NONE',  ( 14.77033916382619694, -15.37368051247184120, -25.75951637363165148 ) ) ;
#33821=CARTESIAN_POINT ( 'NONE',  ( 15.32541171586220941, 27.00755533933892139, -5.943389983610922300 ) ) ;
#33823=CARTESIAN_POINT ( 'NONE',  ( -15.23324207282226261, 23.13468747206823650, -11.65450899073664814 ) ) ;
#33827=CARTESIAN_POINT ( 'NONE',  ( 14.30395659009414011, 24.43853900399440704, -12.55159526015550675 ) ) ;
#33828=EDGE_LOOP ( 'NONE', ( #10232, #22989 ) ) ;
#33829=CYLINDRICAL_SURFACE ( 'NONE', #19008, 18.00000000000001421 ) ;
#33830=ORIENTED_EDGE ( 'NONE', *, *, #14464, .F. ) ;
#33831=CARTESIAN_POINT ( 'NONE',  ( -10.97252080025042353, 17.71808212118776638, -26.81605910367778023 ) ) ;
#33833=CARTESIAN_POINT ( 'NONE',  ( -9.580852559982135475, -18.12344168749379492, -29.34663924488240738 ) ) ;
#33835=CARTESIAN_POINT ( 'NONE',  ( -33.84414506509371989, -17.72909435222108598, -6.697593496457613149 ) ) ;
#33836=CARTESIAN_POINT ( 'NONE',  ( -11.46491240625375951, -25.63296783226419251, -7.374722599587664185 ) ) ;
#33838=CARTESIAN_POINT ( 'NONE',  ( 12.11158980248019645, 16.54297856518634902, -30.00000000000000000 ) ) ;
#33839=EDGE_CURVE ( 'NONE', #2968, #9588, #14513, .T. ) ;
#33841=CARTESIAN_POINT ( 'NONE',  ( 19.44092958653124725, 6.613309545252517019, -28.84111800654028457 ) ) ;
#33848=CARTESIAN_POINT ( 'NONE',  ( -31.38524255402332841, -1.184009006764249472, -8.242489630512061183 ) ) ;
#33849=CARTESIAN_POINT ( 'NONE',  ( 20.97531576542675680, 0.7517682979586068903, -26.21993259525444842 ) ) ;
#33854=CARTESIAN_POINT ( 'NONE',  ( 17.34253826539385201, 27.32041144647958575, -13.70816084473008800 ) ) ;
#33859=CIRCLE ( 'NONE', #22820, 18.00000000000000000 ) ;
#33861=FACE_OUTER_BOUND ( 'NONE', #28665, .T. ) ;
#33862=CARTESIAN_POINT ( 'NONE',  ( 3.399496789611879066, 33.07784035496857200, -12.90587768247559275 ) ) ;
#33868=CARTESIAN_POINT ( 'NONE',  ( 13.09714986319504781, 23.57938164331712372, -15.36463189380894612 ) ) ;
#33871=CARTESIAN_POINT ( 'NONE',  ( -18.64675247270446334, 17.55525769010250059, -7.410062710081297688 ) ) ;
#33875=CARTESIAN_POINT ( 'NONE',  ( 11.54455564027605163, -20.97676539060953615, -19.49701577318683832 ) ) ;
#33876=CARTESIAN_POINT ( 'NONE',  ( -13.59760052849660461, -18.39269962030116190, -22.34963271257799633 ) ) ;
#33878=CARTESIAN_POINT ( 'NONE',  ( 15.22536027402585646, 26.43007570565260522, -7.826986632856818282 ) ) ;
#33882=CARTESIAN_POINT ( 'NONE',  ( -14.89343483659701661, -25.97116541732223283, -9.239377617673552479 ) ) ;
#33884=CARTESIAN_POINT ( 'NONE',  ( -28.56121237968124049, -23.79504838712581360, -7.568206030601050571 ) ) ;
#33885=CARTESIAN_POINT ( 'NONE',  ( 1.236634163872074366, -20.51914614933548719, -30.00000000000001066 ) ) ;
#33886=CARTESIAN_POINT ( 'NONE',  ( 13.22294849863610722, 21.18001974898340478, -17.48564420674206943 ) ) ;
#33887=CARTESIAN_POINT ( 'NONE',  ( 19.80460749329455084, 12.16438029996845493, -14.92251035621654331 ) ) ;
#33890=CARTESIAN_POINT ( 'NONE',  ( -3.458130042104727409, 20.20612265101129168, -29.22679435874877996 ) ) ;
#33892=CARTESIAN_POINT ( 'NONE',  ( -29.79436624158082481, -5.527400279271972749, -14.02904961299980791 ) ) ;
#33897=CARTESIAN_POINT ( 'NONE',  ( -22.62160857727931784, 0.9731345702083473714, -21.66193316938567293 ) ) ;
#33898=CARTESIAN_POINT ( 'NONE',  ( 19.51071764920130391, -6.549296650950685361, -28.48338599449614605 ) ) ;
#33909=CARTESIAN_POINT ( 'NONE',  ( -2.908402701707879068, 35.88643271034062820, -10.18049541942522573 ) ) ;
#33913=CARTESIAN_POINT ( 'NONE',  ( 29.86472888556171768, -22.97618816406824749, -7.129344454106402829 ) ) ;
#33914=CARTESIAN_POINT ( 'NONE',  ( 16.23943293897244544, 12.53170227796935343, -29.42461426250243051 ) ) ;
#33915=CARTESIAN_POINT ( 'NONE',  ( 8.203324777427138059, 19.12455918632797491, -27.23712529939752969 ) ) ;
#33916=VERTEX_POINT ( 'NONE', #21801 ) ;
#33917=CARTESIAN_POINT ( 'NONE',  ( -18.67511144159872316, 8.486512637698147898, -30.00000000000000000 ) ) ;
#33919=CARTESIAN_POINT ( 'NONE',  ( 15.27392571247604103, -26.19117440705182176, -8.759444881256309046 ) ) ;
#33921=CARTESIAN_POINT ( 'NONE',  ( 13.28992586503610340, -18.25382200079949513, -29.99999999999999289 ) ) ;
#33924=CARTESIAN_POINT ( 'NONE',  ( -12.63209216405648405, 21.08522415426002539, -18.44753828729430367 ) ) ;
#33925=CARTESIAN_POINT ( 'NONE',  ( -21.98991108409586204, -24.65262130162854959, -11.21756587170641772 ) ) ;
#33926=CARTESIAN_POINT ( 'NONE',  ( 8.648529717685608631, -19.31184748484744773, -25.15118541177943712 ) ) ;
#33928=ORIENTED_EDGE ( 'NONE', *, *, #19463, .T. ) ;
#33929=CARTESIAN_POINT ( 'NONE',  ( -6.648157636961573580, 19.96354927932426548, -26.46540010809100707 ) ) ;
#33934=CARTESIAN_POINT ( 'NONE',  ( 30.78432895970654926, -0.02295136688160604593, -6.417004196556904461 ) ) ;
#33938=CARTESIAN_POINT ( 'NONE',  ( -30.84974397859977557, 0.01335361837341130647, -4.999999999999999112 ) ) ;
#33942=CARTESIAN_POINT ( 'NONE',  ( 32.74085591134507212, -5.827811756920110220, -10.33996608089739055 ) ) ;
#33950=EDGE_LOOP ( 'NONE', ( #33928, #37906 ) ) ;
#33951=( LENGTH_UNIT ( ) NAMED_UNIT ( * ) SI_UNIT ( .MILLI., .METRE. ) );
#33952=DIRECTION ( 'NONE',  ( 0.000000000000000000, 0.000000000000000000, 1.000000000000000000 ) ) ;
#33956=CARTESIAN_POINT ( 'NONE',  ( 9.852384739805275515, 34.25028444780376446, -8.049578315757582203 ) ) ;
#33959=CARTESIAN_POINT ( 'NONE',  ( 17.59916522844583753, -27.17459308133313201, -5.000000000000004441 ) ) ;
#33966=CARTESIAN_POINT ( 'NONE',  ( -13.06770973401748215, 21.42831458027773550, -17.46073772354927556 ) ) ;
#33969=CARTESIAN_POINT ( 'NONE',  ( 14.48426304913733986, -25.43374522747946287, -10.65622368699242628 ) ) ;
#33972=ORIENTED_EDGE ( 'NONE', *, *, #39802, .F. ) ;
#33974=CARTESIAN_POINT ( 'NONE',  ( -14.00751334334244191, 28.57779656496513354, -9.118724234240687565 ) ) ;
#33975=CARTESIAN_POINT ( 'NONE',  ( -11.86207838096284917, -17.26656891588605447, -26.63928184976938951 ) ) ;
#33980=CARTESIAN_POINT ( 'NONE',  ( -35.33786424633182577, -8.799366064169335644, -5.444321735654653160 ) ) ;
#33981=CARTESIAN_POINT ( 'NONE',  ( -9.365571907152105524, -18.46390408244730708, -27.46573865726494290 ) ) ;
#33984=CARTESIAN_POINT ( 'NONE',  ( 29.58057729095054000, 0.2898696450949133085, -9.714030781592626340 ) ) ;
#33988=CARTESIAN_POINT ( 'NONE',  ( -20.61180082990850693, 0.8259781403983986747, -28.07628969275633324 ) ) ;
#33990=CARTESIAN_POINT ( 'NONE',  ( 25.99411550134611559, -1.208840217080102031, -17.24439678332520742 ) ) ;
#33993=CARTESIAN_POINT ( 'NONE',  ( -19.48557158514998022, -11.24999999999982414, 3.000000000000000000 ) ) ;
#33996=CARTESIAN_POINT ( 'NONE',  ( -20.27181835515031949, 3.600595787728656738, -28.19117047517736196 ) ) ;
#34008=ORIENTED_EDGE ( 'NONE', *, *, #27998, .T. ) ;
#34009=CARTESIAN_POINT ( 'NONE',  ( -22.69837051162585695, 7.744818927720608315, -13.85387379231857352 ) ) ;
#34012=CARTESIAN_POINT ( 'NONE',  ( 23.81893702819105485, -26.18960064386696729, -7.628968477593851105 ) ) ;
#34015=CARTESIAN_POINT ( 'NONE',  ( 10.77342450413916630, 17.44087877699069367, -30.00000000000000000 ) ) ;
#34017=CARTESIAN_POINT ( 'NONE',  ( -16.03826714829968125, 24.67705000163143580, -5.000000000000000000 ) ) ;
#34021=CARTESIAN_POINT ( 'NONE',  ( 15.03218564788412515, 25.92419391550620844, -9.238870818048370737 ) ) ;
#34025=CARTESIAN_POINT ( 'NONE',  ( -13.10376629299052098, 22.42928523344748726, -16.41988283430683282 ) ) ;
#34027=CARTESIAN_POINT ( 'NONE',  ( -9.543759016413366325, -18.14299990126706419, -30.00000000000000000 ) ) ;
#34030=CARTESIAN_POINT ( 'NONE',  ( -34.32242099319713446, -16.67052798041778772, -6.699077853923277814 ) ) ;
#34032=CARTESIAN_POINT ( 'NONE',  ( -12.95816149891683011, -24.84176018504629369, -11.63896638183241983 ) ) ;
#34033=FACE_OUTER_BOUND ( 'NONE', #8780, .T. ) ;
#34034=CARTESIAN_POINT ( 'NONE',  ( 16.09876026818504968, 24.41207849431964405, -5.947509210907390376 ) ) ;
#34036=CARTESIAN_POINT ( 'NONE',  ( 20.29178992508080626, 5.227586473962275271, -25.37103639584170622 ) ) ;
#34039=CARTESIAN_POINT ( 'NONE',  ( -18.54826649988357090, -24.72227203017434150, -12.26027863146039820 ) ) ;
#34041=CARTESIAN_POINT ( 'NONE',  ( -28.92430414141464468, -0.6002475978605696927, -12.47730999436802790 ) ) ;
#34042=CARTESIAN_POINT ( 'NONE',  ( 20.49022872340270851, 0.6388713974194968337, -29.34434107258899971 ) ) ;
#34046=CARTESIAN_POINT ( 'NONE',  ( 19.54664213359407654, -11.28525909758385914, -30.00000000000003908 ) ) ;
#34053=DIRECTION ( 'NONE',  ( -1.000000000000000000, 0.000000000000000000, 0.000000000000000000 ) ) ;
#34054=CARTESIAN_POINT ( 'NONE',  ( 2.387565118073518011, 23.58149098553560563, -21.87002398248182899 ) ) ;
#34055=PLANE ( 'NONE',  #17903 ) ;
#34062=CARTESIAN_POINT ( 'NONE',  ( 14.69102536304534112, 26.94039611839157899, -9.191466769791299285 ) ) ;
#34065=CARTESIAN_POINT ( 'NONE',  ( -15.31736683468135141, 14.60021943509330100, -24.29952530214165662 ) ) ;
#34068=CARTESIAN_POINT ( 'NONE',  ( 11.55613727932546730, -20.97541504343049823, -19.49553383130734474 ) ) ;
#34069=CARTESIAN_POINT ( 'NONE',  ( -12.75218288797893074, -16.30376047647427029, -27.89448312604282165 ) ) ;
#34070=CARTESIAN_POINT ( 'NONE',  ( 19.48557158514988075, -11.24999999999998224, 6.000000000000000000 ) ) ;
#34071=CARTESIAN_POINT ( 'NONE',  ( 15.33017556631518552, 26.64601132140138517, -6.887373872617191140 ) ) ;
#34075=CARTESIAN_POINT ( 'NONE',  ( -13.94116916282742302, -24.59632506325680978, -12.55420017537907817 ) ) ;
#34078=CARTESIAN_POINT ( 'NONE',  ( -16.53721940376430055, -12.13086247549455443, -30.00000000000000355 ) ) ;
#34079=CARTESIAN_POINT ( 'NONE',  ( -2.588656999911660428, -24.74688003723862195, -6.453009911337188598 ) ) ;
#34080=CARTESIAN_POINT ( 'NONE',  ( 11.35289046387891609, 17.31125046002085099, -27.46915152833578233 ) ) ;
#34081=CARTESIAN_POINT ( 'NONE',  ( 21.45236543604948309, 10.76621870831805339, -11.87856902876374576 ) ) ;
#34084=CARTESIAN_POINT ( 'NONE',  ( -4.502816615928998623, 26.15216069617400763, -18.69540600892100812 ) ) ;
#34086=CARTESIAN_POINT ( 'NONE',  ( -22.76661381573873300, -4.191030258134940567, -22.19333013853839986 ) ) ;
#34091=CARTESIAN_POINT ( 'NONE',  ( -20.58891407026878895, 1.184266961143116470, -28.09387474696538689 ) ) ;
#34092=CARTESIAN_POINT ( 'NONE',  ( 35.19885548643981821, -12.96001660873345251, -6.713464945328998290 ) ) ;
#34103=FACE_OUTER_BOUND ( 'NONE', #16693, .T. ) ;
#34106=CARTESIAN_POINT ( 'NONE',  ( -1.922249852543706616, 38.37524763245696846, -5.856172595693201366 ) ) ;
#34107=CARTESIAN_POINT ( 'NONE',  ( -32.35383858704948778, -1.519079388896815930, -4.999999999999999112 ) ) ;
#34111=CARTESIAN_POINT ( 'NONE',  ( 23.89493199558969039, -19.57224858292615366, -14.78313763251888879 ) ) ;
#34112=CARTESIAN_POINT ( 'NONE',  ( 20.04635827611367205, 14.95022894506133859, -4.999999999999998224 ) ) ;
#34113=CARTESIAN_POINT ( 'NONE',  ( 13.65686006951314369, 30.58359301831817589, -6.811602640649293328 ) ) ;
#34115=CARTESIAN_POINT ( 'NONE',  ( -20.47881545949457660, 13.50965256804138370, -8.899456932346438975 ) ) ;
#34117=CARTESIAN_POINT ( 'NONE',  ( 15.66152395236884054, -26.76027550630084662, -5.944054962524266905 ) ) ;
#34118=DIRECTION ( 'NONE',  ( -0.000000000000000000, -0.000000000000000000, -1.000000000000000000 ) ) ;
#34119=CARTESIAN_POINT ( 'NONE',  ( 20.55563217186196212, -29.52600041847795254, -13.99876745781546994 ) ) ;
#34121=CARTESIAN_POINT ( 'NONE',  ( -14.01594577761574101, 23.96872618684867007, -13.51011200901672105 ) ) ;
#34122=CARTESIAN_POINT ( 'NONE',  ( -20.99987834568138823, -24.96315251019730397, -11.24918557064901847 ) ) ;
#34123=CARTESIAN_POINT ( 'NONE',  ( 9.433270209358736835, -23.35418427748271242, -14.68531594918982819 ) ) ;
#34125=EDGE_CURVE ( 'NONE', #33096, #648, #13363, .T. ) ;
#34129=CARTESIAN_POINT ( 'NONE',  ( -10.29501812418428308, 34.74514102979851060, -5.879665602947800274 ) ) ;
#34137=CARTESIAN_POINT ( 'NONE',  ( 30.31434325333418300, 0.03612907296712006971, -8.298080414836505270 ) ) ;
#34138=CARTESIAN_POINT ( 'NONE',  ( 6.749995343096087730, 37.10960504752365807, -5.000000000000000888 ) ) ;
#34142=CARTESIAN_POINT ( 'NONE',  ( -20.81343797531129880, 0.8557099860676852243, -26.83253627507455974 ) ) ;
#34145=CARTESIAN_POINT ( 'NONE',  ( 34.51621760006609207, -7.217447013052957772, -7.634130922725350210 ) ) ;
#34160=CARTESIAN_POINT ( 'NONE',  ( 5.122947202949493573, 19.93899402170990953, -28.50457462493328720 ) ) ;
#34162=CIRCLE ( 'NONE', #12747, 18.00000000000000000 ) ;
#34163=CARTESIAN_POINT ( 'NONE',  ( 17.59916522844583753, -27.17459308133313201, -5.464832681431312622 ) ) ;
#34164=( NAMED_UNIT ( * ) SI_UNIT ( $, .STERADIAN. ) SOLID_ANGLE_UNIT ( ) );
#34167=CARTESIAN_POINT ( 'NONE',  ( -12.04642914189274094, 19.21860882176112639, -21.64378893228296619 ) ) ;
#34169=CARTESIAN_POINT ( 'NONE',  ( 14.61363033921321986, -25.62685285069673924, -10.18295734475554681 ) ) ;
#34173=ORIENTED_EDGE ( 'NONE', *, *, #264, .F. ) ;
#34174=CARTESIAN_POINT ( 'NONE',  ( -13.68341986734493609, 30.02787314512316641, -7.720655657447415443 ) ) ;
#34175=CARTESIAN_POINT ( 'NONE',  ( -11.20940000001327341, -17.48797073134899094, -27.33040502637083691 ) ) ;
#34178=CARTESIAN_POINT ( 'NONE',  ( -34.53800058995564370, -9.629687233961918835, -8.469964886165900708 ) ) ;
#34179=CARTESIAN_POINT ( 'NONE',  ( -15.36059797614417022, -26.70982037388659691, -5.474171403654337631 ) ) ;
#34182=CARTESIAN_POINT ( 'NONE',  ( 21.99066440368976671, 1.589892210864482847, -22.84507827221558784 ) ) ;
#34186=CARTESIAN_POINT ( 'NONE',  ( -30.91582600597228137, -0.05403808547916669897, -5.000000000000000000 ) ) ;
#34188=CARTESIAN_POINT ( 'NONE',  ( 30.72234448700380938, -1.665297440091649372, -10.52892505583194449 ) ) ;
#34191=CARTESIAN_POINT ( 'NONE',  ( 12.20447399291898272, -16.48659499025950836, -29.99999999999999289 ) ) ;
#34194=CARTESIAN_POINT ( 'NONE',  ( -25.22597472235315053, 4.364516542823781542, -12.73472624478601034 ) ) ;
#34198=CARTESIAN_POINT ( 'NONE',  ( -19.48557158514988785, -11.24999999999987743, 6.000000000000000000 ) ) ;
#34204=CARTESIAN_POINT ( 'NONE',  ( -24.56734199138568897, 7.082464585399747214, -8.380301523606016545 ) ) ;
#34207=CARTESIAN_POINT ( 'NONE',  ( 23.08170797751215630, -26.79846190384431992, -5.889568152681599500 ) ) ;
#34209=CARTESIAN_POINT ( 'NONE',  ( 15.19751254492016734, 26.84389974300201587, -7.349166724040926191 ) ) ;
#34212=CARTESIAN_POINT ( 'NONE',  ( -15.79715600521433494, 23.30597418570086887, -9.749926740643289236 ) ) ;
#34216=CARTESIAN_POINT ( 'NONE',  ( 13.23037898294574966, 22.19842390109810992, -16.44731654887686290 ) ) ;
#34221=CARTESIAN_POINT ( 'NONE',  ( -13.64709611685704260, 23.66733992415775845, -14.44796888404773583 ) ) ;
#34224=CARTESIAN_POINT ( 'NONE',  ( -12.39674543852726174, -22.02096203800932273, -17.42484875458988469 ) ) ;
#34227=VERTEX_POINT ( 'NONE', #36116 ) ;
#34228=CARTESIAN_POINT ( 'NONE',  ( -22.18470991521814994, -10.78957402553765199, -20.70439974414385276 ) ) ;
#34229=CARTESIAN_POINT ( 'NONE',  ( -8.861892952964076642, -21.31740138737636059, -19.76521263307946441 ) ) ;
#34231=CARTESIAN_POINT ( 'NONE',  ( 12.43571604352363380, 16.42874407723720864, -28.15360703238361495 ) ) ;
#34233=CARTESIAN_POINT ( 'NONE',  ( 24.67187950889155346, 4.601540168446949686, -13.74189493147921759 ) ) ;
#34238=CARTESIAN_POINT ( 'NONE',  ( -30.70443338618256490, -0.3849243431390188541, -8.278649579022490101 ) ) ;
#34239=CARTESIAN_POINT ( 'NONE',  ( 28.53789851150272838, -0.1047529870928948365, -12.52552137319313807 ) ) ;
#34243=CARTESIAN_POINT ( 'NONE',  ( 20.55563217186196212, -29.52600041847795254, -13.99876745781546994 ) ) ;
#34250=CARTESIAN_POINT ( 'NONE',  ( 14.98890121934609532, -28.67928442654221044, -5.000000000000000000 ) ) ;
#34255=CARTESIAN_POINT ( 'NONE',  ( 2.729340787065954732, 38.05821448855805755, -6.699057688494861829 ) ) ;
#34262=CARTESIAN_POINT ( 'NONE',  ( 12.21266005302986279, 21.68539402877682676, -18.35945844235239832 ) ) ;
#34265=CARTESIAN_POINT ( 'NONE',  ( -15.49039487082849220, 13.58517199178181301, -27.69483034437292801 ) ) ;
#34268=CARTESIAN_POINT ( 'NONE',  ( 9.621585592044306523, -18.34052516761964213, -27.44776497733833764 ) ) ;
#34269=CARTESIAN_POINT ( 'NONE',  ( -22.30837096923181662, -26.42455506716093794, -8.094580056074205388 ) ) ;
#34270=CARTESIAN_POINT ( 'NONE',  ( 15.40143551928530741, 26.74272614036931373, -5.946164455718055741 ) ) ;
#34271=CARTESIAN_POINT ( 'NONE',  ( 14.73068410223729607, 25.41701562580275819, -10.65180837224440147 ) ) ;
#34274=CARTESIAN_POINT ( 'NONE',  ( -11.12516049792199269, -20.47921145105273411, -20.54846162138489873 ) ) ;
#34278=CARTESIAN_POINT ( 'NONE',  ( -29.47215113446729617, -21.71708447961223598, -9.294057262345292614 ) ) ;
#34279=CARTESIAN_POINT ( 'NONE',  ( -0.3144284205193551562, -22.16443700259523197, -19.06343410368202385 ) ) ;
#34280=CARTESIAN_POINT ( 'NONE',  ( 15.55086357314465495, 25.88735796154298541, -6.889558640719104510 ) ) ;
#34281=CARTESIAN_POINT ( 'NONE',  ( 19.55223183195777281, 9.929862210829575986, -20.11535475670744688 ) ) ;
#34282=CARTESIAN_POINT ( 'NONE',  ( 18.00000000000000000, 22.50000000000001421, 6.000000000000000000 ) ) ;
#34285=CARTESIAN_POINT ( 'NONE',  ( -33.40104146632486248, -3.480120356603942255, -6.360699399790051167 ) ) ;
#34291=CARTESIAN_POINT ( 'NONE',  ( -29.02761408569459434, 0.6971569698290208672, -10.19582416827852356 ) ) ;
#34292=CARTESIAN_POINT ( 'NONE',  ( 20.59519988482301756, -7.609356043779510692, -24.29945422642990849 ) ) ;
#34303=CARTESIAN_POINT ( 'NONE',  ( -2.518168780898724979, 31.12813172238224269, -14.74331629931110221 ) ) ;
#34310=CARTESIAN_POINT ( 'NONE',  ( 8.705524501264831017, 18.63857284810273285, -28.61403163583886666 ) ) ;
#34312=CARTESIAN_POINT ( 'NONE',  ( -18.40526182805578870, 10.96415812414948299, -22.25133746893234843 ) ) ;
#34314=CARTESIAN_POINT ( 'NONE',  ( 15.45591863128356991, -26.53792291655177138, -7.354334154706036131 ) ) ;
#34316=CARTESIAN_POINT ( 'NONE',  ( 15.07823932231967312, 26.21524158488056244, -8.764214361564787836 ) ) ;
#34317=CARTESIAN_POINT ( 'NONE',  ( -15.72991998290134141, -16.18894361744923316, -20.11584339644716479 ) ) ;
#34319=CARTESIAN_POINT ( 'NONE',  ( -15.38479227967843244, 26.80208864768298227, -5.945536811150080148 ) ) ;
#34320=CARTESIAN_POINT ( 'NONE',  ( -14.52190046171712368, -14.48203382165085529, -29.24551301647182910 ) ) ;
#34321=CARTESIAN_POINT ( 'NONE',  ( 8.048738417910207943, -21.01130598342334466, -20.86836972816746538 ) ) ;
#34322=CARTESIAN_POINT ( 'NONE',  ( 15.27515461409865338, 26.26107631968810452, -7.828561414818718589 ) ) ;
#34323=CARTESIAN_POINT ( 'NONE',  ( 16.98753680658756338, -11.47516704400511678, -30.00000000000002842 ) ) ;
#34327=CARTESIAN_POINT ( 'NONE',  ( -7.162297359993949897, 23.99211573040527057, -19.88175472533177057 ) ) ;
#34334=CARTESIAN_POINT ( 'NONE',  ( 25.19553447042465422, 0.4082270625723977142, -17.44156586897039674 ) ) ;
#34335=EDGE_CURVE ( 'NONE', #35064, #18367, #15804, .T. ) ;
#34342=CARTESIAN_POINT ( 'NONE',  ( -30.68377196017895514, 0.01256353404212825174, -6.888008929677917003 ) ) ;
#34345=CARTESIAN_POINT ( 'NONE',  ( 34.68926902183491023, -7.262543041722620885, -7.195073363372168629 ) ) ;
#34354=CARTESIAN_POINT ( 'NONE',  ( -16.15214517906706604, 12.62672657229183493, -30.00000000000001421 ) ) ;
#34359=CARTESIAN_POINT ( 'NONE',  ( 17.63833218921318036, 18.28698162993199006, -10.81605670618053772 ) ) ;
#34360=CARTESIAN_POINT ( 'NONE',  ( 9.666666246803703899, 33.51585335600255178, -9.377146499650510947 ) ) ;
#34362=CARTESIAN_POINT ( 'NONE',  ( 11.46616884858724461, -17.50945150416644580, -26.67433058872985896 ) ) ;
#34367=CARTESIAN_POINT ( 'NONE',  ( -11.01126394183691737, 17.29167595606526575, -29.34893377464801034 ) ) ;
#34369=CARTESIAN_POINT ( 'NONE',  ( 9.708222066279674323, -18.59847043248773346, -26.23215512439793073 ) ) ;
#34373=CARTESIAN_POINT ( 'NONE',  ( -11.31816643715098003, 20.85646170319403225, -20.38269801284040739 ) ) ;
#34374=CARTESIAN_POINT ( 'NONE',  ( -19.39179092967061280, -27.18907619913308338, -6.364284092723044850 ) ) ;
#34378=CARTESIAN_POINT ( 'NONE',  ( -21.76008645254054485, -6.076781144368697873, -23.17579509458892772 ) ) ;
#34379=CARTESIAN_POINT ( 'NONE',  ( -15.30203309327454697, -26.66931059147099248, -5.946105180059766404 ) ) ;
#34382=CARTESIAN_POINT ( 'NONE',  ( 30.10894569176270963, 0.2553795474248102271, -8.300237564504525878 ) ) ;
#34386=CARTESIAN_POINT ( 'NONE',  ( -20.81963202979064675, 0.7819132637707100209, -26.82682968236362342 ) ) ;
#34388=CARTESIAN_POINT ( 'NONE',  ( 20.49417979596975314, -0.6040919881699248206, -30.00000000000000000 ) ) ;
#34389=CARTESIAN_POINT ( 'NONE',  ( 18.63203339187605323, -8.577389641220674932, -30.00000000000002842 ) ) ;
#34392=CARTESIAN_POINT ( 'NONE',  ( -26.80025940592816980, 4.409708740836313368, -6.908737485017725888 ) ) ;
#34395=FACE_OUTER_BOUND ( 'NONE', #37676, .T. ) ;
#34403=CARTESIAN_POINT ( 'NONE',  ( -19.87474022753053760, 5.715682130751402745, -27.09873607923148242 ) ) ;
#34406=CARTESIAN_POINT ( 'NONE',  ( 22.86001989442993221, -26.57036944630193531, -7.206849629775319066 ) ) ;
#34408=CARTESIAN_POINT ( 'NONE',  ( 11.71074545945343459, 19.57405692998802849, -21.58253805519631285 ) ) ;
#34410=CARTESIAN_POINT ( 'NONE',  ( -12.32086914825891100, 16.51387112319463668, -28.14762509869785490 ) ) ;
#34413=CARTESIAN_POINT ( 'NONE',  ( 11.15651162539644758, 17.59102559401446797, -26.83334858599937434 ) ) ;
#34418=CARTESIAN_POINT ( 'NONE',  ( -15.19155625167785217, 26.86276375165831709, -7.348661200013363093 ) ) ;
#34420=CARTESIAN_POINT ( 'NONE',  ( -9.620588153019252076, -18.24824637790410264, -28.07461452513831901 ) ) ;
#34424=CARTESIAN_POINT ( 'NONE',  ( -19.49766833869776406, -10.22472788658466314, -24.22319853153801716 ) ) ;
#34425=CARTESIAN_POINT ( 'NONE',  ( -12.59681229544040981, -23.55840868995836246, -14.51872154415304372 ) ) ;
#34427=CARTESIAN_POINT ( 'NONE',  ( 16.14914138567496593, 22.68994970326915706, -9.283840620700846813 ) ) ;
#34428=ORIENTED_EDGE ( 'NONE', *, *, #10166, .F. ) ;
#34429=CARTESIAN_POINT ( 'NONE',  ( 19.66799848466891021, 5.910365882540998150, -28.83167407526441295 ) ) ;
#34435=CARTESIAN_POINT ( 'NONE',  ( -20.55088806256009804, 0.1873367080201817914, -28.68331257151926650 ) ) ;
#34436=CARTESIAN_POINT ( 'NONE',  ( 29.65834914286953250, -0.2741925911900300328, -10.62574247128935490 ) ) ;
#34441=CARTESIAN_POINT ( 'NONE',  ( 15.72991998290128990, -16.18894361744929000, -20.11584339644706887 ) ) ;
#34450=CARTESIAN_POINT ( 'NONE',  ( 3.737393764735764012, 36.42673618779068079, -9.293156675928717192 ) ) ;
#34457=CARTESIAN_POINT ( 'NONE',  ( 15.09524128205707072, 27.81033699783984403, -5.469350279337763965 ) ) ;
#34461=CARTESIAN_POINT ( 'NONE',  ( -15.52769020334683248, 13.63339048884298244, -27.12696093855038626 ) ) ;
#34465=CARTESIAN_POINT ( 'NONE',  ( 9.476873889470034840, -18.17797724348699973, -30.00000000000000000 ) ) ;
#34466=CARTESIAN_POINT ( 'NONE',  ( -15.52302998078869045, -20.83641103844984244, -18.06021460743331630 ) ) ;
#34467=CARTESIAN_POINT ( 'NONE',  ( 14.53385677051821290, 24.96618126256258918, -11.59944340942744034 ) ) ;
#34468=CARTESIAN_POINT ( 'NONE',  ( 15.40885724145108249, 26.80895719503613606, -5.000000000000000000 ) ) ;
#34471=CARTESIAN_POINT ( 'NONE',  ( -9.450798935534860945, -18.19154675410751310, -29.34931450394937613 ) ) ;
#34474=CARTESIAN_POINT ( 'NONE',  ( -31.25384702405562010, -21.56854527912942743, -7.121365677064556365 ) ) ;
#34475=CARTESIAN_POINT ( 'NONE',  ( -4.767036241218260528, -24.79638281802436595, -7.416925339961604635 ) ) ;
#34476=CARTESIAN_POINT ( 'NONE',  ( 12.70314503164341957, 20.08029170463875346, -19.55002564702039436 ) ) ;
#34479=CARTESIAN_POINT ( 'NONE',  ( 20.48907729733518224, 9.348693102924391596, -18.00296546062092773 ) ) ;
#34483=CARTESIAN_POINT ( 'NONE',  ( -20.42150163017176467, -2.418834129410442735, -28.59310508139819262 ) ) ;
#34489=CARTESIAN_POINT ( 'NONE',  ( -30.04950648410215308, 0.8457024189327566610, -5.474049384667112328 ) ) ;
#34490=CARTESIAN_POINT ( 'NONE',  ( 34.89591069308838911, -14.04604181989983935, -7.131079328635554937 ) ) ;
#34502=CARTESIAN_POINT ( 'NONE',  ( -3.913438197523118500, 34.93452689860740179, -11.08172396340525800 ) ) ;
#34508=CARTESIAN_POINT ( 'NONE',  ( 8.682226116870198851, 18.58302833326690262, -29.99999999999999645 ) ) ;
#34510=CARTESIAN_POINT ( 'NONE',  ( -19.49730985190667454, 11.63805976899694272, -16.98486636064236066 ) ) ;
#34512=CARTESIAN_POINT ( 'NONE',  ( 15.13256764714127200, -26.15839328056117807, -8.765583185149749212 ) ) ;
#34514=CARTESIAN_POINT ( 'NONE',  ( 12.89912295072652171, 21.70184657798560934, -17.43093282895208418 ) ) ;
#34515=CARTESIAN_POINT ( 'NONE',  ( -3.859759734048395785E-14, -22.74351282448223799, -21.56489709563626533 ) ) ;
#34518=CARTESIAN_POINT ( 'NONE',  ( -14.07208788724811477, -14.92005942896404669, -30.00000000000001421 ) ) ;
#34519=CARTESIAN_POINT ( 'NONE',  ( 9.624070444996608131, -20.74343144170484621, -20.71045537718826424 ) ) ;
#34520=CARTESIAN_POINT ( 'NONE',  ( 11.17775020265387553, 17.43158091459943293, -27.45587064061833615 ) ) ;
#34522=CARTESIAN_POINT ( 'NONE',  ( 16.98753680658756338, -11.47516704400511500, -29.21470985754709915 ) ) ;
#34525=ORIENTED_EDGE ( 'NONE', *, *, #9229, .F. ) ;
#34526=CARTESIAN_POINT ( 'NONE',  ( -7.450067287675317118, 31.53556863671898824, -12.97597155326280749 ) ) ;
#34530=CARTESIAN_POINT ( 'NONE',  ( 23.92490223308770680, 0.5234191831326777677, -19.50078697197409383 ) ) ;
#34535=CARTESIAN_POINT ( 'NONE',  ( -24.54231522334037408, 0.4673129468823389310, -18.45614678722852275 ) ) ;
#34538=CARTESIAN_POINT ( 'NONE',  ( 34.82172620998498047, -7.298527031968996326, -6.759101599951145012 ) ) ;
#34549=CARTESIAN_POINT ( 'NONE',  ( -19.64406637653126353, -6.006936621460132741, -30.00000000000001066 ) ) ;
#34553=CARTESIAN_POINT ( 'NONE',  ( 14.66009104707607769, 15.34232611559405335, -24.24183191570947216 ) ) ;
#34554=CARTESIAN_POINT ( 'NONE',  ( 9.894829114067803744, 34.42816785295285342, -7.613440901748822931 ) ) ;
#34557=CARTESIAN_POINT ( 'NONE',  ( 16.47043538305651467, -24.28946016894538573, -13.29763944434255230 ) ) ;
#34561=CARTESIAN_POINT ( 'NONE',  ( -12.40803774861176301, 20.46798912209962396, -19.49944249956930875 ) ) ;
#34564=CARTESIAN_POINT ( 'NONE',  ( 9.617438996837455178, -18.47535938133117739, -26.83658795940344177 ) ) ;
#34568=CARTESIAN_POINT ( 'NONE',  ( -10.16947320689176060, 18.25185904155808103, -26.74100241956728397 ) ) ;
#34571=CARTESIAN_POINT ( 'NONE',  ( -34.54759111898754753, -10.75241469091295166, -8.455612022062105382 ) ) ;
#34572=CARTESIAN_POINT ( 'NONE',  ( -15.32303194119059420, -26.70022385808693954, -5.000000000000000888 ) ) ;
#34576=CARTESIAN_POINT ( 'NONE',  ( 30.70345270623383627, 0.1631843812369964675, -5.000000000000000000 ) ) ;
#34577=CARTESIAN_POINT ( 'NONE',  ( 12.65336495406848627, 21.05333586960627557, -18.45227025400517462 ) ) ;
#34581=CARTESIAN_POINT ( 'NONE',  ( -22.73727917875568494, 0.5890566990126905322, -21.61446420491581577 ) ) ;
#34583=CARTESIAN_POINT ( 'NONE',  ( 32.55122689258003987, -2.282376514339032436, -6.834113689379055501 ) ) ;
#34598=CARTESIAN_POINT ( 'NONE',  ( -18.95922262551748361, 7.795319610833783663, -29.42417138239890306 ) ) ;
#34600=CARTESIAN_POINT ( 'NONE',  ( 24.04485151285368616, -26.41317262118404940, -6.755592305404338305 ) ) ;
#34601=CARTESIAN_POINT ( 'NONE',  ( -20.71631403513654845, -29.20819834831656436, -13.99845199583660182 ) ) ;
#34602=CARTESIAN_POINT ( 'NONE',  ( 12.54609464142508735, 21.21266715414756732, -18.42867748839541875 ) ) ;
#34605=CARTESIAN_POINT ( 'NONE',  ( -15.92491312827927885, 24.45805589641368982, -7.366686510344703898 ) ) ;
#34609=CARTESIAN_POINT ( 'NONE',  ( 14.04669866214605456, 23.89545579451645452, -13.51503478317237317 ) ) ;
#34613=CARTESIAN_POINT ( 'NONE',  ( -13.07870427894834719, 22.47409269205623161, -16.41433171529514112 ) ) ;
#34615=CARTESIAN_POINT ( 'NONE',  ( -15.70264670462719714, -26.79635097760029794, -5.473156990174284253 ) ) ;
#34616=CARTESIAN_POINT ( 'NONE',  ( 37.48557158514988430, -11.25000000000009237, 6.000000000000000000 ) ) ;
#34618=CARTESIAN_POINT ( 'NONE',  ( -32.79891082816697434, -15.91098148179321115, -9.730420382999001916 ) ) ;
#34619=CARTESIAN_POINT ( 'NONE',  ( -10.37379948539326513, -20.61367283351156487, -20.63258827435396014 ) ) ;
#34621=CARTESIAN_POINT ( 'NONE',  ( 13.66197743094250328, 18.08662167453329062, -20.78650099872353962 ) ) ;
#34623=CARTESIAN_POINT ( 'NONE',  ( 20.11222822097500540, 5.219997522146664792, -26.51068987014358669 ) ) ;
#34628=CARTESIAN_POINT ( 'NONE',  ( -12.11431921870781281, -16.53859995802357474, -30.00000000000001066 ) ) ;
#34630=CARTESIAN_POINT ( 'NONE',  ( -31.23446777708887367, -0.4277017081496246598, -5.940776528115775612 ) ) ;
#34631=CARTESIAN_POINT ( 'NONE',  ( 20.98375128680927659, 0.6676899881307120088, -26.21249548520855299 ) ) ;
#34632=AXIS2_PLACEMENT_3D ( 'NONE', #4157, #16562, #6597 ) ;
#34635=CARTESIAN_POINT ( 'NONE',  ( -19.54664213359414404, -11.28525909758381651, -19.69475445967427163 ) ) ;
#34644=CARTESIAN_POINT ( 'NONE',  ( 4.827317721685941976, 36.15751965146608171, -9.299952781395255386 ) ) ;
#34645=CARTESIAN_POINT ( 'NONE',  ( 0.000000000000000000, 22.50000000000000355, 10.00000000000000000 ) ) ;
#34652=CARTESIAN_POINT ( 'NONE',  ( 14.27905419341862192, 25.65267611664213732, -11.54866840426435992 ) ) ;
#34655=CARTESIAN_POINT ( 'NONE',  ( -18.21453708440813912, 18.61006694202274403, -6.921138814994913346 ) ) ;
#34659=CARTESIAN_POINT ( 'NONE',  ( 14.03725205635479512, -24.61054561307185296, -12.55068749160697017 ) ) ;
#34661=CARTESIAN_POINT ( 'NONE',  ( 11.69083868191524544, 18.90691405789837276, -22.73601728422654844 ) ) ;
#34663=CARTESIAN_POINT ( 'NONE',  ( 15.39245740739416668, 26.77485551171135114, -5.945824311378989258 ) ) ;
#34667=CARTESIAN_POINT ( 'NONE',  ( -10.17999638199554191, -19.18007577932459284, -23.85944600179882258 ) ) ;
#34670=CARTESIAN_POINT ( 'NONE',  ( -24.19767885117807538, -17.81929995649669252, -15.70298923897014198 ) ) ;
#34671=CARTESIAN_POINT ( 'NONE',  ( -2.147850760800578129, -22.42921841763291724, -18.01282657023325484 ) ) ;
#34672=CARTESIAN_POINT ( 'NONE',  ( 14.82034775369615964, 24.19848967327653000, -11.62209634349768628 ) ) ;
#34673=VERTEX_POINT ( 'NONE', #9682 ) ;
#34674=CARTESIAN_POINT ( 'NONE',  ( 22.00908396029312541, 11.01115965060166246, -8.406495840388641838 ) ) ;
#34678=CARTESIAN_POINT ( 'NONE',  ( -22.05094372219451415, -2.678342847933831816, -23.46479902602865053 ) ) ;
#34684=CARTESIAN_POINT ( 'NONE',  ( -20.39124144463984223, 2.214395427629727298, -29.37149834407417259 ) ) ;
#34685=CARTESIAN_POINT ( 'NONE',  ( 19.34370528778291742, -8.503836621211386060, -26.28178913655981930 ) ) ;
#34695=CARTESIAN_POINT ( 'NONE',  ( -0.6184052358777115677, 31.36018214284430528, -14.72953287677156098 ) ) ;
#34702=CARTESIAN_POINT ( 'NONE',  ( 10.70304607406188957, 23.48154281829076595, -18.10851452067850786 ) ) ;
#34704=AXIS2_PLACEMENT_3D ( 'NONE', #35504, #10717, #1576 ) ;
#34707=CARTESIAN_POINT ( 'NONE',  ( -18.03820307373585763, 9.850268257550711226, -28.29906855951537992 ) ) ;
#34710=CARTESIAN_POINT ( 'NONE',  ( 14.68418499867856752, -25.47351336547173162, -10.64941713223110220 ) ) ;
#34712=CARTESIAN_POINT ( 'NONE',  ( 15.39300221565557436, 26.86528302342467001, -5.000000000000000000 ) ) ;
#34713=CARTESIAN_POINT ( 'NONE',  ( 12.33616729053617966, -27.99489201236593416, -13.58461195433497437 ) ) ;
#34715=CARTESIAN_POINT ( 'NONE',  ( -16.01205366299697630, -16.95014973935591485, -22.09595210912920749 ) ) ;
#34716=CARTESIAN_POINT ( 'NONE',  ( 7.804347359704323139, -23.94321386332827117, -12.77188294322276718 ) ) ;
#34717=CARTESIAN_POINT ( 'NONE',  ( 11.11086231965098037, 17.28031181392691806, -28.71129638840202247 ) ) ;
#34718=CARTESIAN_POINT ( 'NONE',  ( 17.15651132827482073, -12.35653875792482381, -26.27594141802030236 ) ) ;
#34723=CARTESIAN_POINT ( 'NONE',  ( -8.445470182190037534, 36.08267608658951531, -5.870491325241125935 ) ) ;
#34729=CARTESIAN_POINT ( 'NONE',  ( 30.92038317698504457, -0.05869178374276581150, -5.474212382471533189 ) ) ;
#34734=CARTESIAN_POINT ( 'NONE',  ( -30.67041884990485912, 0.02637635525178676568, -6.888046746717600755 ) ) ;
#34735=FACE_OUTER_BOUND ( 'NONE', #8233, .T. ) ;
#34737=CARTESIAN_POINT ( 'NONE',  ( 24.34023952209733110, -5.793758624890436693, -19.88440862677620657 ) ) ;
#34750=CARTESIAN_POINT ( 'NONE',  ( -20.49397253890219162, -0.8422648960003168428, -30.00000000000000000 ) ) ;
#34753=CARTESIAN_POINT ( 'NONE',  ( 17.78493189837258370, 18.49202968733743546, -9.833181245109440027 ) ) ;
#34754=CARTESIAN_POINT ( 'NONE',  ( 5.827110988097120803, 22.69265212915571439, -22.03187520749546735 ) ) ;
#34756=CARTESIAN_POINT ( 'NONE',  ( 13.87211275201727112, -23.13071640756154679, -15.36481742136717266 ) ) ;
#34758=VECTOR ( 'NONE', #6321, 1000.000000000000000 ) ;
#34762=CARTESIAN_POINT ( 'NONE',  ( -12.94403022599198572, 21.62758146855915342, -17.44036610145013810 ) ) ;
#34765=CARTESIAN_POINT ( 'NONE',  ( 9.645968088698525733, -18.94145075774736853, -25.05036544634032936 ) ) ;
#34770=CARTESIAN_POINT ( 'NONE',  ( -9.094450958252869199, 19.08085575228837882, -26.00957991712340700 ) ) ;
#34771=CARTESIAN_POINT ( 'NONE',  ( -18.54826655067808261, -24.72227202651984967, -12.26027862526460233 ) ) ;
#34773=CARTESIAN_POINT ( 'NONE',  ( -34.72733857347371611, -7.593160847666269753, -7.191374443180106546 ) ) ;
#34776=CARTESIAN_POINT ( 'NONE',  ( 26.38915501620417459, 0.4550379995760640561, -15.46437747621563119 ) ) ;
#34781=CARTESIAN_POINT ( 'NONE',  ( -30.74697722743434980, -0.05262810487881691701, -6.887199586812257301 ) ) ;
#34783=CARTESIAN_POINT ( 'NONE',  ( 29.91755462158655732, -1.203610591981010947, -11.48839126716891990 ) ) ;
#34786=ORIENTED_EDGE ( 'NONE', *, *, #3206, .F. ) ;
#34797=CARTESIAN_POINT ( 'NONE',  ( -22.33456346850416452, 9.678077167578175377, -10.87421464888676148 ) ) ;
#34798=CARTESIAN_POINT ( 'NONE',  ( 16.51057184612255213, -20.52216718775187942, -17.97160528296034698 ) ) ;
#34800=CARTESIAN_POINT ( 'NONE',  ( 13.69960780509116915, 23.55256641442795384, -14.45987690255760505 ) ) ;
#34802=CARTESIAN_POINT ( 'NONE',  ( -11.71642904664754070, 16.82516707186347915, -29.99999999999999645 ) ) ;
#34805=CARTESIAN_POINT ( 'NONE',  ( 13.23742591511837396, 22.18590334729812241, -16.44840566425442319 ) ) ;
#34807=CARTESIAN_POINT ( 'NONE',  ( 33.16930538569719999, -19.62507065308114917, -4.999999999999998224 ) ) ;
#34810=CARTESIAN_POINT ( 'NONE',  ( -14.91983404371026012, 26.71086695692340740, -8.742635573326502652 ) ) ;
#34812=CARTESIAN_POINT ( 'NONE',  ( -16.73104734145491079, -26.99160526830743123, -5.933635577335993894 ) ) ;
#34817=CARTESIAN_POINT ( 'NONE',  ( -18.51592210607118716, -9.711178581313356872, -26.96926714808659042 ) ) ;
#34818=CARTESIAN_POINT ( 'NONE',  ( -13.21459172491393552, -24.49299878754191795, -12.58080149311899198 ) ) ;
#34820=CARTESIAN_POINT ( 'NONE',  ( 15.73060052599727499, 21.93190910970603369, -11.69130784369475151 ) ) ;
#34822=CARTESIAN_POINT ( 'NONE',  ( 28.06893040263355132, 2.889919344811102686, -6.900211441879279484 ) ) ;
#34823=EDGE_CURVE ( 'NONE', #27435, #38149, #14586, .T. ) ;
#34827=B_SPLINE_CURVE_WITH_KNOTS ( 'NONE', 3,
 ( #16494, #19738, #22774, #38424, #25422, #26025, #10597, #16288, #34577, #22979, #34984, #849, #6727, #32132, #19136, #13229 ),
 .UNSPECIFIED., .F., .F.,
 ( 4, 2, 2, 2, 2, 2, 2, 4 ),
 ( 0.000000000000000000, 0.1249999999374999671, 0.2499999998749999341, 0.4999999997500000903, 0.6249999996875000852, 0.7499999996249999690, 0.8749999995624999638, 0.9999999994999999586 ),
 .UNSPECIFIED. ) ;
#34829=CARTESIAN_POINT ( 'NONE',  ( -30.75436569807116172, -0.2981417031064238499, -7.815382463431599369 ) ) ;
#34830=CARTESIAN_POINT ( 'NONE',  ( 30.72321469840077057, -0.2642282358989092028, -7.816807012777728936 ) ) ;
#34836=CARTESIAN_POINT ( 'NONE',  ( 1.354211015180573125E-14, -26.63027081345975589, -13.39439507595156265 ) ) ;
#34844=CARTESIAN_POINT ( 'NONE',  ( 4.962866441237491877, 37.35289340691882387, -7.129294914047508591 ) ) ;
#34851=CARTESIAN_POINT ( 'NONE',  ( 23.06200705786680416, -18.88129698918507415, -15.73662040745943003 ) ) ;
#34856=CARTESIAN_POINT ( 'NONE',  ( 15.22299664760056537, 27.42699395385487904, -5.471105699861996463 ) ) ;
#34860=CARTESIAN_POINT ( 'NONE',  ( -14.82391975563179720, 16.62805930398341658, -20.93744056305393286 ) ) ;
#34863=CARTESIAN_POINT ( 'NONE',  ( 9.503358897673383154, -18.21462823815905452, -28.70764644545398880 ) ) ;
#34864=CARTESIAN_POINT ( 'NONE',  ( -19.48557158514988785, -11.24999999999987743, 10.00000000000000000 ) ) ;
#34865=CARTESIAN_POINT ( 'NONE',  ( 13.77319500370393435, 23.38836931657196772, -14.47646253997055332 ) ) ;
#34867=CARTESIAN_POINT ( 'NONE',  ( 10.98205083975412322, 17.31024513893945382, -30.00000000000000000 ) ) ;
#34870=CARTESIAN_POINT ( 'NONE',  ( -11.89641196761903963, -21.48543073582372998, -18.45346097597589718 ) ) ;
#34872=CARTESIAN_POINT ( 'NONE',  ( -22.05632830934130340, -15.21062374720687060, -18.62788710975480200 ) ) ;
#34873=CARTESIAN_POINT ( 'NONE',  ( -3.305456868217321986, -20.38071200921649861, -27.71575502845627170 ) ) ;
#34874=CARTESIAN_POINT ( 'NONE',  ( 11.81735879387240828, 18.14739419313247382, -23.90372284723114049 ) ) ;
#34876=CARTESIAN_POINT ( 'NONE',  ( 20.53826766272770143, 10.36318479709787077, -15.94093620634325070 ) ) ;
#34880=CARTESIAN_POINT ( 'NONE',  ( -33.49006840691916409, -4.412792004044882255, -7.689682260392150859 ) ) ;
#34888=CARTESIAN_POINT ( 'NONE',  ( 18.76590878806661067, -8.252041909800052366, -30.00000000000001421 ) ) ;
#34897=CARTESIAN_POINT ( 'NONE',  ( -1.178190889608008218, 23.73120932599768551, -21.84293309001832739 ) ) ;
#34906=CARTESIAN_POINT ( 'NONE',  ( 13.56803016854205168, 27.21220305392325400, -11.44257138522273287 ) ) ;
#34910=CARTESIAN_POINT ( 'NONE',  ( -19.69150485828470920, 15.64879689043717192, -5.481634527261435075 ) ) ;
#34913=CARTESIAN_POINT ( 'NONE',  ( 13.06130030674361819, -23.09502941311707147, -15.44577141088513272 ) ) ;
#34915=CARTESIAN_POINT ( 'NONE',  ( 11.14895963631104969, 17.78189646060649309, -26.22104407627368161 ) ) ;
#34917=CARTESIAN_POINT ( 'NONE',  ( -11.10756861982300947, 19.59949212537556562, -29.99999999999999645 ) ) ;
#34920=CARTESIAN_POINT ( 'NONE',  ( -16.57717488103276438, -16.52257091567909342, -22.04563894478580721 ) ) ;
#34921=CARTESIAN_POINT ( 'NONE',  ( 7.020580985973422727, -19.34222023316537786, -28.79039117229796219 ) ) ;
#34922=CARTESIAN_POINT ( 'NONE',  ( 15.47833181635298772, 26.56067009156167558, -5.474148242754607985 ) ) ;
#34923=CARTESIAN_POINT ( 'NONE',  ( 30.14705489269769956, -20.42482444568447519, -9.731448662954948148 ) ) ;
#34927=CARTESIAN_POINT ( 'NONE',  ( -5.778086282686619946, 24.63158676520072987, -19.78736581433748398 ) ) ;
#34931=CARTESIAN_POINT ( 'NONE',  ( 29.62952841301010665, 0.01294893774858196268, -10.17754520856805911 ) ) ;
#34935=VERTEX_POINT ( 'NONE', #1132 ) ;
#34936=CARTESIAN_POINT ( 'NONE',  ( -21.70210997138368469, 0.7650954235519592528, -23.85841552861994330 ) ) ;
#34937=CARTESIAN_POINT ( 'NONE',  ( -18.98517864320375281, -25.27528660476427547, -11.33194675972254650 ) ) ;
#34939=CARTESIAN_POINT ( 'NONE',  ( 25.27050923793063220, -6.013975129722774149, -18.85480297636462055 ) ) ;
#34942=ORIENTED_EDGE ( 'NONE', *, *, #36169, .T. ) ;
#34951=CARTESIAN_POINT ( 'NONE',  ( 7.782590637173006698, 18.96886919491949897, -30.00000000000000355 ) ) ;
#34958=CARTESIAN_POINT ( 'NONE',  ( 14.82374459613959949, 15.60418353992821849, -23.14626635614779460 ) ) ;
#34959=CARTESIAN_POINT ( 'NONE',  ( 10.43807493394656660, 32.55179874717006783, -9.848587368490356653 ) ) ;
#34961=CARTESIAN_POINT ( 'NONE',  ( 10.08241157172804670, -17.84938614438609505, -29.33613610785861781 ) ) ;
#34963=CARTESIAN_POINT ( 'NONE',  ( 0.000000000000000000, 22.50000000000000355, 10.00000000000000000 ) ) ;
#34964=AXIS2_PLACEMENT_3D ( 'NONE', #33993, #40074, #6150 ) ;
#34966=CARTESIAN_POINT ( 'NONE',  ( -10.99360060711668474, 17.30291464612033181, -29.99999999999999289 ) ) ;
#34967=VECTOR ( 'NONE', #12316, 1000.000000000000000 ) ;
#34969=CARTESIAN_POINT ( 'NONE',  ( 15.01751060382407310, -26.59764153146664256, -5.946174819114761867 ) ) ;
#34970=DIRECTION ( 'NONE',  ( -1.000000000000000000, 0.000000000000000000, 0.000000000000000000 ) ) ;
#34974=CARTESIAN_POINT ( 'NONE',  ( -9.456804962331334607, 19.97028186113128356, -23.55775169706302208 ) ) ;
#34979=CARTESIAN_POINT ( 'NONE',  ( -29.13564390960204165, -7.175030889379423016, -14.89359602007027483 ) ) ;
#34982=CARTESIAN_POINT ( 'NONE',  ( 20.60096619578946076, 1.002830394841245587, -28.08503524805096063 ) ) ;
#34984=CARTESIAN_POINT ( 'NONE',  ( 11.89393184406004877, 19.38028971260454369, -21.61737903493217416 ) ) ;
#34987=CARTESIAN_POINT ( 'NONE',  ( -22.22060807504403002, 0.6658104290297893746, -22.73532940052641038 ) ) ;
#34990=CARTESIAN_POINT ( 'NONE',  ( 31.53325577840491434, -2.954393997327824817, -10.45565772087099710 ) ) ;
#34991=CARTESIAN_POINT ( 'NONE',  ( 20.22742541439770392, -3.352094935268329134, -29.99999999999998579 ) ) ;
#34995=B_SPLINE_CURVE_WITH_KNOTS ( 'NONE', 3,
 ( #9054, #37080, #40118, #21438, #12297, #9250, #34039, #6195, #18601, #15546, #25084, #10799, #9655, #31574, #14039, #38827, #18990, #34628 ),
 .UNSPECIFIED., .F., .F.,
 ( 4, 2, 2, 2, 2, 2, 2, 2, 4 ),
 ( 5.000000244656254402E-10, 0.1250000003749999478, 0.2500000002499999097, 0.3750000001249998438, 0.4999999999999997780, 0.6249999998749997676, 0.7499999997499998683, 0.8749999996249998580, 0.9999999994999999586 ),
 .UNSPECIFIED. ) ;
#35006=CARTESIAN_POINT ( 'NONE',  ( -19.01510071548347369, 7.808900211911244504, -28.28496368704278652 ) ) ;
#35007=CARTESIAN_POINT ( 'NONE',  ( 13.09734119108189532, -16.42133399325533105, -26.53413149736031684 ) ) ;
#35010=CARTESIAN_POINT ( 'NONE',  ( 15.36061443993781062, 26.97785078317152596, -5.000000000000000888 ) ) ;
#35012=CARTESIAN_POINT ( 'NONE',  ( -14.35436364106707607, 23.18990942748935069, -13.54973528055356624 ) ) ;
#35015=CARTESIAN_POINT ( 'NONE',  ( 11.72828249552547142, 18.87102642502439664, -22.74204984032840926 ) ) ;
#35017=CARTESIAN_POINT ( 'NONE',  ( 18.24555790293216972, -9.366475481951450632, -30.00000000000002842 ) ) ;
#35020=CARTESIAN_POINT ( 'NONE',  ( -14.13481689797295715, 24.87588527889338863, -12.51643896934201372 ) ) ;
#35022=CARTESIAN_POINT ( 'NONE',  ( -16.57759486525810999, -26.77642802984841808, -7.325415354228808518 ) ) ;
#35026=CARTESIAN_POINT ( 'NONE',  ( -34.92155312733419237, -14.43004807528053135, -6.706874702558842216 ) ) ;
#35027=CARTESIAN_POINT ( 'NONE',  ( -14.23983225781402595, -26.43328798539083735, -4.999999999999999112 ) ) ;
#35029=CARTESIAN_POINT ( 'NONE',  ( 16.28234317699659783, 22.93167278076970561, -8.327167766279165662 ) ) ;
#35030=ORIENTED_EDGE ( 'NONE', *, *, #29476, .F. ) ;
#35031=CARTESIAN_POINT ( 'NONE',  ( 28.20661398414674537, 2.887420757311715658, -5.000000000000000000 ) ) ;
#35036=CARTESIAN_POINT ( 'NONE',  ( -20.49328727640310888, 0.5260942599782587603, -29.34226995137056448 ) ) ;
#35037=CARTESIAN_POINT ( 'NONE',  ( 31.56176620184661274, -0.7927402297087241534, -5.936147513203532178 ) ) ;
#35040=CARTESIAN_POINT ( 'NONE',  ( 13.28992586503610340, -18.25382200079949513, -29.99999999999999289 ) ) ;
#35050=CARTESIAN_POINT ( 'NONE',  ( 16.18705333424930970, -13.20565027319068996, -27.01267265381389393 ) ) ;
#35053=CARTESIAN_POINT ( 'NONE',  ( 10.63119325176788088, 18.14365359947311873, -26.16532366619414418 ) ) ;
#35056=CARTESIAN_POINT ( 'NONE',  ( -14.29743425985715355, 15.73966817516812888, -24.20757674709752649 ) ) ;
#35058=CARTESIAN_POINT ( 'NONE',  ( 14.58890700129304463, -25.45407539014443898, -10.65398993192215293 ) ) ;
#35061=CARTESIAN_POINT ( 'NONE',  ( 15.23445058273096464, 26.39864931307285900, -7.828033204951921675 ) ) ;
#35063=CARTESIAN_POINT ( 'NONE',  ( 11.06818295498493576, 17.50574775501806357, -27.44742483198325189 ) ) ;
#35064=VERTEX_POINT ( 'NONE', #19826 ) ;
#35065=CARTESIAN_POINT ( 'NONE',  ( -11.42130609047572065, 18.49161963548644394, -23.84395533656347865 ) ) ;
#35067=CARTESIAN_POINT ( 'NONE',  ( -9.469408548107701051, -18.18187935292228019, -30.00000000000000000 ) ) ;
#35070=CARTESIAN_POINT ( 'NONE',  ( -22.98950691836191496, -13.88151727732919838, -18.61066130745788882 ) ) ;
#35071=CARTESIAN_POINT ( 'NONE',  ( -3.533336070225259196, -21.04848782586652689, -23.28608928280259960 ) ) ;
#35072=CARTESIAN_POINT ( 'NONE',  ( 14.58699662364080929, 23.73430093865497170, -12.57910105661215638 ) ) ;
#35074=CARTESIAN_POINT ( 'NONE',  ( 21.05083558980209801, 7.683405658820698036, -18.99948416535620765 ) ) ;
#35077=CARTESIAN_POINT ( 'NONE',  ( -15.18941732005890266, -26.66619070650552459, -5.000000000000001776 ) ) ;
#35080=CARTESIAN_POINT ( 'NONE',  ( -32.65566155904921430, -4.264910902414662530, -9.490589700126765393 ) ) ;
#35086=CARTESIAN_POINT ( 'NONE',  ( 34.30740497575424541, -16.27724728724163228, -7.121324501852425826 ) ) ;
#35091=CARTESIAN_POINT ( 'NONE',  ( -30.90412082983564446, -0.04211290444597337590, -5.000000000000000888 ) ) ;
#35095=CARTESIAN_POINT ( 'NONE',  ( -0.7518768309112285886, 38.37606218726813267, -6.275896992768287497 ) ) ;
#35103=CARTESIAN_POINT ( 'NONE',  ( 11.49081439112069702, 22.60309983489513286, -18.22883438010077484 ) ) ;
#35106=CARTESIAN_POINT ( 'NONE',  ( -18.17263180773770159, 11.81850911556306372, -21.17646943544158944 ) ) ;
#35109=CARTESIAN_POINT ( 'NONE',  ( 11.94195138395211941, -21.48248341615735768, -18.44782710392617631 ) ) ;
#35113=CARTESIAN_POINT ( 'NONE',  ( 12.91186190338204298, 21.68060954549180863, -17.43383681951817721 ) ) ;
#35114=CARTESIAN_POINT ( 'NONE',  ( -19.69645987729884595, 11.37175641224114919, -21.56489709563623691 ) ) ;
#35116=CARTESIAN_POINT ( 'NONE',  ( -15.10985780742689499, -15.06563729506261851, -25.73346922605977127 ) ) ;
#35117=CARTESIAN_POINT ( 'NONE',  ( 8.497644768481743327, -25.32189558139016228, -5.477296350422366622 ) ) ;
#35118=CARTESIAN_POINT ( 'NONE',  ( 13.84574913428668275, 23.23330865849091253, -14.48585008083296266 ) ) ;
#35119=CARTESIAN_POINT ( 'NONE',  ( 19.90145156205069554, 13.46129076908396627, -11.87680844943539249 ) ) ;
#35123=CARTESIAN_POINT ( 'NONE',  ( -5.983447258044394701, 19.98291656352506251, -27.11177212607830000 ) ) ;
#35128=CARTESIAN_POINT ( 'NONE',  ( 22.73483984765169197, 0.5967685963425408691, -21.61569754599228688 ) ) ;
#35131=EDGE_CURVE ( 'NONE', #29462, #33574, #13719, .T. ) ;
#35135=CARTESIAN_POINT ( 'NONE',  ( -29.66313021947697592, 0.1976963186581543463, -9.712199395440693550 ) ) ;
#35138=CARTESIAN_POINT ( 'NONE',  ( 31.89272422543808361, -8.553727179860587171, -12.07502465680937576 ) ) ;
#35147=CARTESIAN_POINT ( 'NONE',  ( 0.4281292814599761409, 20.49824620653738450, -30.00000000000000000 ) ) ;
#35151=CARTESIAN_POINT ( 'NONE',  ( 17.69882028648708783, 20.03130879389887298, -5.955324216395004200 ) ) ;
#35152=CARTESIAN_POINT ( 'NONE',  ( 8.855091917839381210, 30.59299078850003539, -13.02531624040802072 ) ) ;
#35155=DIRECTION ( 'NONE',  ( 0.000000000000000000, 0.000000000000000000, 1.000000000000000000 ) ) ;
#35157=CARTESIAN_POINT ( 'NONE',  ( 10.14866111327665266, -18.21960830426016997, -26.79090690569056221 ) ) ;
#35161=CARTESIAN_POINT ( 'NONE',  ( -14.29967717032973518, 24.44936570868513215, -12.55117429398542939 ) ) ;
#35163=CARTESIAN_POINT ( 'NONE',  ( 14.06663363425422908, -25.35442907823021130, -10.66521829186682702 ) ) ;
#35168=CARTESIAN_POINT ( 'NONE',  ( -10.84898765319574743, 23.30394029384613575, -18.13347752456717998 ) ) ;
#35172=CARTESIAN_POINT ( 'NONE',  ( -32.40829156996449711, -7.016000414201827518, -11.20844734717147162 ) ) ;
#35175=CARTESIAN_POINT ( 'NONE',  ( 29.86380350792722282, 0.1690758829598159041, -9.240701576314629406 ) ) ;
#35179=CARTESIAN_POINT ( 'NONE',  ( -30.91582600597228137, -0.05403808547916690019, -5.474125485033605187 ) ) ;
#35183=CARTESIAN_POINT ( 'NONE',  ( 32.52266725778360268, -3.089069589389634274, -8.625450327480431056 ) ) ;
#35196=EDGE_CURVE ( 'NONE', #25273, #15130, #1009, .T. ) ;
#35198=CARTESIAN_POINT ( 'NONE',  ( -19.10455879864122153, 7.830559145427559820, -27.15426290237969198 ) ) ;
#35199=CARTESIAN_POINT ( 'NONE',  ( 13.39371427707866147, -15.78149709652679533, -27.86034563683584508 ) ) ;
#35201=CARTESIAN_POINT ( 'NONE',  ( 14.78333195896292729, 25.78429753009990577, -10.16969888846196568 ) ) ;
#35203=CARTESIAN_POINT ( 'NONE',  ( -12.04424134404128921, 16.72615764091300861, -28.13376640329193634 ) ) ;
#35207=CARTESIAN_POINT ( 'NONE',  ( 15.36863164365442103, 26.51124612085094867, -6.888122883055683765 ) ) ;
#35209=CARTESIAN_POINT ( 'NONE',  ( 18.76822264364483317, -10.35557248195002877, -25.57773590016846654 ) ) ;
#35211=EDGE_LOOP ( 'NONE', ( #14678, #25160 ) ) ;
#35212=CARTESIAN_POINT ( 'NONE',  ( -15.19876735762676034, 27.08650375569634861, -6.877893297480420109 ) ) ;
#35214=CARTESIAN_POINT ( 'NONE',  ( -10.41468997611843506, -18.62962352831552693, -24.96183479470249367 ) ) ;
#35218=CARTESIAN_POINT ( 'NONE',  ( -35.38382356931356298, -13.39769055746643289, -5.438178884671905244 ) ) ;
#35219=CARTESIAN_POINT ( 'NONE',  ( -14.09564871292362476, -26.21398149618797291, -7.362640844368039339 ) ) ;
#35220=FACE_OUTER_BOUND ( 'NONE', #15791, .T. ) ;
#35221=CARTESIAN_POINT ( 'NONE',  ( 13.32665242662786120, 15.89484158179648610, -27.00953544631929759 ) ) ;
#35223=CARTESIAN_POINT ( 'NONE',  ( 28.20661398414674537, 2.887420757311715658, -5.474884631757898745 ) ) ;
#35229=CARTESIAN_POINT ( 'NONE',  ( -30.99742014632522569, -0.1379718400911541798, -5.473566688364370769 ) ) ;
#35231=CARTESIAN_POINT ( 'NONE',  ( 31.60127994866165224, -0.7964638025070726046, -5.000000000000000000 ) ) ;
#35235=CARTESIAN_POINT ( 'NONE',  ( -19.69645987729884595, 11.37175641224115097, -29.99999999999998934 ) ) ;
#35251=CARTESIAN_POINT ( 'NONE',  ( 16.57028389081698094, -14.37381587238541059, -24.32133266205364563 ) ) ;
#35254=CARTESIAN_POINT ( 'NONE',  ( 15.20648748154197882, 27.39160813737696998, -5.939486291738587553 ) ) ;
#35256=B_SPLINE_CURVE_WITH_KNOTS ( 'NONE', 3,
 ( #6753, #34601, #25849, #1279 ),
 .UNSPECIFIED., .F., .F.,
 ( 4, 4 ),
 ( 0.000000000000000000, 1.000000000000000000 ),
 .UNSPECIFIED. ) ;
#35257=ORIENTED_EDGE ( 'NONE', *, *, #21732, .F. ) ;
#35259=CARTESIAN_POINT ( 'NONE',  ( -17.69219503082499756, 19.52419099561771176, -7.880095719941950350 ) ) ;
#35261=CARTESIAN_POINT ( 'NONE',  ( 14.32771630080133463, -25.06525504208602939, -11.59986630204942060 ) ) ;
#35263=CARTESIAN_POINT ( 'NONE',  ( 15.18140632243098054, 26.25845010830521531, -8.297908434051732840 ) ) ;
#35265=CARTESIAN_POINT ( 'NONE',  ( 14.28858787313288481, 24.47746469342002129, -12.55008231428947596 ) ) ;
#35267=CARTESIAN_POINT ( 'NONE',  ( -10.94041201910780359, 17.33660477453622306, -29.99999999999999645 ) ) ;
#35269=CARTESIAN_POINT ( 'NONE',  ( -15.47550425816466557, -26.73936689671932143, -5.000000000000000888 ) ) ;
#35271=CARTESIAN_POINT ( 'NONE',  ( -32.64518230009728939, -19.71632926622226734, -7.116952983000433441 ) ) ;
#35273=CARTESIAN_POINT ( 'NONE',  ( -2.394825184670892781, -23.73107514896808112, -12.88530523879403944 ) ) ;
#35274=CARTESIAN_POINT ( 'NONE',  ( 11.41005643133681957, 17.03110932016596735, -29.35731938081785941 ) ) ;
#35276=CARTESIAN_POINT ( 'NONE',  ( 19.21215415183591446, 7.317176409479575483, -28.27861274171054973 ) ) ;
#35277=CARTESIAN_POINT ( 'NONE',  ( 34.38704122072325475, -17.20178129237611842, -4.999999999999999112 ) ) ;
#35281=CARTESIAN_POINT ( 'NONE',  ( -20.43418187165424982, -1.772479648697218302, -29.30004495981471990 ) ) ;
#35287=EDGE_CURVE ( 'NONE', #20607, #39797, #14327, .T. ) ;
#35288=CARTESIAN_POINT ( 'NONE',  ( 24.72333287932298163, -9.962440173953478251, -18.66584102224920372 ) ) ;
#35297=CARTESIAN_POINT ( 'NONE',  ( -1.339087178513852283, 26.79985410012201541, -18.61668850162147848 ) ) ;
#35304=CARTESIAN_POINT ( 'NONE',  ( 9.656570333113133842, 18.37762487846717363, -27.33940497250931045 ) ) ;
#35307=CARTESIAN_POINT ( 'NONE',  ( -18.55075427606121252, 13.25029436287058715, -16.96479077551187586 ) ) ;
#35311=CARTESIAN_POINT ( 'NONE',  ( 9.569772169525011307, -18.12929409070867948, -29.34686813031393271 ) ) ;
#35313=CARTESIAN_POINT ( 'NONE',  ( 15.40208502184672135, 26.83309954512951023, -5.473965072825944134 ) ) ;
#35314=CARTESIAN_POINT ( 'NONE',  ( -21.88499642459564853, -5.528038495964381127, -30.00000000000000355 ) ) ;
#35317=CARTESIAN_POINT ( 'NONE',  ( -22.16102929819185974, -19.64143327435995801, -15.76658576923206034 ) ) ;
#35318=CARTESIAN_POINT ( 'NONE',  ( 7.953009581834296071, -24.24005142096364551, -11.78114088531529191 ) ) ;
#35319=CARTESIAN_POINT ( 'NONE',  ( 11.61490188824428493, 18.32440375615002282, -23.87370887680063447 ) ) ;
#35320=CARTESIAN_POINT ( 'NONE',  ( 16.68830378044837914, 11.92867436094057787, -29.99999999999999645 ) ) ;
#35321=DIRECTION ( 'NONE',  ( 1.000000000000000000, 0.000000000000000000, 0.000000000000000000 ) ) ;
#35324=CARTESIAN_POINT ( 'NONE',  ( -8.157141749000260234, 34.61756633539883410, -9.342187312551713418 ) ) ;
#35325=ORIENTED_EDGE ( 'NONE', *, *, #33101, .F. ) ;
#35327=CARTESIAN_POINT ( 'NONE',  ( -9.469853072659795146, -18.32362292512856428, -28.08296521917836941 ) ) ;
#35330=CARTESIAN_POINT ( 'NONE',  ( 30.81126407598692651, -0.05061877264937817561, -6.416964798920022695 ) ) ;
#35336=CARTESIAN_POINT ( 'NONE',  ( -22.20966955782450469, 0.7103411302137916383, -22.74070771460645091 ) ) ;
#35338=CARTESIAN_POINT ( 'NONE',  ( 19.94806447466153543, -4.723319992639698484, -29.25382421619654849 ) ) ;
#35352=( LENGTH_UNIT ( ) NAMED_UNIT ( * ) SI_UNIT ( .MILLI., .METRE. ) );
#35356=CARTESIAN_POINT ( 'NONE',  ( 15.87504137958280559, 15.79823347536147082, -19.97344786039081654 ) ) ;
#35357=CARTESIAN_POINT ( 'NONE',  ( 7.777352336794518983, 26.89720915371588816, -16.82449721399039078 ) ) ;
#35363=CARTESIAN_POINT ( 'NONE',  ( 13.26834981302413752, -22.56586285155463756, -16.37744211164412533 ) ) ;
#35367=CARTESIAN_POINT ( 'NONE',  ( -13.49987786938234535, 22.79920604360487602, -15.45166244955937707 ) ) ;
#35369=CARTESIAN_POINT ( 'NONE',  ( 14.66427835382668299, -26.25532329094042439, -7.831039160053395953 ) ) ;
#35373=CARTESIAN_POINT ( 'NONE',  ( -11.48887937525355341, 24.79999023685312309, -16.14676052428935904 ) ) ;
#35375=CARTESIAN_POINT ( 'NONE',  ( -16.57032934033265192, -22.18377020236782826, -16.08031648850850104 ) ) ;
#35378=CARTESIAN_POINT ( 'NONE',  ( -35.20073123246135083, -8.756190693406901815, -6.311296342382265223 ) ) ;
#35382=CARTESIAN_POINT ( 'NONE',  ( 22.68044555609654367, 0.7780309201116830664, -21.63808993525804780 ) ) ;
#35386=CARTESIAN_POINT ( 'NONE',  ( -22.22324547119116289, 0.6552216296766762982, -22.73395167228940750 ) ) ;
#35390=CARTESIAN_POINT ( 'NONE',  ( 20.47947323059178260, -0.9304062671392134831, -29.31544170430820628 ) ) ;
#35405=CARTESIAN_POINT ( 'NONE',  ( -22.90242673301339593, 8.786414512089246287, -10.86241974061178972 ) ) ;
#35407=CARTESIAN_POINT ( 'NONE',  ( 20.28942584164974505, -25.11661602538714888, -11.27543687046667387 ) ) ;
#35410=CARTESIAN_POINT ( 'NONE',  ( 14.96161369655125206, 26.15114394812015064, -9.229261913996447575 ) ) ;
#35412=CARTESIAN_POINT ( 'NONE',  ( -15.03288268948483264, 23.64078904719026042, -11.63896337504832879 ) ) ;
#35415=CARTESIAN_POINT ( 'NONE',  ( 14.56710521870112807, 24.87586913598118343, -11.60179260043244653 ) ) ;
#35417=CARTESIAN_POINT ( 'NONE',  ( 24.85582250148247496, -12.74015949003176651, -17.59997480698870476 ) ) ;
#35420=CARTESIAN_POINT ( 'NONE',  ( -10.74659509297316440, 17.51247683012617884, -28.69615268264896102 ) ) ;
#35422=CARTESIAN_POINT ( 'NONE',  ( -16.49457207817568261, -26.65912990296860130, -7.789058334551107521 ) ) ;
#35423=DIRECTION ( 'NONE',  ( 0.000000000000000000, 0.000000000000000000, 1.000000000000000000 ) ) ;
#35425=CARTESIAN_POINT ( 'NONE',  ( -24.63622891667736781, -10.18470011515834095, -18.66157544239288057 ) ) ;
#35426=CARTESIAN_POINT ( 'NONE',  ( -9.357072968089592990, -18.59482942431551677, -26.85790916864404565 ) ) ;
#35428=CARTESIAN_POINT ( 'NONE',  ( 14.67864225457747906, 16.82336705159722001, -20.92344909559215793 ) ) ;
#35430=CARTESIAN_POINT ( 'NONE',  ( 25.64058186160713859, 3.762799545439524440, -12.71090497642184580 ) ) ;
#35434=EDGE_LOOP ( 'NONE', ( #25812, #23191 ) ) ;
#35435=CARTESIAN_POINT ( 'NONE',  ( -20.99434144220187548, 0.5542567078580580286, -26.20245057682946310 ) ) ;
#35437=CARTESIAN_POINT ( 'NONE',  ( 30.84859707095975878, -0.5449750927740264483, -8.270921991002078144 ) ) ;
#35441=AXIS2_PLACEMENT_3D ( 'NONE', #28607, #583, #7262 ) ;
#35444=CARTESIAN_POINT ( 'NONE',  ( -28.84245173844059806, 0.9132675324983203780, -10.20106989243743278 ) ) ;
#35445=CARTESIAN_POINT ( 'NONE',  ( -6.023418944065151770, 39.81932404830322270, -14.45070082761206365 ) ) ;
#35455=CARTESIAN_POINT ( 'NONE',  ( 15.94967524335434739, -13.83360700755901185, -26.33159008689450431 ) ) ;
#35461=CARTESIAN_POINT ( 'NONE',  ( 10.41696638283783471, 17.65700839937217381, -29.33613504912931091 ) ) ;
#35464=CARTESIAN_POINT ( 'NONE',  ( -17.64770094672744349, 19.45792562635240230, -8.363180893698942242 ) ) ;
#35467=CARTESIAN_POINT ( 'NONE',  ( 13.32179451523274238, -23.61806545529600143, -14.47902645169415337 ) ) ;
#35469=CARTESIAN_POINT ( 'NONE',  ( 11.69932325419884300, 18.89880935514919713, -22.73734831153147695 ) ) ;
#35471=CARTESIAN_POINT ( 'NONE',  ( 15.36544744475249580, 26.69572735888668902, -6.416978652968691854 ) ) ;
#35473=CARTESIAN_POINT ( 'NONE',  ( -14.81640337485448100, 25.68318687829989599, -10.17575449534364829 ) ) ;
#35475=CARTESIAN_POINT ( 'NONE',  ( -13.67385565238511269, -24.11288955641917298, -13.51489229801976322 ) ) ;
#35477=CARTESIAN_POINT ( 'NONE',  ( -28.90832190807780222, -18.69259600629643714, -11.97739893689305646 ) ) ;
#35478=CARTESIAN_POINT ( 'NONE',  ( -5.491606936905080616, -21.66488701077363643, -19.98327345564413449 ) ) ;
#35479=CARTESIAN_POINT ( 'NONE',  ( 14.03912507337044779, 21.76248058076597403, -15.52699132478714894 ) ) ;
#35481=CARTESIAN_POINT ( 'NONE',  ( 23.83304178564468501, 8.268703381674290753, -7.903184250208921569 ) ) ;
#35483=CARTESIAN_POINT ( 'NONE',  ( 15.48853125999101898, -26.74269726803731828, -5.000000000000000000 ) ) ;
#35486=CARTESIAN_POINT ( 'NONE',  ( -32.11025114950868442, -1.657766350062749527, -6.846984724189184135 ) ) ;
#35492=CARTESIAN_POINT ( 'NONE',  ( 75.15099915297797395, 43.38844959084117647, 3.000000000000000000 ) ) ;
#35494=CARTESIAN_POINT ( 'NONE',  ( 28.51905879638759700, -12.47949435409169539, -14.75475664525949071 ) ) ;
#35498=CARTESIAN_POINT ( 'NONE',  ( -32.33143948541789570, 1.358872982501806215, 0.000000000000000000 ) ) ;
#35503=CARTESIAN_POINT ( 'NONE',  ( -0.5479328185110891036, 27.95115490892091259, -17.59429925479824064 ) ) ;
#35504=CARTESIAN_POINT ( 'NONE',  ( 0.000000000000000000, 0.000000000000000000, -30.00000000000000000 ) ) ;
#35508=CARTESIAN_POINT ( 'NONE',  ( -20.57924982997939622, -27.21273881503329051, -4.999999999999998224 ) ) ;
#35509=CARTESIAN_POINT ( 'NONE',  ( 14.05079942517586389, 29.36071225880166580, -7.738770433462001108 ) ) ;
#35512=CARTESIAN_POINT ( 'NONE',  ( -17.27691955920570877, 11.15657196891051228, -28.29868769472810541 ) ) ;
#35515=CARTESIAN_POINT ( 'NONE',  ( 15.41906236961596655, -26.60135734087577219, -6.887199331419184389 ) ) ;
#35517=CARTESIAN_POINT ( 'NONE',  ( 11.03763599804776341, 17.52625919505898011, -27.44504327041069303 ) ) ;
#35518=CARTESIAN_POINT ( 'NONE',  ( -33.62187204924172335, 0.04418559750806001774, -13.79123840944734347 ) ) ;
#35522=CARTESIAN_POINT ( 'NONE',  ( -26.61324971144608043, -23.59943729456863082, -9.772242488793104087 ) ) ;
#35523=CARTESIAN_POINT ( 'NONE',  ( 7.642913368978748956, -23.62237106133328624, -13.77340500620915620 ) ) ;
#35524=CARTESIAN_POINT ( 'NONE',  ( 13.35043658488273266, 21.98571059302396336, -16.46575276999205073 ) ) ;
#35525=CARTESIAN_POINT ( 'NONE',  ( 20.47654757076874787, 13.90376119549317124, -7.426114723384639404 ) ) ;
#35528=CARTESIAN_POINT ( 'NONE',  ( -7.286326729150405690, 35.71687252700443338, -8.445018646286913011 ) ) ;
#35531=CARTESIAN_POINT ( 'NONE',  ( -12.52581896409591877, -22.55617444508696678, -16.45362975895816504 ) ) ;
#35538=CARTESIAN_POINT ( 'NONE',  ( -30.74131631141073129, 0.1242922002067064352, -5.474147495693744148 ) ) ;
#35540=CARTESIAN_POINT ( 'NONE',  ( 22.59748200846286181, -6.094062071576993311, -22.04567670539332624 ) ) ;
#35555=CARTESIAN_POINT ( 'NONE',  ( 18.53648777117533442, 17.88871277907829338, -6.924686450352337985 ) ) ;
#35556=AXIS2_PLACEMENT_3D ( 'NONE', #2258, #36385, #39224 ) ;
#35557=CARTESIAN_POINT ( 'NONE',  ( 9.323248225502032582, 32.23778593834843065, -11.17991894423324339 ) ) ;
#35562=CARTESIAN_POINT ( 'NONE',  ( 14.04058618686241466, -23.68300519570117402, -14.41379008992138822 ) ) ;
#35566=CARTESIAN_POINT ( 'NONE',  ( -15.10048454435680831, 26.14110364457479818, -8.767509008662626613 ) ) ;
#35568=CARTESIAN_POINT ( 'NONE',  ( 14.81091239784893077, -26.28932095263721536, -7.830188071801472915 ) ) ;
#35574=CARTESIAN_POINT ( 'NONE',  ( -10.30011504994442717, 23.87368139273885248, -18.05724923619832012 ) ) ;
#35580=CARTESIAN_POINT ( 'NONE',  ( -32.61466699540454073, -8.035061020377614938, -11.17799411198647164 ) ) ;
#35583=CARTESIAN_POINT ( 'NONE',  ( 30.47622998064611721, 0.1276006758484945214, -7.358534401045794482 ) ) ;
#35590=CARTESIAN_POINT ( 'NONE',  ( -22.73404044138284164, 0.5996816946850819230, -21.61592112696820678 ) ) ;
#35592=CARTESIAN_POINT ( 'NONE',  ( 30.45180831424324808, -2.034437368685610981, -11.43179728121123162 ) ) ;
#35593=CARTESIAN_POINT ( 'NONE',  ( 20.50220473200229065, -0.6271520275686577328, -30.00000000000000711 ) ) ;
#35606=CARTESIAN_POINT ( 'NONE',  ( 6.092423932518094887, 37.33975570695338320, -5.438183848281402888 ) ) ;
#35609=CARTESIAN_POINT ( 'NONE',  ( 20.81479864165018512, -27.12526061484643236, -6.349197363260469018 ) ) ;
#35616=CARTESIAN_POINT ( 'NONE',  ( 14.80287293261903159, 25.72487161761031516, -10.17325132652339903 ) ) ;
#35618=CARTESIAN_POINT ( 'NONE',  ( -11.56430756512898661, 17.30006398449676297, -26.87031197432354901 ) ) ;
#35621=CARTESIAN_POINT ( 'NONE',  ( 11.03950910960345766, 17.27365618835783678, -30.00000000000000000 ) ) ;
#35623=CARTESIAN_POINT ( 'NONE',  ( 21.96604632341627195, -11.26784406932779348, -20.69622655604641537 ) ) ;
#35625=CARTESIAN_POINT ( 'NONE',  ( -15.23746052738172096, 27.38211562678985445, -5.471314660788269890 ) ) ;
#35627=CARTESIAN_POINT ( 'NONE',  ( -15.51450792689023750, -25.25784468116843229, -11.51896233938664693 ) ) ;
#35629=VERTEX_POINT ( 'NONE', #21615 ) ;
#35630=CARTESIAN_POINT ( 'NONE',  ( -34.21394365919860547, -14.11642697757303644, -8.422019832718921961 ) ) ;
#35631=CARTESIAN_POINT ( 'NONE',  ( -14.49814074169044709, -25.88491989834313145, -9.244276984472083569 ) ) ;
#35633=CARTESIAN_POINT ( 'NONE',  ( 17.24384880539558651, 21.04619446147080097, -6.430924243040796462 ) ) ;
#35635=CARTESIAN_POINT ( 'NONE',  ( 20.31991420201310206, 4.509322195999590832, -26.47951906542851930 ) ) ;
#35639=CARTESIAN_POINT ( 'NONE',  ( -27.27908345015220348, 0.04356745379364866666, -14.45463337275631233 ) ) ;
#35641=CARTESIAN_POINT ( 'NONE',  ( 24.07089776856416563, 0.1762921601959324680, -19.45410240058878770 ) ) ;
#35646=CARTESIAN_POINT ( 'NONE',  ( -20.88993331574549117, 1.492557873551023873, -26.28200927340007809 ) ) ;
#35649=CARTESIAN_POINT ( 'NONE',  ( -6.155076441694329326, 21.71698211341365692, -29.99999999999997868 ) ) ;
#35656=CARTESIAN_POINT ( 'NONE',  ( -26.20904522235016287, 5.310845850833655568, -5.477248126412333384 ) ) ;
#35659=CARTESIAN_POINT ( 'NONE',  ( 26.06425415636434906, -22.71578164446442827, -11.11508149911450793 ) ) ;
#35663=CARTESIAN_POINT ( 'NONE',  ( 10.77401535176683822, 17.85200931278258807, -26.79744273874945293 ) ) ;
#35667=CARTESIAN_POINT ( 'NONE',  ( -14.81419240842891050, 15.18325971397014307, -24.25831821709929415 ) ) ;
#35669=EDGE_CURVE ( 'NONE', #14281, #7759, #38646, .T. ) ;
#35670=CARTESIAN_POINT ( 'NONE',  ( 15.37571132048090838, -26.71368809714059722, -5.474175248281667017 ) ) ;
#35672=CARTESIAN_POINT ( 'NONE',  ( 14.74942196309478604, 25.36140116702692637, -10.65398990804295032 ) ) ;
#35673=ORIENTED_EDGE ( 'NONE', *, *, #14841, .T. ) ;
#35674=CARTESIAN_POINT ( 'NONE',  ( 11.67905974016245629, 18.91828259921463129, -22.73395179757990547 ) ) ;
#35675=ORIENTED_EDGE ( 'NONE', *, *, #851, .T. ) ;
#35676=CARTESIAN_POINT ( 'NONE',  ( -11.13871245836219259, 17.78928257176252359, -26.21993262638637034 ) ) ;
#35678=CARTESIAN_POINT ( 'NONE',  ( -15.33464666325443559, -26.58010993391619792, -6.888001209383307177 ) ) ;
#35680=CARTESIAN_POINT ( 'NONE',  ( -30.32740607997149240, -18.32269088211211994, -11.06668654378994887 ) ) ;
#35681=CARTESIAN_POINT ( 'NONE',  ( -4.810070356376328071, -20.19244794699170953, -26.53957745834831528 ) ) ;
#35682=CARTESIAN_POINT ( 'NONE',  ( 15.91914112585197216, 24.98921244238988493, -5.946992071948343117 ) ) ;
#35684=CARTESIAN_POINT ( 'NONE',  ( 21.66250921451431921, 7.810554196117029058, -16.92292203280336693 ) ) ;
#35689=CARTESIAN_POINT ( 'NONE',  ( -23.96107556257267746, -1.546995113576812964, -20.27043652965265608 ) ) ;
#35696=LINE ( 'NONE', #7850, #10605 ) ;
#35697=CARTESIAN_POINT ( 'NONE',  ( 33.71607969487701695, -17.27553485048664683, -7.545771892860997809 ) ) ;
#35707=CARTESIAN_POINT ( 'NONE',  ( 1.006457374325394838, 24.67265317861021501, -20.69366133597257118 ) ) ;
#35714=CARTESIAN_POINT ( 'NONE',  ( 11.19449165307062266, 21.93316151188967922, -19.27160384251886427 ) ) ;
#35718=CARTESIAN_POINT ( 'NONE',  ( -19.77774007911304821, 14.30023323257737466, -10.37717975262850878 ) ) ;
#35722=CARTESIAN_POINT ( 'NONE',  ( 9.805821007926871502, -18.55489467393325853, -26.22290329400297537 ) ) ;
#35724=CARTESIAN_POINT ( 'NONE',  ( 15.35452447619515226, 26.73442772235758014, -6.416210666809704755 ) ) ;
#35725=CARTESIAN_POINT ( 'NONE',  ( -22.52744239175981278, -0.1803094636421871677, -20.90349153980994501 ) ) ;
#35728=CARTESIAN_POINT ( 'NONE',  ( -15.11226011019654436, -14.18218723851762597, -27.77779782121918473 ) ) ;
#35729=CARTESIAN_POINT ( 'NONE',  ( 3.028292443394525524, -21.32411716264335766, -22.21865855438248971 ) ) ;
#35730=CARTESIAN_POINT ( 'NONE',  ( 11.12785985892924678, 17.21691741209329862, -29.99999999999999289 ) ) ;
#35731=CARTESIAN_POINT ( 'NONE',  ( 17.78979992564072887, 12.92841434147965352, -20.10125189250855726 ) ) ;
#35735=CARTESIAN_POINT ( 'NONE',  ( -4.114515543405717679, 20.32799847914411373, -27.75925566174262826 ) ) ;
#35742=CARTESIAN_POINT ( 'NONE',  ( -30.19601209477679760, 0.1621268579053716241, -8.299309318683974368 ) ) ;
#35745=CARTESIAN_POINT ( 'NONE',  ( 20.60227848500122860, -5.552195928352420928, -25.73354454585938811 ) ) ;
#35760=CARTESIAN_POINT ( 'NONE',  ( 18.93676227246565702, 16.79700351661384161, -7.901259146623853091 ) ) ;
#35761=CARTESIAN_POINT ( 'NONE',  ( 5.727250998068078580, 19.76148542614543047, -28.52014932781858292 ) ) ;
#35766=CARTESIAN_POINT ( 'NONE',  ( 9.819171776840725840, -18.04961070180578986, -28.69512037941552407 ) ) ;
#35770=CARTESIAN_POINT ( 'NONE',  ( -11.00327412694905860, 17.34993409992508973, -28.70683927363747401 ) ) ;
#35773=CARTESIAN_POINT ( 'NONE',  ( 12.95888722777509727, -25.15559516903838500, -10.68953037264193817 ) ) ;
#35778=CARTESIAN_POINT ( 'NONE',  ( -7.247758014959435613, 19.72005091410585464, -26.50610415850021795 ) ) ;
#35781=CARTESIAN_POINT ( 'NONE',  ( -34.24415449774322440, -5.469239270874415304, -6.781267690620076394 ) ) ;
#35784=CARTESIAN_POINT ( 'NONE',  ( 20.47879743316550005, 0.9320964914785054845, -29.34969434330313831 ) ) ;
#35789=CARTESIAN_POINT ( 'NONE',  ( -30.00917842038222005, 0.01052955857392639215, -9.237561733509775053 ) ) ;
#35792=CARTESIAN_POINT ( 'NONE',  ( 29.56647952434581583, -2.710646861654836925, -13.25517925932730456 ) ) ;
#35804=CARTESIAN_POINT ( 'NONE',  ( 2.680372758886228279, 20.41866721373630966, -28.46039174759823709 ) ) ;
#35808=CARTESIAN_POINT ( 'NONE',  ( 16.81687198955598461, -22.15028281434977231, -16.05891094166905475 ) ) ;
#35812=CARTESIAN_POINT ( 'NONE',  ( 14.89744943408475564, 25.91887218477155130, -9.702362698303520716 ) ) ;
#35814=CARTESIAN_POINT ( 'NONE',  ( -15.12259515852657898, 25.63742652657455778, -9.242452702712727231 ) ) ;
#35818=CARTESIAN_POINT ( 'NONE',  ( 14.56114463551361204, 24.89209121383319001, -11.60131081651779184 ) ) ;
#35820=CARTESIAN_POINT ( 'NONE',  ( 17.33150493693412031, -10.96591108411289639, -30.00000000000002842 ) ) ;
#35822=CARTESIAN_POINT ( 'NONE',  ( -10.60445392351956073, 17.59993408138762661, -28.69024928499496241 ) ) ;
#35824=CARTESIAN_POINT ( 'NONE',  ( -10.20341636066711288, -17.78360352085077878, -29.33359148140973005 ) ) ;
#35827=CARTESIAN_POINT ( 'NONE',  ( -33.68730855286997183, -13.89000784508904829, -9.301074370182135453 ) ) ;
#35828=CARTESIAN_POINT ( 'NONE',  ( -9.617329463714023419, -18.95265504179631932, -25.05348104573760537 ) ) ;
#35830=CARTESIAN_POINT ( 'NONE',  ( 14.60200688919959688, 18.24034312353848009, -18.75124519320161554 ) ) ;
#35832=CARTESIAN_POINT ( 'NONE',  ( 22.40999101807990712, 3.009793452745128661, -20.80770581881638392 ) ) ;
#35833=CARTESIAN_POINT ( 'NONE',  ( -1.829593030691901284E-15, 22.50000000000001066, 3.000000000000000000 ) ) ;
#35836=CARTESIAN_POINT ( 'NONE',  ( -25.30972341225729139, 0.2006976411555125572, -17.41501298532444864 ) ) ;
#35837=CARTESIAN_POINT ( 'NONE',  ( 30.64785752585394718, -0.7125550944224900984, -9.193437879178903316 ) ) ;
#35841=CARTESIAN_POINT ( 'NONE',  ( -28.74177917110700875, 1.753266042911047373, -8.316192635012841450 ) ) ;
#35842=CARTESIAN_POINT ( 'NONE',  ( -13.47223693944937040, 18.09844039693852125, -21.24786896499725231 ) ) ;
#35852=CARTESIAN_POINT ( 'NONE',  ( -21.24220381125994805, 5.046223848463253780, -22.05423595162513450 ) ) ;
#35855=CARTESIAN_POINT ( 'NONE',  ( 26.32663925810967953, -25.71384748841218837, -5.442504371432549171 ) ) ;
#35858=CARTESIAN_POINT ( 'NONE',  ( 11.64919678992194640, 19.63822387691775262, -21.57097631828376194 ) ) ;
#35862=CARTESIAN_POINT ( 'NONE',  ( -16.55555455799639830, 22.89925119996338765, -6.424656108638855834 ) ) ;
#35866=CARTESIAN_POINT ( 'NONE',  ( 14.76729391302192695, -25.81058457567449338, -9.710596626364806028 ) ) ;
#35869=CARTESIAN_POINT ( 'NONE',  ( 11.04758111719894309, 17.42002116339528683, -28.07786199837244112 ) ) ;
#35872=ORIENTED_EDGE ( 'NONE', *, *, #23047, .T. ) ;
#35873=CARTESIAN_POINT ( 'NONE',  ( -15.38296630468078874, 26.90060637120896558, -5.473630184351862660 ) ) ;
#35875=CARTESIAN_POINT ( 'NONE',  ( -15.19613505986383473, -26.28779615057171881, -8.296983900613629004 ) ) ;
#35878=CARTESIAN_POINT ( 'NONE',  ( -24.91495442474104749, -15.04743612541264852, -16.62452746883704791 ) ) ;
#35879=CARTESIAN_POINT ( 'NONE',  ( -8.832931388505667059, -24.56742532686079272, -10.78344481105500385 ) ) ;
#35880=CARTESIAN_POINT ( 'NONE',  ( 15.56695106341455848, 24.30445274633115815, -9.260401158391204035 ) ) ;
#35882=CARTESIAN_POINT ( 'NONE',  ( 20.64360361735735339, 8.470246920354872699, -19.02919037500957700 ) ) ;
#35883=CARTESIAN_POINT ( 'NONE',  ( 12.05832241004688399, 18.99596958976722760, -21.04195414767209726 ) ) ;
#35887=CARTESIAN_POINT ( 'NONE',  ( -20.74499114794467758, -1.156592509646555689, -27.31797897823820520 ) ) ;
#35893=ADVANCED_FACE ( 'NONE', ( #16933 ), #26267, .F. ) ;
#35895=CARTESIAN_POINT ( 'NONE',  ( 26.22005807680820766, -12.44079363307010233, -16.63921512830654237 ) ) ;
#35896=AXIS2_PLACEMENT_3D ( 'NONE', #20324, #32923, #11177 ) ;
#35904=CARTESIAN_POINT ( 'NONE',  ( 0.2213127261196708995, 20.90796579412245748, -26.96645221465433551 ) ) ;
#35905=DIRECTION ( 'NONE',  ( 1.000000000000000000, 0.000000000000000000, 0.000000000000000000 ) ) ;
#35911=CARTESIAN_POINT ( 'NONE',  ( 14.65960527224459931, 28.71189413793838341, -6.386546476000780181 ) ) ;
#35914=CARTESIAN_POINT ( 'NONE',  ( -18.68060247292710585, 14.65156323798503912, -13.87922052841179799 ) ) ;
#35918=CARTESIAN_POINT ( 'NONE',  ( 15.26849416126754910, -26.39863181468341580, -7.827248033921830661 ) ) ;
#35920=CARTESIAN_POINT ( 'NONE',  ( 15.40660648310854164, 26.81700542816128063, -5.000000000000000000 ) ) ;
#35921=CARTESIAN_POINT ( 'NONE',  ( 9.163310636333564574, 20.63632441393291117, -20.55760979252978871 ) ) ;
#35925=CARTESIAN_POINT ( 'NONE',  ( -14.94827155352230186, -14.02787326271796609, -29.23873448612896553 ) ) ;
#35926=CARTESIAN_POINT ( 'NONE',  ( 4.439926597751906456, -20.64563978286073365, -24.32161315903661247 ) ) ;
#35927=CARTESIAN_POINT ( 'NONE',  ( 11.88552478615052976, 18.71945594169985938, -22.76728644064645124 ) ) ;
#35928=CARTESIAN_POINT ( 'NONE',  ( 19.02469128737116577, 14.03524138465703253, -13.88975380088736955 ) ) ;
#35932=CARTESIAN_POINT ( 'NONE',  ( -7.388453759928180098, 36.32445320202015893, -7.146513852312973647 ) ) ;
#35940=CARTESIAN_POINT ( 'NONE',  ( -29.94001474276964814, 0.4362189444618576606, -8.302034482558056538 ) ) ;
#35943=CARTESIAN_POINT ( 'NONE',  ( 31.03616632986720347, -9.319775343359541608, -12.97620689962225704 ) ) ;
#35955=VERTEX_POINT ( 'NONE', #5334 ) ;
#35957=CARTESIAN_POINT ( 'NONE',  ( -13.18357918683125618, -15.75518424256909888, -30.00000000000001066 ) ) ;
#35960=CARTESIAN_POINT ( 'NONE',  ( 19.07008944147191443, 16.95185708702321747, -5.000000000000002665 ) ) ;
#35961=CARTESIAN_POINT ( 'NONE',  ( 7.014095819933510612, 19.62255229036581738, -27.16548337421515669 ) ) ;
#35966=CARTESIAN_POINT ( 'NONE',  ( 13.60193512794777249, -23.64579311371437598, -14.45468143796861327 ) ) ;
#35972=CARTESIAN_POINT ( 'NONE',  ( -14.93437990693434614, 25.80124217664804931, -9.708838696810092372 ) ) ;
#35975=CARTESIAN_POINT ( 'NONE',  ( 13.26340735356318135, -25.63066692232520793, -9.260339685793301356 ) ) ;
#35979=CARTESIAN_POINT ( 'NONE',  ( -11.90375846996125020, 33.19065507634929446, -5.449804871099760639 ) ) ;
#35983=CARTESIAN_POINT ( 'NONE',  ( -21.43593173410406294, -3.250475320730803031, -24.59978728874802201 ) ) ;
#35986=CARTESIAN_POINT ( 'NONE',  ( 26.47025118594213922, 0.3293273261899055115, -15.45460282459215584 ) ) ;
#35991=CARTESIAN_POINT ( 'NONE',  ( -27.13259105340829080, 0.2465074430099665204, -14.47731736851761930 ) ) ;
#35995=CARTESIAN_POINT ( 'NONE',  ( 26.85449993285726578, -3.950704618538266821, -16.99524324133061626 ) ) ;
#36009=CARTESIAN_POINT ( 'NONE',  ( 2.866343458708493497, 21.79950405809651315, -24.26554964526188840 ) ) ;
#36012=CARTESIAN_POINT ( 'NONE',  ( 16.47321826383852184, -22.95941082514774578, -15.14534849247683646 ) ) ;
#36018=CARTESIAN_POINT ( 'NONE',  ( 15.19538877031547308, 26.53216222070651398, -7.823603041336555819 ) ) ;
#36021=CARTESIAN_POINT ( 'NONE',  ( -13.18473458846506396, 21.24086736371716455, -17.47963371193705129 ) ) ;
#36024=CARTESIAN_POINT ( 'NONE',  ( 13.26563377173174096, 22.13583170298742075, -16.45275615339405206 ) ) ;
#36026=CARTESIAN_POINT ( 'NONE',  ( 17.65215317207318080, -10.44170805849464401, -30.00000000000002842 ) ) ;
#36028=CARTESIAN_POINT ( 'NONE',  ( -10.79848222091381871, 17.83570280373058026, -26.79973138845655711 ) ) ;
#36030=CARTESIAN_POINT ( 'NONE',  ( -18.36895873238599108, -27.24750037505589262, -4.999999999999997335 ) ) ;
#36032=ORIENTED_EDGE ( 'NONE', *, *, #15705, .T. ) ;
#36033=CARTESIAN_POINT ( 'NONE',  ( -20.73329258327116875, -7.162834230695762194, -24.32145964058944188 ) ) ;
#36034=CARTESIAN_POINT ( 'NONE',  ( -14.77796826032629696, -26.49119245572812531, -6.417790910078942090 ) ) ;
#36037=CARTESIAN_POINT ( 'NONE',  ( 22.21443852417969111, 2.286644819169600051, -21.81262643821637681 ) ) ;
#36041=CARTESIAN_POINT ( 'NONE',  ( -20.97617324094073510, 0.7433129137733408554, -26.21918480705897991 ) ) ;
#36043=CARTESIAN_POINT ( 'NONE',  ( 20.49959133494802543, 0.2219702378425635336, -30.00000000000000000 ) ) ;
#36046=CARTESIAN_POINT ( 'NONE',  ( -29.21107446086027082, 1.733986180571662095, -5.000000000000000000 ) ) ;
#36048=CARTESIAN_POINT ( 'NONE',  ( -21.88444403592365362, 6.126538576424530369, -21.50719306941233455 ) ) ;
#36057=CARTESIAN_POINT ( 'NONE',  ( -25.41367398360687346, 5.264759306010887485, -10.30541271499615164 ) ) ;
#36060=CARTESIAN_POINT ( 'NONE',  ( 24.21332198295975502, -23.75827105196518474, -11.15521848907045666 ) ) ;
#36063=CARTESIAN_POINT ( 'NONE',  ( 10.79245250836826564, 17.68824287289717034, -27.42597519482002610 ) ) ;
#36066=CARTESIAN_POINT ( 'NONE',  ( -13.63746324345819261, 16.03261875762171584, -25.28435114513372284 ) ) ;
#36070=CARTESIAN_POINT ( 'NONE',  ( 12.14281235004362358, 19.90984008834854890, -20.54315895355848554 ) ) ;
#36072=CARTESIAN_POINT ( 'NONE',  ( 12.39413036303999149, 20.48625930257307104, -19.49701620399659419 ) ) ;
#36075=CARTESIAN_POINT ( 'NONE',  ( -15.11182017094948016, 26.49105686739811460, -8.289746988309037334 ) ) ;
#36077=CARTESIAN_POINT ( 'NONE',  ( -9.506566060136700358, -18.16246691004805314, -30.00000000000000000 ) ) ;
#36080=CARTESIAN_POINT ( 'NONE',  ( -31.33135991916500984, -16.39895654298046423, -11.06949826535703352 ) ) ;
#36081=CARTESIAN_POINT ( 'NONE',  ( -8.170773189261824498, -23.31984667172876868, -14.74591960211686725 ) ) ;
#36083=CARTESIAN_POINT ( 'NONE',  ( 15.93428740759538265, 25.01899822204553203, -5.474102051487178322 ) ) ;
#36086=CARTESIAN_POINT ( 'NONE',  ( 19.41880252833811227, 6.610239277501288591, -29.41827274932495584 ) ) ;
#36089=DIRECTION ( 'NONE',  ( -1.000000000000000000, 0.000000000000000000, 0.000000000000000000 ) ) ;
#36093=CARTESIAN_POINT ( 'NONE',  ( -32.26688085667248629, -1.675871053962237012, -5.926420720323367419 ) ) ;
#36094=CARTESIAN_POINT ( 'NONE',  ( 20.82064840824700624, 0.7693617283651914551, -26.82585393716254529 ) ) ;
#36108=CARTESIAN_POINT ( 'NONE',  ( 0.4084515277692671864, 38.10027764858106281, -7.117403505773802763 ) ) ;
#36115=CARTESIAN_POINT ( 'NONE',  ( 14.46172013027408632, 28.25976373080003867, -8.225629111251091530 ) ) ;
#36116=CARTESIAN_POINT ( 'NONE',  ( -32.33143948542088708, 1.358872982498823268, -5.000000000000000888 ) ) ;
#36117=ORIENTED_EDGE ( 'NONE', *, *, #9131, .F. ) ;
#36118=CARTESIAN_POINT ( 'NONE',  ( -16.41392363336672844, 12.39559230606829487, -28.28840681818169145 ) ) ;
#36121=CARTESIAN_POINT ( 'NONE',  ( 15.45930891439913601, -26.66055752704448523, -6.416469317147711848 ) ) ;
#36122=DIRECTION ( 'NONE',  ( -1.000000000000000000, 0.000000000000000000, 0.000000000000000000 ) ) ;
#36123=CARTESIAN_POINT ( 'NONE',  ( 15.22307974005524223, 26.43793140921028240, -7.826725321211265296 ) ) ;
#36127=CARTESIAN_POINT ( 'NONE',  ( -25.79871209414094935, -22.89210493903414090, -11.11974611591713291 ) ) ;
#36128=CARTESIAN_POINT ( 'NONE',  ( 1.767497973323724381, -24.39642072439984943, -9.396636978634532511 ) ) ;
#36129=CARTESIAN_POINT ( 'NONE',  ( 15.52046154931812261, 26.41174381453696540, -5.000000000000000888 ) ) ;
#36130=CARTESIAN_POINT ( 'NONE',  ( 18.90886957614733177, 10.57106918749075319, -21.18213341435799180 ) ) ;
#36133=CARTESIAN_POINT ( 'NONE',  ( -5.270476743073104764, 25.91271121330065696, -18.72494855390057467 ) ) ;
#36142=CARTESIAN_POINT ( 'NONE',  ( -20.95633139473599726, 0.9343472425770981138, -26.23583468170135546 ) ) ;
#36144=CARTESIAN_POINT ( 'NONE',  ( 24.22071271199023101, -7.313483937193986151, -19.78735341019923055 ) ) ;
#36157=CARTESIAN_POINT ( 'NONE',  ( 16.76787866856672338, 15.62184907137590706, -17.91620485821478326 ) ) ;
#36159=CARTESIAN_POINT ( 'NONE',  ( 6.908205946113893603, 19.31174812457788548, -29.26867246192825078 ) ) ;
#36162=CARTESIAN_POINT ( 'NONE',  ( -22.16749550643533340, 10.73470648441587905, -8.406596372856219190 ) ) ;
#36164=FACE_OUTER_BOUND ( 'NONE', #37769, .T. ) ;
#36165=CARTESIAN_POINT ( 'NONE',  ( 13.94326871252339473, -24.14806653283149629, -13.49309882371043834 ) ) ;
#36166=CARTESIAN_POINT ( 'NONE',  ( 37.48538792151179422, -11.24999995791135809, -5.000000000000002665 ) ) ;
#36169=EDGE_CURVE ( 'NONE', #14281, #16948, #12426, .T. ) ;
#36171=CARTESIAN_POINT ( 'NONE',  ( -13.20806276164241488, 22.23819342938818622, -16.44376970385624759 ) ) ;
#36173=CARTESIAN_POINT ( 'NONE',  ( 13.64569075595249181, -26.22458777178208322, -6.419671810663616363 ) ) ;
#36178=CARTESIAN_POINT ( 'NONE',  ( -12.21035293360103147, 31.03120155201804309, -9.465151556475316141 ) ) ;
#36184=CARTESIAN_POINT ( 'NONE',  ( 30.65966444727390794, 0.03748699155148955270, -6.888076747643670394 ) ) ;
#36189=CARTESIAN_POINT ( 'NONE',  ( -29.97333235930364381, 0.04935946867576600922, -9.238760947532812295 ) ) ;
#36193=CARTESIAN_POINT ( 'NONE',  ( 21.43667605784225572, -3.053840757090042324, -24.61930641589043489 ) ) ;
#36211=CARTESIAN_POINT ( 'NONE',  ( 3.933113624042559930, 20.35544397462496846, -27.75572121666948178 ) ) ;
#36214=CARTESIAN_POINT ( 'NONE',  ( 14.50103858733138829, -20.35908921518062087, -19.15145559871423941 ) ) ;
#36220=CARTESIAN_POINT ( 'NONE',  ( 11.39842292676588720, 18.51123022929508721, -23.84032446260234295 ) ) ;
#36224=CARTESIAN_POINT ( 'NONE',  ( -11.34469411494776203, 17.22161296595826485, -28.09528742440320670 ) ) ;
#36228=CARTESIAN_POINT ( 'NONE',  ( 15.42070031560629317, 26.50090741082905055, -6.417193677922045758 ) ) ;
#36230=CARTESIAN_POINT ( 'NONE',  ( 18.12106542394759501, -11.46725993656733777, -25.57869145427667945 ) ) ;
#36233=CARTESIAN_POINT ( 'NONE',  ( -13.50527592257643050, 23.96582696250451860, -14.41748651284650151 ) ) ;
#36234=CARTESIAN_POINT ( 'NONE',  ( -32.33143948541789570, 1.358872982501806215, -5.000000000000000000 ) ) ;
#36235=CARTESIAN_POINT ( 'NONE',  ( -10.71436039581699795, -17.92443767809337629, -26.74123038190443324 ) ) ;
#36240=CARTESIAN_POINT ( 'NONE',  ( -27.04735894903886972, -9.297324301607403640, -16.71430700021294413 ) ) ;
#36241=CARTESIAN_POINT ( 'NONE',  ( -14.28239120255770622, -25.56022528091948587, -10.18897211997865782 ) ) ;
#36244=CARTESIAN_POINT ( 'NONE',  ( 20.40557468639088157, 2.415499751543392914, -28.75714396012276097 ) ) ;
#36248=CARTESIAN_POINT ( 'NONE',  ( -29.65891584835985384, -0.01954106857342741491, -10.17503558318995083 ) ) ;
#36249=CARTESIAN_POINT ( 'NONE',  ( 31.65879457089920024, -0.9929091283696672710, -6.398057018500724169 ) ) ;
#36252=CARTESIAN_POINT ( 'NONE',  ( -20.74417435968310031, 3.585152392585164272, -25.26646650636820013 ) ) ;
#36263=CARTESIAN_POINT ( 'NONE',  ( -19.89457789833269885, 5.001894110080484346, -29.40556248342900147 ) ) ;
#36266=CARTESIAN_POINT ( 'NONE',  ( 21.45659587343440222, -22.35059298105742798, -13.95210435312599273 ) ) ;
#36269=CARTESIAN_POINT ( 'NONE',  ( 14.72331344930747932, 25.96238726373383088, -10.15914416928072050 ) ) ;
#36272=CARTESIAN_POINT ( 'NONE',  ( -14.74746392996318356, 18.03178186202489641, -18.77012448782567944 ) ) ;
#36276=CARTESIAN_POINT ( 'NONE',  ( 15.30701244550224338, 26.47243815946491452, -7.358024508618584036 ) ) ;
#36280=CARTESIAN_POINT ( 'NONE',  ( -14.67353854144589675, 25.58823882037592412, -10.64067760867671808 ) ) ;
#36282=CARTESIAN_POINT ( 'NONE',  ( -15.51079060825593281, -26.67363690140799903, -6.415640535509750997 ) ) ;
#36284=CIRCLE ( 'NONE', #12826, 16.00000000000000000 ) ;
#36286=CARTESIAN_POINT ( 'NONE',  ( -30.51621992633454639, -15.97226344309796886, -11.97627014025983705 ) ) ;
#36287=CARTESIAN_POINT ( 'NONE',  ( -7.977729298563027704, -22.95874574334327889, -15.75516193211872640 ) ) ;
#36288=CARTESIAN_POINT ( 'NONE',  ( 12.93365880273942281, 18.25915373805785791, -21.78730442601257167 ) ) ;
#36290=CARTESIAN_POINT ( 'NONE',  ( 20.83270517224113760, 6.805427843616754124, -21.08448443926039317 ) ) ;
#36296=CARTESIAN_POINT ( 'NONE',  ( -23.01684666815623714, -0.4182225803685448717, -21.47969933400415954 ) ) ;
#36297=CARTESIAN_POINT ( 'NONE',  ( 30.96479225765983045, -0.1042645752839200801, -5.473789633946161359 ) ) ;
#36301=CARTESIAN_POINT ( 'NONE',  ( 18.07620401364302865, 24.68088026512193167, -13.58461195433497082 ) ) ;
#36302=CARTESIAN_POINT ( 'NONE',  ( -75.15099915297791711, 43.38844959084113384, 0.000000000000000000 ) ) ;
#36308=CARTESIAN_POINT ( 'NONE',  ( 1.569683897492700098, 38.21696230019209395, -6.697046784752907378 ) ) ;
#36316=CARTESIAN_POINT ( 'NONE',  ( 14.71880540954476935, 27.90283997931214088, -7.780570891888019425 ) ) ;
#36319=CARTESIAN_POINT ( 'NONE',  ( -18.78764273638527982, 16.18379394525580039, -10.35842720535364592 ) ) ;
#36322=CARTESIAN_POINT ( 'NONE',  ( 10.55467174157632293, -19.57048749257938525, -22.73257509897530326 ) ) ;
#36323=CARTESIAN_POINT ( 'NONE',  ( 12.13489577391684904, 19.91918273965267261, -20.54176214682885515 ) ) ;
#36324=CARTESIAN_POINT ( 'NONE',  ( 15.40434907611582638, 26.82505288294843027, -5.474005114572026542 ) ) ;
#36325=CARTESIAN_POINT ( 'NONE',  ( -3.485571585149886520, -11.25000000000002132, 10.00000000000000000 ) ) ;
#36327=CARTESIAN_POINT ( 'NONE',  ( -20.41145111406656198, -16.99166856771202205, -18.69276795763255805 ) ) ;
#36328=CARTESIAN_POINT ( 'NONE',  ( 3.253891525658406447, -22.11403326693343985, -19.03245994517476092 ) ) ;
#36329=CARTESIAN_POINT ( 'NONE',  ( 11.29606703750313912, 17.49295334550439307, -26.84622463755728106 ) ) ;
#36330=CARTESIAN_POINT ( 'NONE',  ( 18.06948145980227949, 10.11918264026371439, -26.62323384584303909 ) ) ;
#36334=CARTESIAN_POINT ( 'NONE',  ( -4.760937472852409869, 20.33112424556681574, -27.05855014857421637 ) ) ;
#36342=CARTESIAN_POINT ( 'NONE',  ( -27.00797239653981663, 0.4251854506619431873, -14.48925554260671689 ) ) ;
#36344=CARTESIAN_POINT ( 'NONE',  ( 26.03424934262190504, -8.709753677229443269, -17.70432680259551361 ) ) ;
#36345=ADVANCED_FACE ( 'NONE', ( #6916 ), #19318, .T. ) ;
#36359=CARTESIAN_POINT ( 'NONE',  ( 17.24737218078871592, 14.85018931016522181, -17.94678984768380303 ) ) ;
#36360=CARTESIAN_POINT ( 'NONE',  ( 8.110597763130101612, 20.77001312407615075, -23.39814370609576244 ) ) ;
#36362=CARTESIAN_POINT ( 'NONE',  ( -21.25246432144205500, 11.48441715314585387, -10.88392780175655794 ) ) ;
#36365=CARTESIAN_POINT ( 'NONE',  ( 10.55460110364784931, -19.04761602628894934, -23.81187091824480362 ) ) ;
#36368=CARTESIAN_POINT ( 'NONE',  ( 19.79815887584821610, 19.84782313723624370, -5.000000000000007994 ) ) ;
#36369=CARTESIAN_POINT ( 'NONE',  ( -15.36269874125315482, 26.70556469616796846, -6.416677824283240739 ) ) ;
#36370=CARTESIAN_POINT ( 'NONE',  ( -14.44668725894448436, -16.26647643531120124, -24.50689636315220810 ) ) ;
#36371=CARTESIAN_POINT ( 'NONE',  ( 13.43210918908202878, -25.89342552787512730, -8.311467949088584106 ) ) ;
#36377=CARTESIAN_POINT ( 'NONE',  ( -7.743198174825847602, 19.19541131226637276, -27.89444138947942875 ) ) ;
#36383=CARTESIAN_POINT ( 'NONE',  ( 30.86596729670053563, -0.003225903683491773612, -5.000000000000000000 ) ) ;
#36385=DIRECTION ( 'NONE',  ( 0.000000000000000000, 0.000000000000000000, 1.000000000000000000 ) ) ;
#36388=CARTESIAN_POINT ( 'NONE',  ( -21.70627603254861526, 0.7432028481183311497, -23.85585032862205423 ) ) ;
#36391=CARTESIAN_POINT ( 'NONE',  ( 32.67224823038714732, -4.906388482558933894, -9.920036700255655759 ) ) ;
#36404=CARTESIAN_POINT ( 'NONE',  ( 7.091416633034167027, 36.58341554298284137, -6.718649601333577692 ) ) ;
#36408=CARTESIAN_POINT ( 'NONE',  ( 11.91734804082858012, -17.02703054535963290, -27.27743194981858821 ) ) ;
#36413=CARTESIAN_POINT ( 'NONE',  ( 11.00268105793074547, 17.54964049701253259, -27.44232077932614899 ) ) ;
#36415=CARTESIAN_POINT ( 'NONE',  ( -15.33310310740069227, 26.06452538537273966, -7.829622284288262790 ) ) ;
#36418=CARTESIAN_POINT ( 'NONE',  ( 15.06272762976659330, 25.82752587005803235, -9.240082175145575505 ) ) ;
#36420=CARTESIAN_POINT ( 'NONE',  ( 24.06311164388931445, -14.23786492898669387, -17.59357969373190755 ) ) ;
#36423=CARTESIAN_POINT ( 'NONE',  ( -11.60894466518139545, 19.67965406879041623, -21.56349800617989132 ) ) ;
#36424=CYLINDRICAL_SURFACE ( 'NONE', #4337, 60.00000000000014211 ) ;
#36425=CARTESIAN_POINT ( 'NONE',  ( -10.48684353440000194, -17.61503585894356050, -30.00000000000000000 ) ) ;
#36429=CARTESIAN_POINT ( 'NONE',  ( -35.35897274256637957, -12.18463282932507852, -6.291972826754448356 ) ) ;
#36430=CARTESIAN_POINT ( 'NONE',  ( -15.03672417963925056, -26.50613305951797827, -6.888625959290687106 ) ) ;
#36433=CARTESIAN_POINT ( 'NONE',  ( 24.26573961589400952, 2.169758022266998765, -17.60781658105700487 ) ) ;
#36437=CARTESIAN_POINT ( 'NONE',  ( -30.95087757567503672, -0.08989953764334629449, -5.000000000000000000 ) ) ;
#36439=CARTESIAN_POINT ( 'NONE',  ( 27.05815561153594473, -0.6001877338740869705, -15.34801442178561359 ) ) ;
#36444=CARTESIAN_POINT ( 'NONE',  ( -24.48240760914098502, 2.712249908169665158, -16.64270392758168526 ) ) ;
#36454=DIRECTION ( 'NONE',  ( -0.000000000000000000, -0.000000000000000000, 1.000000000000000000 ) ) ;
#36456=CARTESIAN_POINT ( 'NONE',  ( -23.92566527182959391, 5.176061040404443148, -14.76782440308691591 ) ) ;
#36458=DIRECTION ( 'NONE',  ( -1.000000000000000000, 0.000000000000000000, 0.000000000000000000 ) ) ;
#36459=CARTESIAN_POINT ( 'NONE',  ( 18.70657072468925364, -18.32550425351821488, -18.79420699992576971 ) ) ;
#36461=CARTESIAN_POINT ( 'NONE',  ( 10.68641602773397636, 17.65275450399973423, -28.05634532095279710 ) ) ;
#36464=CARTESIAN_POINT ( 'NONE',  ( -14.03330550907330654, 18.32430351830364756, -19.75759142101557586 ) ) ;
#36467=CARTESIAN_POINT ( 'NONE',  ( 11.20058424733595892, 17.74459894083964784, -26.22661702102002224 ) ) ;
#36471=CARTESIAN_POINT ( 'NONE',  ( -15.18975761229610022, 26.55092571743323404, -7.822985543115054341 ) ) ;
#36474=CARTESIAN_POINT ( 'NONE',  ( -11.55840277251474646, -20.97515074911826360, -19.49524396482431143 ) ) ;
#36477=CARTESIAN_POINT ( 'NONE',  ( -18.11135944020848498, -10.93062044766753793, -26.25495776335099762 ) ) ;
#36478=CARTESIAN_POINT ( 'NONE',  ( -13.30200433025800777, -25.37444367340206242, -10.20725642727310678 ) ) ;
#36480=CARTESIAN_POINT ( 'NONE',  ( 11.83150832767071314, 16.74097710667822270, -30.00000000000000000 ) ) ;
#36482=CARTESIAN_POINT ( 'NONE',  ( 22.91801202536632687, 6.219164452797125264, -15.83068595770922826 ) ) ;
#36485=CARTESIAN_POINT ( 'NONE',  ( 0.000000000000000000, 22.50000000000000355, 10.00000000000000000 ) ) ;
#36488=CARTESIAN_POINT ( 'NONE',  ( -22.50773814093716396, -0.7003419581363549140, -22.56284863701274190 ) ) ;
#36489=CARTESIAN_POINT ( 'NONE',  ( 20.52860846656784588, 0.8226844751264725808, -28.70573514187030995 ) ) ;
#36494=CARTESIAN_POINT ( 'NONE',  ( 21.88499642459564143, -5.528038495964486820, -29.99999999999998224 ) ) ;
#36503=CARTESIAN_POINT ( 'NONE',  ( 1.293490870016113403, 31.31656944015267996, -14.73212527803245919 ) ) ;
#36510=CARTESIAN_POINT ( 'NONE',  ( 14.65877742485253421, 27.77006656560355680, -8.242821808329072297 ) ) ;
#36514=CARTESIAN_POINT ( 'NONE',  ( -16.37425825659163792, 12.35560620482834970, -30.00000000000000000 ) ) ;
#36517=CARTESIAN_POINT ( 'NONE',  ( 15.06737418716398480, -26.14303779321338084, -8.767816294897599505 ) ) ;
#36518=CARTESIAN_POINT ( 'NONE',  ( 15.39919595897969806, 26.75075905497483930, -5.946079338151666782 ) ) ;
#36519=CARTESIAN_POINT ( 'NONE',  ( 14.83164354014592945, 25.63566593113468173, -10.17862006668016051 ) ) ;
#36523=CARTESIAN_POINT ( 'NONE',  ( -29.42985357383858869, -23.05064539992688921, -7.560940416845337353 ) ) ;
#36524=CARTESIAN_POINT ( 'NONE',  ( 3.957494336073486441, -24.62814106778900225, -8.398072415613651032 ) ) ;
#36525=CARTESIAN_POINT ( 'NONE',  ( 11.74988495535431454, 18.20669567406710954, -23.89381587855401534 ) ) ;
#36526=CARTESIAN_POINT ( 'NONE',  ( 20.21597881006783837, 12.43147293057613645, -12.89012422323875917 ) ) ;
#36529=CARTESIAN_POINT ( 'NONE',  ( -4.218276626635449666, 29.63384946082300431, -15.71993721405139155 ) ) ;
#36537=CARTESIAN_POINT ( 'NONE',  ( -25.10967418331198431, 0.5688158262986504621, -17.45731339471036137 ) ) ;
#36538=CARTESIAN_POINT ( 'NONE',  ( 19.70705905309527139, -5.958174894697001456, -28.49491022416014019 ) ) ;
#36553=CARTESIAN_POINT ( 'NONE',  ( 17.60659027557944967, -14.36865807356775626, -23.06510994001489578 ) ) ;
#36554=CARTESIAN_POINT ( 'NONE',  ( 20.03430053822841828, 14.93931088505822657, -5.965758641065874279 ) ) ;
#36556=CARTESIAN_POINT ( 'NONE',  ( 12.40530672973724080, 32.54280113045124523, -5.895856452077529397 ) ) ;
#36558=CARTESIAN_POINT ( 'NONE',  ( -21.55543886414327304, 11.63864511105562194, -8.900058298306362303 ) ) ;
#36561=CARTESIAN_POINT ( 'NONE',  ( 15.52008768824105545, -26.55333232259659582, -7.352602181182319008 ) ) ;
#36563=CARTESIAN_POINT ( 'NONE',  ( 13.47223693944937750, 18.09844039693851769, -30.00000000000000355 ) ) ;
#36564=CARTESIAN_POINT ( 'NONE',  ( -15.16325337730098255, 26.31972413366512242, -8.296376571532537270 ) ) ;
#36566=CARTESIAN_POINT ( 'NONE',  ( -23.62391352436328873, -26.37202438933310589, -7.195775402117879693 ) ) ;
#36567=CARTESIAN_POINT ( 'NONE',  ( 10.73433329256054414, -21.08021252179972294, -19.58150332943896643 ) ) ;
#36572=CARTESIAN_POINT ( 'NONE',  ( -11.83993818029857437, 32.97031935882627351, -6.772281498610635886 ) ) ;
#36578=CARTESIAN_POINT ( 'NONE',  ( 27.08975123792179218, 0.3078043105649791999, -14.48142009230936900 ) ) ;
#36584=CARTESIAN_POINT ( 'NONE',  ( -20.96866610389652053, 0.8170365396961356552, -26.22569017582818063 ) ) ;
#36587=CARTESIAN_POINT ( 'NONE',  ( 24.19774762110479926, -2.790396721216801268, -20.13477434463229798 ) ) ;
#36603=CARTESIAN_POINT ( 'NONE',  ( 3.318832056366368022, 20.47935037984655793, -27.74009767284220729 ) ) ;
#36607=CARTESIAN_POINT ( 'NONE',  ( 12.27390640609045036, -16.43329545370340838, -29.28898356251528412 ) ) ;
#36612=CARTESIAN_POINT ( 'NONE',  ( 14.25784677919622823, 24.55947563112205145, -12.54307605572578055 ) ) ;
#36615=CARTESIAN_POINT ( 'NONE',  ( -11.20756347206190284, 17.73954208893731277, -26.22736157229892839 ) ) ;
#36617=CARTESIAN_POINT ( 'NONE',  ( 15.14201655615061526, -26.36804160454520485, -7.828362067540088454 ) ) ;
#36619=CARTESIAN_POINT ( 'NONE',  ( 11.07485645340150171, 17.25102576792224340, -29.35029984720032914 ) ) ;
#36621=CARTESIAN_POINT ( 'NONE',  ( 22.67567822676405953, -14.36290881944746900, -18.61438165153855095 ) ) ;
#36623=CARTESIAN_POINT ( 'NONE',  ( -14.29471368831881328, 25.61313551457574178, -11.55151809035900712 ) ) ;
#36625=CARTESIAN_POINT ( 'NONE',  ( -17.10877210688781958, -26.84738589896849703, -7.313269270788000043 ) ) ;
#36627=DIRECTION ( 'NONE',  ( 0.000000000000000000, 0.000000000000000000, 1.000000000000000000 ) ) ;
#36630=CARTESIAN_POINT ( 'NONE',  ( -35.25710161250010799, -11.00445477990710685, -6.726159309538959796 ) ) ;
#36632=CARTESIAN_POINT ( 'NONE',  ( -15.13531929286639155, -26.65245416579944759, -5.000000000000000888 ) ) ;
#36635=CARTESIAN_POINT ( 'NONE',  ( 20.86090429746450781, 3.082049809194417289, -25.22830055382215875 ) ) ;
#36639=CARTESIAN_POINT ( 'NONE',  ( -30.84155282226171124, -0.08171445749998075547, -6.415951416867066825 ) ) ;
#36641=CARTESIAN_POINT ( 'NONE',  ( 31.13255865061531935, -1.317985051374632066, -9.160379792037252500 ) ) ;
#36644=CARTESIAN_POINT ( 'NONE',  ( -22.04274155920867884, 2.809314319882194599, -21.86559244833277305 ) ) ;
#36653=CARTESIAN_POINT ( 'NONE',  ( -2.485571585149885632, -11.24999999999987566, 10.00000000000000000 ) ) ;
#36656=CARTESIAN_POINT ( 'NONE',  ( -23.86420076115572186, 7.970790765993674754, -8.878367169149885996 ) ) ;
#36659=CARTESIAN_POINT ( 'NONE',  ( 15.51366702551998955, -14.30026934863555788, -26.35746096789312176 ) ) ;
#36661=CARTESIAN_POINT ( 'NONE',  ( 11.95885763855134343, 20.12759201311160950, -20.50636973948041586 ) ) ;
#36664=CARTESIAN_POINT ( 'NONE',  ( -13.78067611128539838, 16.29607663636611647, -24.15683527709576239 ) ) ;
#36667=CARTESIAN_POINT ( 'NONE',  ( 12.94909081049822142, 21.61942785653063126, -17.44119972322781109 ) ) ;
#36671=CARTESIAN_POINT ( 'NONE',  ( -14.89167003689908775, 25.93687804966682364, -9.701378797208148441 ) ) ;
#36673=CARTESIAN_POINT ( 'NONE',  ( -13.03749113462529685, -23.09334588019250489, -15.44824872094964796 ) ) ;
#36676=AXIS2_PLACEMENT_3D ( 'NONE', #31720, #25614, #10187 ) ;
#36677=CARTESIAN_POINT ( 'NONE',  ( -34.06221145678576079, -17.84677894165469070, -5.435607523623667170 ) ) ;
#36678=CARTESIAN_POINT ( 'NONE',  ( -7.489852218780842286, -19.16649717563461408, -28.77838134633300626 ) ) ;
#36679=CYLINDRICAL_SURFACE ( 'NONE', #24790, 60.00000000000001421 ) ;
#36680=CARTESIAN_POINT ( 'NONE',  ( 13.62177027565629395, 19.65269395691544574, -18.61040937102566772 ) ) ;
#36683=CARTESIAN_POINT ( 'NONE',  ( 21.51332232471817818, 6.076221697413749290, -19.98667434612283955 ) ) ;
#36690=CARTESIAN_POINT ( 'NONE',  ( -31.63647013363080873, -0.8270238094956997577, -5.469293166058980304 ) ) ;
#36691=CARTESIAN_POINT ( 'NONE',  ( 20.48330953517068664, 0.8273339926270942835, -30.00000000000000000 ) ) ;
#36706=CARTESIAN_POINT ( 'NONE',  ( 3.705883046374359946, 36.09340752835787214, -9.737407412482861346 ) ) ;
#36714=CARTESIAN_POINT ( 'NONE',  ( 14.49954575914088117, 27.42131279283395529, -9.169623025717175580 ) ) ;
#36717=CARTESIAN_POINT ( 'NONE',  ( -18.00665338107467051, 15.31517184407994669, -14.87167487327246640 ) ) ;
#36719=CIRCLE ( 'NONE', #10757, 17.00000000000000000 ) ;
#36721=CARTESIAN_POINT ( 'NONE',  ( 9.786533863580281434, -18.56354127006651211, -26.22476242672100000 ) ) ;
#36722=CARTESIAN_POINT ( 'NONE',  ( -12.11431921870781281, -16.53859995802357474, -29.29246340261923720 ) ) ;
#36724=CARTESIAN_POINT ( 'NONE',  ( 15.27973808755479723, 26.56710540162124801, -7.356736264727379293 ) ) ;
#36729=CARTESIAN_POINT ( 'NONE',  ( -28.85413502746283498, -22.61874590850457523, -8.864180790608637395 ) ) ;
#36730=CARTESIAN_POINT ( 'NONE',  ( 1.335132817696313978, -21.21848675767797587, -23.33513061438837610 ) ) ;
#36731=CARTESIAN_POINT ( 'NONE',  ( 15.02468189385244024, 25.06093797422134273, -10.19064726329248138 ) ) ;
#36733=CARTESIAN_POINT ( 'NONE',  ( 22.21982769557913784, 11.10346373912405049, -5.482723809593267106 ) ) ;
#36735=CARTESIAN_POINT ( 'NONE',  ( -5.141937788641745222, 36.05078749574169450, -9.302716111124565757 ) ) ;
#36737=CARTESIAN_POINT ( 'NONE',  ( -20.24687895915023716, -3.686470766795223675, -28.55337830014365963 ) ) ;
#36743=CARTESIAN_POINT ( 'NONE',  ( -29.99078130865111547, 0.6403921273831606475, -7.361166318520860230 ) ) ;
#36744=CARTESIAN_POINT ( 'NONE',  ( 34.70950711422840840, -12.76021984960118338, -7.998181218355810529 ) ) ;
#36750=FACE_BOUND ( 'NONE', #33828, .T. ) ;
#36758=CARTESIAN_POINT ( 'NONE',  ( 29.70821612178828630, -22.86209932760419861, -7.558102420314961378 ) ) ;
#36759=CARTESIAN_POINT ( 'NONE',  ( 17.51810871584791940, 13.86375751818291846, -19.02218500560174874 ) ) ;
#36760=CARTESIAN_POINT ( 'NONE',  ( 7.501377273760489572, 19.07882637373012713, -29.99999999999999645 ) ) ;
#36762=CARTESIAN_POINT ( 'NONE',  ( -22.27105386152767608, 10.77722882959855966, -7.426802025917476513 ) ) ;
#36764=CARTESIAN_POINT ( 'NONE',  ( 15.59663170297798729, -26.74431364097485897, -5.944724389301430989 ) ) ;
#36766=CARTESIAN_POINT ( 'NONE',  ( 35.84808252048253507, -3.038699442442335030, -4.999999999999996447 ) ) ;
#36767=CARTESIAN_POINT ( 'NONE',  ( -11.46203485482419815, 18.45655401365020509, -23.85043275240798266 ) ) ;
#36769=CARTESIAN_POINT ( 'NONE',  ( -15.94698504394344596, -17.91589082531237764, -21.01243287115451963 ) ) ;
#36770=CARTESIAN_POINT ( 'NONE',  ( 13.02878361272089691, -26.04899829346652140, -6.894447511635101833 ) ) ;
#36774=CARTESIAN_POINT ( 'NONE',  ( -8.005635539500367770, 26.78432071055680908, -16.83492925294579123 ) ) ;
#36779=CARTESIAN_POINT ( 'NONE',  ( 21.70875678425652566, 0.7301209385331313140, -23.85431322577691304 ) ) ;
#36783=CARTESIAN_POINT ( 'NONE',  ( -30.71051382067356172, -0.01506129966919131369, -6.887934430901168525 ) ) ;
#36786=CARTESIAN_POINT ( 'NONE',  ( 33.01932729430679814, -6.854573688073132942, -10.30955742185432200 ) ) ;
#36790=CARTESIAN_POINT ( 'NONE',  ( -37.62663912510979003, -8.659558992827880886, -5.000000000000005329 ) ) ;
#36800=CARTESIAN_POINT ( 'NONE',  ( 6.623974762475253186, 33.89653518476367111, -11.11648977816992812 ) ) ;
#36805=CARTESIAN_POINT ( 'NONE',  ( 13.76863925707710301, -20.58511431638807210, -19.22791859126990488 ) ) ;
#36811=CARTESIAN_POINT ( 'NONE',  ( -15.24185242054940836, 26.37366825853258945, -7.827947956013988851 ) ) ;
#36813=CARTESIAN_POINT ( 'NONE',  ( 12.22774578270097656, -22.02461334279974636, -17.44299809173021387 ) ) ;
#36817=CARTESIAN_POINT ( 'NONE',  ( -10.27241934331446416, 20.16311048434034348, -22.50241456494288173 ) ) ;
#36819=CARTESIAN_POINT ( 'NONE',  ( -11.05369788186578539, -17.27790053512912039, -30.00000000000000711 ) ) ;
#36821=VECTOR ( 'NONE', #29335, 1000.000000000000000 ) ;
#36823=CARTESIAN_POINT ( 'NONE',  ( -25.03491786389344043, -8.622393956815280092, -18.71499684687251630 ) ) ;
#36824=CARTESIAN_POINT ( 'NONE',  ( -13.87499679755532078, -24.58662948498892220, -12.55662072122034800 ) ) ;
#36826=EDGE_LOOP ( 'NONE', ( #36117, #30848, #4770, #30148 ) ) ;
#36827=CARTESIAN_POINT ( 'NONE',  ( 21.14671899331803928, 1.666164666168168385, -25.10787130110661991 ) ) ;
#36833=CARTESIAN_POINT ( 'NONE',  ( -30.79303797620794114, -0.1002779665139238718, -6.885808881345242050 ) ) ;
#36835=CARTESIAN_POINT ( 'NONE',  ( 30.12800540966269125, -0.8552404287211460288, -10.58273019797263714 ) ) ;
#36839=CARTESIAN_POINT ( 'NONE',  ( -20.91675722910995816, 2.871490340677382402, -25.21439981239640815 ) ) ;
#36851=CARTESIAN_POINT ( 'NONE',  ( -24.85289228938016493, 7.121634862230863838, -5.479396508039022784 ) ) ;
#36855=CARTESIAN_POINT ( 'NONE',  ( 21.93136298064665723, -25.57125421755331729, -9.878379079991990608 ) ) ;
#36858=CARTESIAN_POINT ( 'NONE',  ( 11.28378745254010695, 18.60854979943831111, -23.82222365283083576 ) ) ;
#36862=CARTESIAN_POINT ( 'NONE',  ( -16.18186380107325917, 24.02863330739335623, -6.421819638462467061 ) ) ;
#36865=CARTESIAN_POINT ( 'NONE',  ( 14.85533356076911637, 25.56315567979834213, -10.18121021804152448 ) ) ;
#36866=ORIENTED_EDGE ( 'NONE', *, *, #25538, .T. ) ;
#36867=DIRECTION ( 'NONE',  ( -0.000000000000000000, -0.000000000000000000, -1.000000000000000000 ) ) ;
#36868=EDGE_LOOP ( 'NONE', ( #17768, #35675, #33527, #15324 ) ) ;
#36869=CARTESIAN_POINT ( 'NONE',  ( -10.92279190285937140, 17.50161691125836327, -28.07041777319187048 ) ) ;
#36871=CARTESIAN_POINT ( 'NONE',  ( -14.76270255855745894, -25.48967811294425800, -10.64446229900349650 ) ) ;
#36873=CARTESIAN_POINT ( 'NONE',  ( -19.19651427957619561, -10.81311144643282773, -24.21601489736221779 ) ) ;
#36874=CARTESIAN_POINT ( 'NONE',  ( -10.17830574738310823, -20.64784012530623158, -20.65330454052350007 ) ) ;
#36876=CARTESIAN_POINT ( 'NONE',  ( 13.87278661928481860, 20.14957414006898873, -17.58567953334315703 ) ) ;
#36878=CARTESIAN_POINT ( 'NONE',  ( 19.81143946857858040, 6.663503521798424423, -25.44058611693839467 ) ) ;
#36885=CARTESIAN_POINT ( 'NONE',  ( -21.39596226364862375, -0.2386576062743040183, -24.90343605780445557 ) ) ;
#36887=CARTESIAN_POINT ( 'NONE',  ( 22.74759679801531220, 0.5550921298590332231, -21.60981102281446553 ) ) ;
#36893=CARTESIAN_POINT ( 'NONE',  ( 22.40982762235196901, 2.618079236896951656, -30.00000000000000355 ) ) ;
#36901=CARTESIAN_POINT ( 'NONE',  ( 2.741814962476898820, 38.30556977738701363, -5.000000000000001776 ) ) ;
#36908=CIRCLE ( 'NONE', #19384, 57.00000000000003553 ) ;
#36909=CARTESIAN_POINT ( 'NONE',  ( 15.07870883215744762, 27.77416456386047727, -5.935715514897943024 ) ) ;
#36913=CARTESIAN_POINT ( 'NONE',  ( -15.82159548417086725, 15.31645673244926442, -21.04376448643831665 ) ) ;
#36917=CARTESIAN_POINT ( 'NONE',  ( 14.60635565259179991, -25.45748058625455457, -10.65361818253279935 ) ) ;
#36918=CARTESIAN_POINT ( 'NONE',  ( -12.40276988179543771, -16.90054568133930957, -26.59307398819964519 ) ) ;
#36920=CARTESIAN_POINT ( 'NONE',  ( 14.28350017971037111, 24.49113824962887520, -12.54891074749486712 ) ) ;
#36922=B_SPLINE_SURFACE_WITH_KNOTS ( 'NONE', 3, 3, ( 
 ( #11537, #6029, #36518, #9284, #12329, #2595, #27569, #30227, #12132, #18433, #30824, #33489, #31022, #2396, #14785, #8689, #27767, #23926, #5629, #18039, #39757, #11935, #36323, #6813, #15774, #13314, #25314, #16579, #22656, #31809, #3580, #37313, #22460, #21865 ),
 ( #25116, #28164, #34270, #340, #12724, #19415, #35061, #22067, #3381, #19616, #936, #9488, #4176, #34467, #22257, #32010, #25710, #28359, #6615, #10275, #16177, #37513, #6424, #7216, #34661, #3975, #12921, #38104, #31217, #28562, #9690, #138, #737, #12528 ),
 ( #24919, #15978, #16375, #13115, #19022, #25504, #31414, #537, #19217, #28761, #37712, #10077, #9876, #31606, #18829, #3776, #34865, #37905, #7014, #23473, #33037, #8028, #36070, #29567, #4379, #20030, #8232, #38507, #14328, #17192, #35869, #16783, #26721, #38713 ),
 ( #23065, #25907, #10891, #29771, #13519, #29169, #20435, #35263, #5186, #1336, #13720, #32631, #39107, #1747, #10682, #32831, #26110, #11090, #14126, #4987, #7624, #17398, #1953, #20638, #35469, #11293, #26525, #26319, #32426, #20234, #10478, #19827, #23673, #28962 ),
 ( #4585, #1138, #38306, #32216, #16986, #22859, #7417, #29364, #4785, #1541, #13925, #23274, #35672, #7826, #38913, #21029, #17799, #12077, #30774, #30578, #2934, #24074, #14733, #24667, #27123, #5975, #33636, #36467, #26923, #24273, #27710, #39308, #18382, #8439 ),
 ( #9036, #29966, #8636, #11882, #33438, #40102, #33237, #21420, #5578, #34021, #17991, #36865, #2737, #12278, #33827, #37061, #15323, #39901, #15128, #36667, #27517, #17597, #8837, #9231, #14932, #11488, #5384, #30379, #2544, #24467, #21616, #30173, #21224, #2146 ),
 ( #27320, #14529, #11687, #23873, #39708, #36276, #20835, #2348, #39509, #5783, #18186, #6370, #21813, #9826, #16321, #34609, #15722, #37849, #34216, #28507, #31555, #25449, #25065, #679, #6956, #13263, #18775, #19363, #3721, #3527, #31165, #37657, #27912, #37260 ),
 ( #9635, #31361, #3330, #6564, #28110, #6762, #10222, #22205, #19163, #16124, #13059, #12472, #15924, #12869, #288, #10024, #38052, #22403, #34805, #25655, #31761, #12671, #37461, #22608, #22015, #3923, #28706, #884, #34413, #6177, #28307, #487, #18578, #18971 ),
 ( #25261, #30965, #3132, #15529, #89, #9434, #24866, #4735, #7167, #39059, #20181, #10426, #7974, #35818, #13668, #32376, #28910, #13879, #17142, #32577, #20386, #22810, #23425, #38458, #35015, #14278, #10631, #31954, #1488, #4940, #38257, #23013, #19978, #19772 ),
 ( #26268, #16527, #1088, #32166, #35207, #29520, #38661, #7366, #32781, #4533, #11237, #17344, #26468, #35415, #4122, #1695, #13466, #7573, #29720, #1901, #25856, #1286, #26669, #4327, #11041, #10834, #19565, #16732, #29115, #26058, #16934, #29318, #23225, #35621 ),
 ( #7778, #14071, #38865, #39660, #39260, #17544, #34322, #17942, #28019, #36418, #9542, #14478, #11833, #23822, #21920, #24222, #6476, #15633, #36024, #30124, #30325, #14684, #18880, #11439, #194, #2298, #396, #27073, #3241, #8790, #31271, #12581, #3434, #24973 ),
 ( #39460, #18141, #28216, #36228, #37366, #11642, #23626, #24024, #15832, #21178, #8182, #20589, #32986, #5138, #5733, #33581, #2497, #30531, #29918, #14885, #2098, #20980, #26871, #8391, #8583, #33388, #20787, #33184, #5335, #27274, #17748, #5531, #36619, #31669 ),
 ( #9738, #34922, #13576, #37568, #28416, #4236, #19077, #29224, #12974, #591, #16430, #22918, #995, #22318, #16639, #25363, #35118, #38163, #32067, #3834, #7271, #25962, #19884, #37765, #38363, #10333, #10135, #9936, #4029, #34520, #3633, #34717, #32276, #22121 ),
 ( #13170, #6870, #13376, #16842, #28820, #25765, #22714, #19673, #31469, #22512, #19471, #19270, #29022, #4440, #1196, #10535, #7477, #12777, #25172, #25565, #16234, #28617, #6670, #787, #37964, #35319, #16030, #7073, #31865, #20892, #2206, #38565, #5447, #35730 ),
 ( #36129, #14592, #14388, #26981, #7881, #38768, #8493, #10949, #30030, #17453, #20288, #10738, #8085, #11546, #23123, #39367, #32485, #33091, #35524, #7688, #23933, #17250, #5244, #29824, #23334, #20697, #32686, #8292, #36329, #33294, #13982, #17855, #39165, #38970 ),
 ( #20089, #20494, #1393, #4641, #4841, #26579, #26373, #1801, #17044, #2009, #13779, #26775, #32888, #11348, #23730, #29424, #11144, #5042, #29623, #17656, #26171, #1600, #14184, #23530, #35927, #2403, #30638, #14989, #18048, #24129, #30441, #2603, #9295, #24929 ),
 ( #11943, #27183, #21873, #3199, #27376, #33694, #39765, #24725, #15588, #2999, #27973, #36731, #24334, #37324, #8895, #18641, #6039, #21285, #39568, #36929, #148, #11744, #31032, #21089, #21679, #36525, #8697, #12537, #5843, #34080, #18443, #18245, #15387, #2796 ),
 ( #15188, #6239, #27779, #9497, #34280, #6434, #30234, #12337, #40166, #9095, #37125, #14793, #21480, #33497, #27579, #5636, #39964, #12141, #24531, #33886, #30833, #34476, #10089, #6624, #15986, #34874, #22870, #12931, #15784, #746, #19627, #3390, #19032, #10286 ),
 ( #31424, #3591, #22469, #28973, #7025, #28367, #22668, #547, #948, #3985, #351, #28174, #4188, #34672, #35072, #19427, #25322, #31820, #37721, #9887, #13124, #7226, #22267, #28773, #6825, #19226, #25919, #37917, #13328, #1148, #31616, #25720, #35274, #38114 ),
 ( #12732, #3786, #16188, #28572, #32023, #13531, #25515, #16387, #16591, #38316, #10488, #18838, #25124, #31226, #37523, #9700, #22076, #8243, #32227, #39118, #38518, #2158, #17408, #19839, #11499, #32844, #23080, #20649, #33050, #26331, #4796, #1347, #26536, #29784 ),
 ( #14541, #20042, #5200, #4997, #17202, #32437, #38924, #29181, #10693, #16996, #26935, #16795, #13730, #4390, #11304, #11100, #26122, #35479, #4596, #7635, #1964, #14138, #29375, #17609, #32642, #23884, #29978, #23684, #10901, #1552, #14340, #13935, #23287, #39322 ),
 ( #38725, #36083, #35682, #7430, #23483, #7836, #20244, #29579, #1757, #35880, #8038, #20446, #26732, #30786, #9242, #9049, #21629, #2557, #33450, #3145, #5592, #24679, #12091, #14944, #5397, #2748, #6190, #17811, #37073, #27134, #27725, #24086, #30186, #36480 ),
 ( #12290, #24480, #34034, #18003, #33248, #27925, #18595, #30390, #39720, #8648, #2949, #30979, #21432, #15541, #27332, #11896, #102, #24285, #12484, #36876, #36680, #2361, #15141, #36288, #14745, #8451, #39522, #40113, #11699, #21041, #20849, #8850, #21236, #33838 ),
 ( #33647, #5796, #18198, #30591, #15336, #5986, #27532, #39913, #18394, #13276, #6972, #10037, #31569, #22416, #24878, #3735, #25668, #22217, #18789, #12683, #501, #3539, #19376, #7181, #301, #16137, #12881, #18983, #25277, #9650, #34231, #19579, #21826, #37670 ),
 ( #25078, #16338, #31177, #1101, #37474, #22028, #28521, #35029, #13073, #34427, #28720, #6577, #31775, #34820, #3937, #15937, #899, #38066, #31971, #31374, #10236, #22622, #34621, #28320, #696, #6382, #15734, #9839, #4136, #3342, #28123, #6774, #16541, #25464 ),
 ( #19175, #37864, #28923, #37273, #9447, #7987, #16947, #26683, #4952, #26484, #19993, #38272, #29532, #22825, #7588, #20400, #4749, #38878, #23028, #1707, #35830, #29734, #1300, #32794, #17156, #29331, #13683, #10848, #35221, #32180, #26071, #17358, #7382, #19785 ),
 ( #4342, #7791, #14291, #35633, #23240, #14087, #20194, #16747, #1501, #26280, #38472, #32590, #1913, #11054, #13481, #25869, #10440, #29128, #23438, #10645, #38675, #13892, #35428, #32389, #4546, #4267, #31504, #12812, #29053, #10370, #6507, #13610, #3670, #31701 ),
 ( #22747, #22547, #35151, #16062, #6704, #16671, #19112, #38199, #25598, #28451, #18913, #16266, #19710, #31304, #7305, #430, #1028, #3472, #15867, #32103, #25397, #13408, #37997, #626, #34958, #34553, #37605, #3868, #1231, #13008, #19506, #37793, #9968, #25999 ),
 ( #7108, #28650, #31898, #9575, #823, #21956, #6903, #28256, #9774, #22347, #34753, #4062, #34359, #25207, #13203, #19307, #10171, #16468, #28851, #22151, #25803, #35356, #10977, #1838, #39199, #22953, #29854, #29257, #33120, #8116, #10570, #2235, #23565, #13809 ),
 ( #26203, #20523, #11378, #4673, #35555, #5273, #7718, #26809, #14216, #17077, #7511, #4869, #8328, #19914, #23761, #1428, #2038, #32312, #4473, #36157, #14014, #14416, #26606, #20120, #11174, #23156, #38597, #32718, #20729, #32521, #32918, #29452, #1632, #17685 ),
 ( #35960, #17284, #5076, #38396, #29655, #30061, #35760, #16877, #10771, #26402, #38801, #17483, #14623, #23365, #39000, #7916, #20320, #27407, #11773, #36359, #9327, #23964, #39795, #30667, #27810, #11575, #18473, #17883, #21709, #36959, #39394, #31063, #12169, #2432 ),
 ( #5666, #24362, #20917, #5872, #9124, #24565, #40195, #14823, #15416, #30469, #27012, #6268, #2629, #8522, #33725, #37154, #30265, #15017, #11971, #24158, #36759, #27210, #27607, #3227, #2828, #18275, #21511, #39992, #33322, #8927, #15220, #39599, #33914, #18669 ),
 ( #34112, #5470, #36554, #21319, #8725, #21117, #33525, #18078, #6069, #30864, #3026, #12367, #24755, #16641, #14390, #35928, #19885, #26172, #22919, #17251, #8086, #35731, #26776, #1802, #29825, #23336, #38364, #13780, #2010, #32278, #20495, #10950, #29624, #35320 ),
 ( #23124, #7478, #32068, #5043, #19674, #35525, #26374, #23531, #7272, #14185, #13577, #17454, #32687, #35119, #39166, #7882, #10537, #32889, #22715, #1394, #20090, #29023, #1601, #4842, #20289, #4237, #4441, #11145, #38566, #1197, #25963, #10739, #16843, #29425 ),
 ( #29225, #7690, #32486, #4642, #26580, #13983, #17045, #38769, #38972, #11547, #8896, #18049, #26982, #24532, #36526, #27781, #33887, #2797, #14794, #8293, #33695, #33092, #27184, #36930, #21481, #2207, #17856, #39965, #5245, #27580, #8698, #12143, #20893, #17657 ),
 ( #15388, #5449, #33498, #3000, #9096, #39569, #30235, #6040, #27377, #39368, #30032, #18444, #5637, #15189, #24130, #30834, #14593, #39766, #23934, #11349, #11944, #23731, #36130, #20698, #2404, #30442, #11745, #36330, #8494, #33295, #21091, #2604, #14990, #30639 ),
 ( #24335, #36733, #21286, #5844, #18246, #22471, #6435, #34674, #16389, #12338, #353, #24931, #27974, #34081, #149, #12538, #19228, #34876, #15589, #7028, #19429, #34281, #37126, #3987, #18840, #22078, #31822, #748, #28175, #31227, #10091, #15989, #37325, #6240 ),
 ( #28369, #3391, #9296, #6626, #40167, #21681, #13126, #31033, #31619, #18642, #3201, #25518, #15785, #3788, #549, #9498, #12933, #21874, #12733, #34479, #28574, #25125, #9890, #37525, #9702, #24726, #19034, #6827, #31426, #3593, #16190, #25324, #37919, #37723 ),
 ( #22269, #4392, #7432, #23290, #11102, #4190, #20044, #16797, #22872, #29183, #13533, #38116, #23485, #25722, #1349, #32439, #29581, #13330, #20246, #19629, #35882, #38727, #951, #32846, #13937, #16594, #1759, #14140, #19841, #26124, #22671, #7638, #10903, #26333 ),
 ( #17204, #32230, #28775, #8040, #13733, #10288, #35481, #38927, #32025, #38520, #10695, #25921, #23082, #28975, #29378, #4999, #4598, #16998, #35684, #1554, #35074, #7838, #32644, #1150, #4799, #20449, #26538, #7228, #38319, #10490, #35276, #9051, #5594, #2750 ),
 ( #39120, #20851, #15143, #27534, #8245, #23886, #5798, #11306, #33649, #2363, #18201, #26937, #23686, #21434, #30593, #14543, #33250, #17611, #11898, #39915, #30392, #12094, #36290, #39324, #24482, #11502, #36878, #33452, #8453, #26734, #24088, #33841, #36086, #17410 ),
 ( #20651, #33052, #29786, #5400, #8852, #18005, #17813, #2560, #2160, #5202, #11701, #1966, #30188, #27334, #14747, #27137, #14343, #36482, #24287, #29981, #39524, #36683, #8650, #21238, #21044, #14946, #39722, #37275, #25466, #15543, #31571, #34429, #12883, #6192 ),
 ( #6384, #30981, #15338, #28523, #2951, #18792, #9652, #6776, #30788, #37672, #37075, #698, #15939, #18396, #10039, #31376, #21631, #19177, #3737, #24880, #3344, #40115, #25080, #28322, #3541, #16139, #34036, #34623, #9449, #5988, #37866, #21828, #27728, #12685 ),
 ( #13075, #12292, #24681, #9245, #9841, #37476, #18597, #3148, #27927, #104, #503, #22030, #12486, #22418, #31179, #34233, #25279, #15736, #28125, #303, #6579, #18985, #22219, #38880, #28925, #16749, #26486, #35635, #22827, #1104, #4751, #10647, #10238, #28722 ),
 ( #23030, #13483, #3939, #1302, #17158, #16340, #7793, #25670, #26282, #901, #13278, #20196, #10442, #38677, #35430, #31973, #7590, #19581, #22624, #29130, #23242, #4138, #4548, #25871, #16543, #1709, #13685, #29333, #29534, #38274, #1503, #11056, #13894, #14089 ),
 ( #35031, #35223, #7384, #10850, #34822, #7183, #26073, #19787, #32182, #4344, #38474, #38068, #6974, #31777, #19995, #32391, #32592, #19378, #16949, #14293, #18154, #33403, #35832, #27481, #8598, #39073, #36635, #24236, #2113, #20801, #17360, #2311, #5544, #20995 ),
 ( #11848, #26885, #23440, #2703, #39273, #20402, #30138, #33596, #26685, #11452, #8404, #8196, #23838, #11251, #24038, #39867, #39477, #14697, #17955, #36433, #29736, #33198, #27088, #36037, #11656, #15091, #30340, #8804, #30544, #7989, #32796, #36244, #20603, #23639 ),
 ( #4954, #2512, #14899, #5748, #29932, #27288, #1915, #39673, #33001, #21191, #5152, #14492, #17558, #5350, #17763, #254, #18937, #12242, #27678, #9196, #28075, #16089, #6140, #9000, #34182, #12837, #36827, #40065, #3495, #18345, #28474, #24632, #37026, #15687 ),
 ( #21582, #25230, #37628, #30934, #9399, #5942, #31132, #34382, #37423, #9796, #33984, #455, #15494, #12044, #31528, #27879, #21387, #18743, #22176, #15290, #52, #37228, #18544, #12437, #3099, #12641, #24434, #25030, #3295, #21981, #9599, #30737, #21777, #6532 ),
 ( #34576, #15892, #24831, #33794, #31325, #2900, #6334, #6726, #19135, #28278, #3691, #29282, #22370, #16901, #25825, #1451, #10192, #34776, #32544, #13836, #38019, #4089, #848, #35382, #26228, #13636, #38624, #7132, #22573, #7741, #34982, #10798, #16694, #19530 ),
 ( #31726, #29078, #13228, #23182, #1255, #35583, #32336, #13030, #31921, #35175, #16493, #20145, #16287, #4498, #28877, #17103, #1052, #19941, #26023, #4699, #649, #25421, #38423, #7538, #25620, #28673, #13431, #10596, #37818, #38225, #9990, #22773, #6925, #19331 ),
 ( #3889, #10394, #7331, #19737, #4294, #32130, #22978, #39021, #20941, #4900, #11603, #14647, #8546, #8142, #23986, #30290, #36578, #1863, #2459, #27036, #26832, #14240, #20753, #11004, #20348, #11199, #8750, #38825, #23389, #26429, #33349, #8351, #35784, #7938 ),
 ( #39418, #2257, #32742, #39223, #36184, #26631, #17709, #21140, #30084, #14846, #24183, #5693, #1657, #29877, #23590, #17307, #29681, #35986, #20549, #5491, #33547, #32942, #29480, #14038, #5100, #17508, #2061, #14437, #11402, #23784, #27234, #33144, #5297, #39620 ),
 ( #36383, #11797, #17906, #21929, #30885, #3448, #8950, #34137, #18298, #15843, #6288, #28228, #9553, #30492, #24587, #12391, #9147, #409, #33749, #34334, #36982, #34530, #21532, #37377, #3252, #12788, #6486, #25184, #18891, #204, #15643, #24779, #28030, #18104 ),
 ( #37580, #18693, #5893, #33934, #9749, #27630, #22131, #12192, #8, #2653, #31282, #6091, #18496, #15039, #31086, #30688, #11993, #27432, #37177, #39818, #3048, #24386, #21343, #12592, #2853, #36779, #24983, #15241, #40014, #15440, #27833, #9350, #21729, #29234 ),
 ( #31677, #34729, #1005, #35330, #3844, #16650, #37973, #16245, #14350, #25779, #1208, #1973, #13180, #13586, #11312, #25973, #26741, #7282, #22326, #10148, #39128, #28627, #32289, #35128, #38374, #6880, #19281, #796, #22724, #23694, #25575, #3645, #28829, #7489 ),
 ( #31479, #10546, #37773, #6681, #29032, #19089, #16040, #32078, #22521, #19895, #4450, #34931, #4037, #604, #38173, #22932, #4246, #16856, #7082, #28425, #19480, #12984, #25373, #31877, #9945, #13386, #16441, #10344, #19683, #21051, #20858, #36489, #11509, #36691 ),
 ( #33258, #36297, #33655, #2568, #23893, #9058, #33459, #12301, #18403, #27541, #39531, #33059, #18208, #17619, #11707, #21442, #5996, #26944, #2370, #24488, #29989, #12102, #5603, #36887, #5407, #2167, #27735, #33849, #36094, #8459, #17820, #39729, #30796, #24295 ),
 ( #2958, #14754, #18011, #14551, #14952, #30600, #21246, #15346, #30196, #40122, #24095, #8251, #20659, #8658, #5208, #27341, #39332, #27145, #30401, #11905, #8859, #5806, #2757, #15150, #39923, #509, #15947, #34631, #37679, #30988, #22038, #31382, #37282, #12892 ),
 ( #28132, #21638, #6783, #6199, #311, #10048, #34830, #15549, #31185, #13083, #18604, #704, #9660, #25473, #34239, #3156, #16345, #37872, #21836, #12692, #24887, #19186, #22424, #9849, #6980, #3352, #6392, #31783, #18800, #19385, #25286, #15743, #34042, #3549 ),
 ( #9456, #3946, #22226, #28727, #16146, #37084, #25087, #18993, #37484, #907, #110, #28532, #34436, #24687, #6587, #3743, #31577, #9253, #27935, #12494, #28329, #35641, #38683, #20000, #10856, #13284, #32399, #1718, #10654, #7188, #1111, #29136, #32188, #7801 ),
 ( #13488, #28930, #10448, #29338, #17368, #7389, #10244, #35437, #14095, #38073, #25878, #4757, #19588, #22629, #17164, #4144, #7996, #23247, #25678, #29741, #20201, #38280, #26492, #38886, #4349, #23036, #31979, #4554, #32598, #29540, #11062, #22832, #23446, #16756 ),
 ( #35231, #16955, #35037, #16550, #19794, #20407, #1309, #13690, #26079, #35837, #1509, #38480, #7595, #13899, #26290, #32803, #4960, #17565, #15100, #27095, #18351, #24440, #33603, #5356, #39080, #24244, #23645, #17769, #27488, #12050, #33009, #8413, #30552, #36043 ),
 ( #29937, #9006, #21394, #36249, #11257, #5949, #20807, #24048, #33801, #2709, #30146, #33205, #36835, #17961, #2118, #8204, #1921, #36439, #5755, #14705, #39874, #5157, #30349, #14499, #14300, #2518, #26690, #18160, #20609, #2317, #8606, #39484, #26890, #39280 ),
 ( #11458, #21002, #23845, #11662, #11854, #33409, #5552, #14906, #27295, #36641, #39682, #8810, #21199, #34783, #9803, #37824, #31331, #6149, #21785, #9997, #59, #16096, #18944, #37635, #30941, #18550, #27886, #6539, #6933, #24837, #27684, #12648, #31534, #15297 ),
 ( #3106, #3698, #28482, #9405, #28082, #24638, #9606, #12846, #15898, #655, #15500, #19142, #34188, #30746, #22376, #6342, #40072, #37431, #13038, #33990, #18750, #15693, #12444, #31138, #37235, #3502, #2906, #28285, #21988, #461, #25236, #37035, #260, #34388 ),
 ( #25427, #22182, #3303, #12249, #34583, #9204, #25036, #21588, #6734, #10199, #25833, #7749, #856, #35592, #4301, #20153, #28884, #13236, #11012, #32552, #16501, #22781, #19539, #13845, #4709, #32346, #17112, #38233, #1060, #26438, #13438, #29489, #35390, #10403 ),
 ( #22582, #7548, #31928, #1666, #19948, #14046, #10808, #31733, #35183, #13645, #7338, #38836, #34990, #23192, #19745, #35792, #32139, #38633, #4506, #23397, #19340, #3898, #16295, #1460, #16909, #26032, #29291, #28681, #38431, #25628, #16702, #38026, #7139, #29086 ),
 ( #4097, #1262, #10604, #22985, #26237, #8361, #32952, #17316, #30500, #4908, #20761, #11611, #8758, #32751, #39629, #39030, #2661, #17913, #20357, #12003, #24191, #33155, #36587, #17517, #1873, #39826, #21147, #5109, #11411, #8151, #2468, #33554, #20950, #5701 ),
 ( #23598, #14250, #18113, #2266, #11805, #5307, #15048, #11208, #23994, #20557, #27439, #36391, #24393, #7947, #29689, #14446, #14655, #39231, #26641, #35995, #29888, #26840, #2070, #23793, #27241, #33356, #36193, #17717, #30092, #27045, #30297, #5499, #39427, #14855 ),
 ( #8555, #3654, #37386, #12200, #27842, #16047, #6100, #22139, #24991, #3456, #36989, #24596, #33942, #12600, #613, #30894, #33757, #18702, #37591, #21351, #9156, #28238, #2861, #12992, #21541, #18504, #213, #6689, #9560, #3057, #417, #15448, #18898, #21938 ),
 ( #31290, #9758, #28434, #15, #34538, #34345, #34145, #12398, #28038, #18306, #27640, #24788, #36786, #5902, #30697, #15250, #12797, #15651, #40021, #37187, #9358, #21737, #6493, #3259, #6295, #19096, #31095, #8958, #31488, #25191, #15852, #22333, #7496, #6889 ),
 ( #10156, #13188, #19289, #25582, #37981, #4456, #25383, #4253, #13795, #22731, #31684, #22529, #1013, #4047, #19901, #7702, #806, #16656, #13394, #19489, #25786, #34939, #34737, #20105, #3855, #38181, #29038, #26188, #9953, #16863, #16252, #32502, #35338, #37781 ),
 ( #13595, #7092, #29242, #31885, #32295, #10555, #1412, #16451, #38582, #10755, #4659, #28836, #23143, #22938, #35138, #10355, #1214, #28636, #7289, #19692, #17060, #32087, #25981, #38381, #35540, #29437, #1615, #35745, #11158, #14198, #11560, #20711, #29639, #27193 ),
 ( #2221, #5650, #14607, #39583, #8710, #30453, #26387, #14404, #38985, #1818, #7899, #26594, #23548, #33307, #21100, #35943, #33509, #18061, #8099, #10962, #13998, #20508, #36144, #38785, #14806, #2024, #32906, #24141, #30046, #5058, #20304, #36538, #8313, #17866 ),
 ( #4854, #26996, #17467, #11756, #39382, #23350, #5458, #32702, #29840, #33107, #26792, #17266, #39182, #30247, #11362, #23745, #5258, #2416, #23947, #17671, #36344, #8506, #20903, #24941, #27986, #9309, #160, #37137, #31239, #39978, #12550, #33898, #12155, #9712 ),
 ( #37336, #21694, #9508, #2614, #34092, #3402, #40179, #36744, #30651, #18455, #21493, #21888, #25138, #18258, #6253, #30845, #36941, #3011, #27591, #11956, #37538, #39779, #15402, #18655, #15797, #27389, #34292, #33706, #22092, #6446, #15002, #6639, #18850, #2809 ),
 ( #15202, #28186, #363, #12744, #6054, #34490, #19046, #24346, #24547, #8911, #21300, #12350, #9108, #31048, #5856, #27793, #24738, #3212, #15602, #25335, #28385, #35288, #10301, #12944, #37735, #28586, #31634, #28987, #38129, #6838, #4407, #16398, #7654, #13746 ),
 ( #16810, #26136, #31438, #3604, #31833, #16200, #19239, #9903, #3802, #758, #10503, #38532, #13139, #10708, #23092, #25530, #561, #35494, #37931, #13341, #16000, #32243, #19439, #10101, #1363, #7239, #22481, #22284, #34685, #25733, #7446, #3998, #29194, #34888 ),
 ( #7040, #28788, #22882, #962, #22682, #35086, #19640, #19854, #32035, #4204, #16605, #1163, #13545, #25932, #38332, #14154, #23497, #20462, #13950, #35895, #1770, #7851, #26345, #4811, #4612, #29390, #38738, #8054, #17012, #1567, #32451, #38938, #32656, #10919 ),
 ( #17217, #26552, #29591, #23302, #20258, #11113, #35697, #32857, #20057, #4329, #1490, #10836, #32579, #28509, #16529, #886, #3925, #10026, #16323, #28708, #35417, #23227, #31763, #35623, #7780, #10224, #13061, #20183, #22610, #38259, #16126, #16936, #4124, #35017 ),
 ( #13265, #22405, #26270, #10428, #19980, #28912, #13881, #6958, #32168, #25657, #19365, #19567, #19774, #25451, #38663, #31956, #7575, #16734, #38054, #29117, #7169, #1090, #22813, #4535, #13468, #26060, #25858, #35209, #681, #7368, #10633, #37852, #1288, #23015 ),
 ( #34807, #13670, #38460, #32378, #29320, #14280, #30327, #33186, #11644, #4942, #20388, #1903, #20789, #8793, #39061, #1697, #26873, #5533, #29522, #32783, #36420, #11044, #21180, #17346, #29722, #8393, #14887, #5337, #26672, #8585, #11239, #27075, #30126, #36026 ),
 ( #17751, #23628, #8184, #39262, #33391, #20591, #14686, #32988, #5140, #11835, #23824, #39462, #27276, #17546, #24026, #4737, #20982, #24224, #2300, #29920, #2101, #36621, #14480, #2499, #17944, #39662, #11441, #36230, #17144, #14073, #26470, #38867, #23427, #35820 ),
 ( #7976, #18143, #25567, #24974, #28821, #3835, #5735, #38165, #19271, #9543, #7074, #34923, #12778, #31470, #28020, #12975, #16235, #31670, #19472, #21921, #22513, #37569, #33583, #13377, #9739, #31076, #592, #4030, #37367, #22122, #19078, #18882, #34522, #34323 ),
 ( #15634, #31272, #6477, #28618, #25364, #3435, #31866, #3634, #10334, #16431, #37965, #6671, #3243, #788, #195, #16031, #997, #25766, #15833, #397, #12582, #28217, #10136, #28417, #25173, #37766, #9938, #22319, #34718, #6871, #13171, #28549, #30467, #24563 ),
 ( #24361, #15016, #25491, #27406, #6267, #33913, #36758, #27209, #36958, #723, #39598, #13099, #8724, #21318, #21509, #11772, #3762, #33724, #39794, #9326, #33523, #40193, #3025, #37152, #8925, #12366, #18668, #37890, #2628, #31062, #15415, #15219, #11970, #9123 ),
 ( #10064, #21116, #5870, #2827, #18274, #30666, #5665, #18472, #22443, #6068, #30863, #27809, #24754, #24157, #27606, #21708, #39991, #34111, #34851, #16163, #17881, #30264, #2431, #14821, #12168, #36553, #18077, #924, #7204, #35050, #26309, #1736, #22644, #14114 ),
 ( #38903, #20220, #4162, #10465, #7408, #26512, #4774, #32619, #17181, #13507, #16567, #11079, #28947, #35659, #23055, #25896, #16363, #13707, #29557, #28746, #23463, #38089, #22848, #10672, #13300, #7000, #35251, #38702, #35455, #1126, #20018, #31999, #19606, #1326 ),
 ( #16974, #38294, #19813, #19402, #26097, #1528, #31797, #32205, #13915, #3962, #10876, #25696, #7612, #4365, #16773, #10264, #29156, #38496, #32415, #23265, #4572, #29352, #7817, #11677, #39891, #29956, #32820, #17788, #36659, #20424, #11279, #27311, #1939, #12069 ),
 ( #8017, #35855, #21020, #23664, #4976, #2134, #30164, #5775, #8220, #2337, #14317, #18176, #24065, #36060, #29762, #30568, #14723, #39700, #8429, #21214, #26709, #36459, #20627, #39097, #17387, #27111, #2535, #33028, #14518, #39500, #26911, #2728, #5176, #11873 ),
 ( #39299, #14922, #33429, #15119, #24262, #27508, #8828, #17979, #5570, #8625, #30369, #17584, #33624, #11476, #33225, #23862, #36266, #20825, #5373, #18963, #6752, #40093, #15712, #12464, #18571, #24856, #9222, #33818, #19156, #21412, #37252, #28101, #25254, #9026 ),
 ( #672, #24658, #12271, #279, #34600, #12664, #34012, #15916, #37053, #6556, #9627, #3519, #3124, #31350, #37649, #31548, #21607, #9819, #22007, #21805, #6170, #25056, #5966, #15315, #30956, #3712, #18371, #30766, #2927, #28300, #3322, #27701, #15521, #27904 ),
 ( #37451, #79, #34207, #31157, #9425, #34406, #16113, #476, #22196, #28499, #24457, #36855, #6360, #18768, #12860, #6948, #13254, #875, #32367, #7768, #28697, #20170, #32567, #7157, #10016, #10213, #29105, #17132, #19556, #22395, #35199, #13867, #37840, #25647 ),
 ( #3914, #4725, #23003, #25441, #29507, #38449, #38044, #26256, #38652, #31946, #10418, #19355, #32158, #35407, #10622, #10825, #22598, #1480, #16519, #13051, #34798, #28902, #31752, #19761, #23213, #16313, #1080, #38249, #35007, #13455, #4113, #13661, #25848, #1278 ),
 ( #7565, #4318, #22800, #35609, #7357, #16722, #26050, #4525, #19966, #16925, #29309, #23416, #5127, #27259, #11821, #32769, #8172, #30315, #35808, #17932, #26859, #2485, #11225, #7963, #33570, #14874, #39049, #17534, #2087, #21167, #39648, #24210, #36607, #20576 ),
 ( #23616, #8774, #17736, #32972, #11030, #8379, #5720, #20376, #18130, #4928, #29908, #5324, #17333, #1684, #14467, #33375, #30113, #36012, #14674, #26658, #29707, #36214, #14061, #39248, #11629, #11429, #23812, #26455, #20777, #36408, #38854, #33174, #8571, #1890 ),
 ( #2284, #14268, #27063, #39448, #24012, #20969, #5518, #5921, #21755, #18521, #18321, #37610, #9776, #24612, #27456, #34557, #37005, #12417, #434, #2878, #37206, #36805, #12816, #6315, #30716, #24411, #25209, #24808, #34362, #3077, #15869, #21366, #18721, #15269 ),
 ( #33959, #34163, #39844, #28258, #6117, #21960, #31111, #27658, #3275, #40042, #12221, #9376, #18918, #9175, #233, #21561, #30914, #22156, #15668, #25007, #6707, #15467, #37404, #30519, #9578, #2679, #28054, #27859, #30, #15067, #12619, #12020, #6510, #31306 ),
 ( #3475, #8976, #33772, #28454, #1433, #16066, #31903, #22752, #19922, #3674, #10577, #9972, #13815, #29060, #31507, #23163, #4273, #34756, #32318, #4479, #38000, #16473, #13013, #38204, #1236, #16678, #16883, #6907, #7516, #22551, #19115, #38602, #34961, #630 ),
 ( #28656, #26210, #25402, #37799, #22350, #22959, #10376, #19311, #31704, #16269, #3872, #13616, #25809, #828, #29262, #4070, #35562, #10778, #35363, #7112, #13208, #26004, #25601, #19510, #10176, #28857, #1033, #13415, #35157, #7312, #19719, #32108, #38401, #17289 ),
 ( #1637, #4679, #11582, #26816, #29458, #14019, #4875, #7921, #5279, #14422, #23371, #20924, #32925, #24167, #30272, #39401, #11181, #17084, #30069, #26411, #23572, #33331, #17890, #38807, #14220, #36365, #10983, #23970, #5082, #8530, #29662, #35766, #39605, #5476 ),
 ( #29859, #2440, #20327, #39206, #32724, #14830, #23766, #1846, #26612, #27216, #2044, #11779, #20528, #7723, #39005, #36165, #35966, #8121, #17490, #11383, #14630, #20127, #8335, #20735, #33128, #32526, #17693, #2243, #27018, #12768, #27612, #15624, #21715, #6467 ),
 ( #24964, #18676, #34117, #3031, #6274, #36561, #15423, #37358, #33919, #30475, #24367, #12176, #15226, #31068, #18872, #11977, #27816, #24571, #30673, #36965, #21325, #5675, #31264, #33532, #9129, #25555, #9533, #21123, #28010, #27414, #3426, #3232, #8733, #388 ),
 ( #5877, #183, #36764, #12572, #21910, #34314, #39997, #15822, #28209, #18085, #8935, #2635, #15023, #6075, #33730, #12373, #39803, #18280, #18479, #2835, #21516, #30870, #24760, #37159, #9334, #584, #16631, #3826, #1386, #16226, #4229, #10325, #35311, #29012 ),
 ( #4021, #19665, #7470, #31661, #32059, #29216, #1187, #32266, #25757, #12966, #28609, #4431, #34710, #10526, #13369, #13568, #25355, #37757, #22310, #987, #25163, #19261, #22112, #7065, #25955, #9731, #9928, #38354, #31460, #37561, #6861, #780, #28812, #19877 ),
 ( #22909, #16835, #13162, #22503, #19070, #16422, #7263, #22706, #34512, #25556, #6662, #37957, #3626, #16021, #10128, #28408, #31858, #34913, #19462, #38153, #35109, #38759, #14175, #29415, #14380, #17846, #29817, #5033, #23723, #26767, #20081, #11136, #20486, #26366 ),
 ( #5236, #17242, #10731, #36121, #35515, #29615, #39360, #23924, #4633, #20279, #2197, #7678, #30020, #38962, #14583, #23326, #32478, #5438, #26973, #10940, #1792, #26572, #33287, #11536, #36322, #8486, #32679, #35722, #20885, #7874, #30226, #2002, #4833, #23116 ),
 ( #39157, #13975, #17035, #1591, #23522, #13770, #35918, #26162, #11338, #20689, #8077, #32880, #17444, #8282, #38557, #33084, #17649, #24517, #3186, #27173, #18037, #34068, #8688, #18827, #2594, #30432, #6026, #12526, #30822, #11933, #6229, #14980, #24714, #27765 ),
 ( #37115, #40154, #15576, #27367, #31020, #5834, #2394, #21863, #18234, #39559, #9084, #24917, #5628, #30627, #27567, #39755, #2785, #24323, #2989, #6422, #18431, #33875, #12327, #15375, #21079, #39954, #21470, #36721, #9282, #34268, #21666, #27963, #37310, #14784 ),
 ( #135, #9486, #33488, #8885, #11736, #24121, #18631, #12130, #36517, #21273, #33683, #15177, #36917, #28356, #34659, #31604, #10475, #28960, #4174, #16577, #37710, #535, #38304, #12919, #19614, #7012, #9874, #338, #37903, #1136, #12721, #13516, #22065, #6810 ),
 ( #22255, #25502, #19215, #25905, #6613, #22654, #3773, #7415, #16175, #10273, #16373, #22857, #35058, #35261, #32008, #13312, #28759, #10075, #934, #31215, #22457, #3379, #28560, #15771, #25312, #735, #13113, #28162, #25114, #37511, #9688, #34863, #19412, #34465 ),
 ( #31807, #7214, #3973, #19020, #31411, #25708, #3578, #15976, #38101, #1745, #27271, #32214, #26317, #14124, #10889, #2688, #35467, #11831, #38711, #36813, #23272, #39658, #4985, #30529, #24220, #15077, #8787, #1951, #17396, #26523, #29769, #19825, #38911, #21176 ),
 ( #7622, #35670, #39853, #29362, #5731, #8026, #36617, #20028, #32424, #16984, #35866, #24419, #13923, #16781, #11088, #33579, #4377, #4582, #18139, #26107, #29166, #1538, #7824, #23471, #27466, #20433, #20231, #12030, #32629, #14326, #1334, #13718, #4783, #38505 ),
 ( #17190, #10680, #29565, #23063, #32829, #12424, #5928, #15674, #19122, #12229, #24817, #34169, #33969, #9383, #24620, #9584, #13019, #25016, #241, #18924, #21969, #15278, #6320, #28062, #21569, #37411, #637, #34369, #34564, #3679, #25408, #21374, #21765, #6126 ),
 ( #15477, #37617, #30725, #25217, #18729, #9783, #18530, #2886, #8985, #6517, #12626, #31313, #3482, #27665, #31118, #15878, #30921, #28265, #33780, #441, #6714, #16073, #18329, #40049, #3282, #3084, #37013, #9183, #27867, #38, #12822, #28462, #37214, #22162 ),
 ( #31517, #10787, #34969, #1041, #38214, #17091, #35568, #23170, #7730, #4077, #7120, #4687, #19519, #26217, #13625, #16480, #6915, #4281, #20134, #19317, #32533, #28662, #13421, #1244, #31713, #29466, #25815, #29271, #26011, #31909, #10584, #22560, #25608, #32116 ),
 ( #22966, #1644, #1439, #14026, #38609, #19929, #35369, #16684, #7525, #37806, #29066, #9979, #35163, #3879, #38009, #10382, #28864, #32324, #22357, #13215, #38408, #22760, #7319, #19726, #4487, #16276, #34765, #835, #16890, #13822, #10182, #10991, #17895, #17297 ),
 ( #38813, #30481, #11588, #1851, #39610, #27224, #5087, #23773, #20337, #5285, #8536, #23976, #11785, #14227, #14835, #29865, #26419, #5682, #2050, #23378, #33134, #36567, #29669, #14427, #11391, #11186, #26822, #26618, #27026, #2642, #39010, #23578, #30074, #8739 ),
 ( #24172, #21128, #17497, #36173, #32730, #17697, #20929, #36371, #33538, #35975, #18093, #39212, #35773, #7927, #8340, #4884, #2247, #8128, #20536, #20741, #14634, #32932, #39408, #33338, #5481, #30278, #2450, #6280, #24972, #28018, #21330, #12380, #21721, #27617 ),
 ( #6475, #18484, #11982, #37365, #36770, #30876, #395, #25171, #5883, #21523, #3433, #8941, #31270, #40199, #15831, #24576, #33739, #6669, #28215, #12183, #3039, #15432, #34519, #12776, #37567, #9737, #33926, #36971, #22120, #9138, #19076, #31075, #6081, #24374 ),
 ( #18287, #31468, #30678, #27822, #18684, #2841, #15029, #24771, #18879, #3240, #37166, #193, #40005, #15231, #9341, #27419, #34123, #9541, #15632, #12580, #39808, #21919, #34321, #26170, #10134, #38362, #7687, #22917, #10737, #4235, #19269, #34921, #23122, #13169 ),
 ( #31668, #35117, #31864, #37963, #4028, #28616, #12973, #38564, #590, #16429, #7270, #4439, #28415, #35318, #34716, #35523, #7476, #6869, #20088, #13575, #16029, #3632, #29021, #3833, #16841, #29223, #22511, #994, #37764, #22713, #25961, #1195, #1392, #16233 ),
 ( #10534, #13375, #786, #19672, #25362, #25564, #7072, #9935, #22317, #19470, #28819, #19883, #32066, #25764, #38162, #10332, #16638, #32275, #13778, #7880, #5446, #17452, #8696, #14792, #23932, #35926, #29423, #14591, #13981, #8084, #17854, #2402, #23333, #38969 ),
 ( #11545, #27182, #20287, #39567, #11743, #26578, #1599, #36524, #11143, #14387, #24128, #4840, #39164, #38767, #32484, #8291, #32685, #26372, #4640, #26774, #36328, #5041, #30233, #35729, #20696, #17249, #29622, #10948, #11347, #39366, #17043, #23529, #23729, #20493 ),
 ( #8492, #32887, #1800, #29823, #20891, #17655, #14183, #33293, #2008, #36128, #26980, #30029, #33090, #2205, #5243, #40165, #9496, #18442, #14988, #8894, #36928, #39963, #15587, #3389, #36730, #12336, #9094, #15187, #21479, #5842, #30440, #15783, #18047, #33885 ),
 ( #21284, #21872, #5635, #33693, #12536, #27375, #37522, #18244, #30637, #24724, #31225, #9294, #2795, #24928, #27578, #3198, #6238, #147, #12140, #27972, #34279, #28173, #24530, #6433, #18640, #30832, #6038, #37124, #2602, #11942, #2998, #350, #39764, #24333 ),
 ( #15386, #21678, #25123, #34079, #31031, #37323, #18837, #27778, #12731, #21088, #33496, #38113, #1346, #10285, #35273, #4389, #26121, #22075, #10088, #34671, #37720, #3590, #9886, #22266, #28972, #16794, #25321, #29180, #13729, #3785, #6623, #9699, #16187, #31819 ),
 ( #7429, #22869, #19838, #28571, #6824, #34475, #19225, #38315, #25719, #745, #19031, #16386, #32226, #31423, #15985, #546, #13123, #13327, #28366, #12930, #25514, #1147, #22667, #31615, #35071, #37916, #22468, #3984, #10487, #34873, #19626, #7024, #19426, #28772 ),
 ( #7225, #947, #32022, #4187, #16590, #13530, #25918, #32436, #26330, #14137, #17201, #33048, #20847, #13934, #29783, #26535, #32641, #38923, #23286, #7634, #33246, #35478, #11099, #26731, #5198, #38724, #10900, #35681, #14339, #2359, #4795, #20041, #20445, #39320 ),
 ( #23079, #29976, #29374, #5395, #8241, #10692, #14743, #23683, #7835, #11497, #23882, #29578, #35879, #4595, #17407, #20647, #36081, #36287, #20243, #26933, #1756, #38517, #17809, #23482, #16995, #4996, #8449, #1551, #8037, #32843, #1963, #39117, #11303, #17607 ),
 ( #2156, #14539, #30184, #33448, #24478, #33836, #39718, #15334, #18787, #27723, #12482, #21824, #3340, #39520, #27530, #11894, #14942, #21039, #27330, #24283, #6188, #34229, #2555, #6380, #31175, #21234, #24084, #27132, #33645, #9047, #37271, #36678, #5984, #5590 ),
 ( #8848, #18001, #9445, #21430, #30977, #39911, #24876, #30388, #2947, #5794, #18196, #36478, #18392, #34032, #11697, #30589, #30784, #2746, #8646, #15139, #18593, #12089, #36874, #40111, #3143, #12288, #24677, #15539, #37071, #27923, #9240, #21627, #100, #897 ),
 ( #35027, #22823, #16336, #31372, #6772, #35219, #25275, #1099, #28921, #12879, #19173, #16135, #7380, #13479, #25867, #38270, #22215, #37668, #19783, #9837, #4134, #31773, #34619, #25076, #22414, #10438, #37472, #32178, #6575, #31567, #19374, #9648, #15732, #3733 ),
 ( #28121, #3537, #7179, #28519, #299, #694, #19577, #13274, #12681, #31969, #22026, #16539, #38064, #25666, #34818, #10234, #34425, #6970, #18981, #13071, #15935, #28318, #25462, #37862, #22620, #499, #10035, #3935, #28718, #38673, #4747, #29329, #13681, #26882 ),
 ( #5149, #29126, #19991, #36034, #10643, #20798, #4544, #32387, #7985, #14489, #32792, #13890, #8193, #16945, #26681, #29732, #23637, #23238, #39069, #17555, #11449, #1499, #29929, #1911, #1705, #26278, #35828, #26069, #35426, #10846, #23835, #38470, #23026, #1298 ),
 ( #4950, #8401, #20398, #17356, #14289, #11248, #7586, #14085, #11052, #35631, #20600, #36241, #32998, #2109, #39270, #4340, #16745, #17154, #7789, #20192, #32588, #29530, #26482, #38876, #23436, #8594, #49, #12434, #27285, #33981, #24827, #5541, #6137, #30734 ),
 ( #36632, #30135, #39864, #3096, #36430, #8801, #18151, #17952, #33593, #20992, #33791, #37225, #8997, #24431, #2897, #5939, #39474, #30541, #12041, #30337, #21384, #9396, #18341, #18541, #27876, #33195, #5346, #5745, #2509, #33400, #27085, #14896, #39670, #12239 ),
 ( #21579, #11844, #11653, #17760, #30931, #24233, #21188, #2700, #2308, #15491, #14694, #24035, #15087, #27478, #36824, #15287, #27675, #40062, #24629, #37023, #9193, #1401, #18740, #13786, #251, #15889, #31525, #31129, #29231, #28275, #35327, #3688, #21978, #28471 ),
 ( #34572, #32285, #34379, #25418, #3492, #6529, #38574, #6723, #10543, #26178, #31322, #38370, #23132, #7486, #10745, #646, #12638, #452, #35531, #18934, #16851, #16086, #22928, #25027, #37420, #12834, #13027, #21774, #25227, #3292, #19132, #4447, #15684, #9596 ),
 ( #37625, #34179, #19891, #28072, #6331, #9793, #22173, #40161, #21674, #6619, #18637, #15982, #15583, #31419, #34075, #24721, #31221, #25317, #6235, #19026, #27969, #31026, #3781, #15778, #3585, #19222, #3193, #28363, #742, #541, #16184, #37517, #12333, #143 ),
 ( #22262, #25120, #12927, #37121, #9289, #12532, #12728, #13120, #24925, #33882, #18833, #37717, #21476, #37318, #9881, #2995, #36925, #9493, #21869, #345, #6819, #9696, #34274, #6430, #3385, #34667, #28169, #31612, #22071, #28567, #9091, #6033, #34471, #18438 ),
 ( #30828, #15383, #27771, #32222, #35678, #28767, #28968, #10484, #10281, #25915, #943, #26117, #29573, #1342, #16789, #35475, #38513, #31815, #22865, #4385, #38110, #13726, #17198, #10688, #10897, #20240, #1753, #37911, #38312, #22664, #13321, #19423, #25716, #35067 ),
 ( #35269, #13930, #7222, #3981, #25509, #38720, #19622, #1144, #7424, #4791, #23280, #7832, #32637, #32016, #4183, #10083, #16586, #26325, #23073, #13525, #34870, #29177, #22465, #7020, #16381, #19833, #7630, #20036, #32433, #4591, #16992, #29370, #1547, #29778 ),
 ( #23679, #21230, #23479, #8034, #11096, #17997, #33243, #35875, #20441, #11299, #14334, #11694, #20842, #1960, #27326, #39315, #30585, #36673, #5585, #17603, #32838, #36474, #4993, #29972, #39715, #24279, #17404, #20644, #2550, #26728, #30385, #11494, #14939, #36077 ),
 ( #39113, #18193, #8238, #36282, #8844, #33043, #5390, #5194, #33642, #30180, #2152, #14535, #5789, #8446, #11889, #26929, #14133, #23879, #2355, #17805, #26531, #14739, #38919, #27129, #39515, #24080, #8642, #21035, #33444, #18388, #34420, #21622, #19169, #34027 ),
 ( #12875, #6570, #25269, #31367, #25071, #28116, #9440, #295, #2743, #21819, #3533, #95, #36871, #30780, #18587, #6183, #37467, #37664, #2942, #34224, #30972, #37067, #3138, #27718, #12084, #9832, #39907, #15535, #6376, #15931, #27525, #18977, #33833, #22211 ),
 ( #18781, #34615, #31171, #12284, #5981, #40108, #12677, #24674, #22021, #27919, #9643, #28313, #6768, #15330, #494, #15135, #12478, #9237, #3336, #24474, #9042, #21427, #24872, #37266, #15728, #7374, #28713, #4334, #16330, #19370, #25863, #19986, #891, #1293 ),
 ( #1494, #32383, #13677, #16740, #38265, #29122, #31562, #10434, #4539, #28917, #25456, #31768, #7175, #10229, #26065, #13885, #6965, #22818, #19572, #25662, #31963, #13270, #689, #26274, #28514, #4129, #35214, #16941, #16131, #23021, #22410, #38668, #38465, #3728 ),
 ( #19779, #38059, #34812, #22616, #10638, #35022, #35422, #16534, #7580, #29325, #10840, #3931, #23232, #35627, #1095, #13474, #32173, #13066, #7784, #37857, #10031, #29526, #14078, #17148, #24030, #39266, #1701, #26476, #17350, #20393, #17755, #26877, #35824, #33395 ),
 ( #8397, #11839, #20793, #5537, #14891, #36625, #32583, #20595, #4946, #7980, #38871, #32787, #29727, #39468, #27280, #1907, #39666, #24228, #14284, #11048, #20188, #26677, #2105, #30331, #39065, #11445, #23432, #2504, #36235, #11243, #23632, #4742, #14484, #36425 ),
 ( #36030, #33191, #8188, #32993, #23828, #5144, #17550, #29924, #14690, #5341, #30130, #2304, #27079, #11648, #8589, #20986, #17948, #31318, #5740, #21574, #12430, #9590, #33587, #246, #39859, #3487, #18735, #21184, #12828, #34175, #24427, #21974, #37219, #36819 ),
 ( #28067, #27670, #3288, #34374, #15884, #21380, #6525, #6325, #6131, #33786, #44, #30536, #12036, #18335, #28270, #18147, #2695, #15083, #12632, #27872, #27472, #8992, #5934, #30730, #31125, #15486, #2891, #18930, #33975, #25224, #447, #25022, #12234, #15283 ),
 ( #24625, #8797, #40056, #37019, #9189, #37416, #18536, #30926, #3089, #24822, #9390, #21770, #15680, #10589, #34771, #841, #38014, #16895, #35375, #22972, #7532, #3884, #6920, #4493, #19323, #26017, #13426, #16282, #6719, #4082, #19936, #19128, #32329, #22363 ) ),
 .UNSPECIFIED., .F., .F., .F.,
 ( 4, 3, 3, 3, 3, 3, 3, 3, 3, 3, 3, 3, 3, 3, 3, 3, 3, 3, 3, 3, 3, 3, 3, 3, 3, 3, 3, 3, 3, 3, 3, 3, 3, 3, 3, 3, 3, 3, 3, 3, 3, 3, 3, 3, 3, 3, 3, 3, 3, 3, 3, 4 ),
 ( 4, 3, 3, 3, 3, 3, 3, 3, 3, 3, 3, 4 ),
 ( -4.440892098500626162E-16, 0.0001220703125634871116, 0.0002441406251274183124, 0.0004882812502552807141, 0.0009765625005110055174, 0.001953125001022455124, 0.003906250002045354337, 0.007812500004091152764, 0.01562500000818274962, 0.03125000001636594332, 0.04687500002454914050, 0.06250000003273233073, 0.07812500004091552097, 0.09375000004909872509, 0.1093750000572819153, 0.1250000000654651056, 0.1406250000736483097, 0.1416015625741597617, 0.1420898438244154738, 0.1425781250746712137, 0.1445312500756941176, 0.1484375000777398979, 0.1562500000818314860, 0.1718750000900146901, 0.1875000000981978943, 0.2031250001063810706, 0.2187500001145642747, 0.2343750001227474788, 0.2500000001309306552, 0.2656250001391138316, 0.2812500001472970634, 0.2968750001554802398, 0.3125000001636634162, 0.3281250001718466480, 0.3320312501738924560, 0.3330078126744039357, 0.3332519532995317779, 0.3334960939246596201, 0.3339843751749153600, 0.3359375001759382640, 0.3437500001800298244, 0.3750000001963962326, 0.4062500002127625853, 0.4375000002291289936, 0.4687500002454954018, 0.4726562502475412098, 0.4746093752485641137, 0.4750976564988198536, 0.4755859377490755380, 0.4765625002495870177, 0.4843750002536785781, 0.5000000002618617545 ),
 ( 0.000000000000000000, 0.06250000000000004163, 0.1250000000000000833, 0.1875000000000001110, 0.2500000000000001665, 0.3750000000000002220, 0.5000000000000003331, 0.6250000000000004441, 0.7500000000000004441, 0.8750000000000005551, 0.9375000000000006661, 1.000000000000000666 ),
 .UNSPECIFIED. ) ;
#36925=CARTESIAN_POINT ( 'NONE',  ( -13.30932211733667714, -23.61699183225733734, -14.47971286837055516 ) ) ;
#36927=CARTESIAN_POINT ( 'NONE',  ( -28.82765927138905582, -24.00093021346537370, -6.713486956739352252 ) ) ;
#36928=CARTESIAN_POINT ( 'NONE',  ( 1.466865423182375894, -22.17185249639828371, -19.06817386734656239 ) ) ;
#36929=CARTESIAN_POINT ( 'NONE',  ( 13.16433369016599642, 21.27373372467787505, -17.47625806870802379 ) ) ;
#36930=CARTESIAN_POINT ( 'NONE',  ( 18.28086812270377948, 11.17358269430334339, -22.25045871718272394 ) ) ;
#36932=CARTESIAN_POINT ( 'NONE',  ( -5.098808368553501502, 35.72236394901918999, -9.747318335016483815 ) ) ;
#36934=CARTESIAN_POINT ( 'NONE',  ( -24.31092352897995923, -3.750127306134790395, -20.04326310685654278 ) ) ;
#36937=ORIENTED_EDGE ( 'NONE', *, *, #30354, .T. ) ;
#36940=CARTESIAN_POINT ( 'NONE',  ( -26.25002775687122991, 0.6713331420556990503, -15.48113191161911040 ) ) ;
#36941=CARTESIAN_POINT ( 'NONE',  ( 29.97182693708377244, -10.99419485510059857, -13.85563110560112676 ) ) ;
#36954=CARTESIAN_POINT ( 'NONE',  ( -2.597202671505355998, 23.56478163197531472, -21.87304641510805325 ) ) ;
#36956=DIRECTION ( 'NONE',  ( 0.000000000000000000, 0.000000000000000000, 1.000000000000000000 ) ) ;
#36958=CARTESIAN_POINT ( 'NONE',  ( 29.35710168727448277, -22.60462445154060163, -8.421042284273656975 ) ) ;
#36959=CARTESIAN_POINT ( 'NONE',  ( 15.82973276131441409, 13.18043781167240525, -27.70532646144207689 ) ) ;
#36960=CARTESIAN_POINT ( 'NONE',  ( 12.74815967810739714, 30.65541959961472074, -9.036990827636632417 ) ) ;
#36963=CARTESIAN_POINT ( 'NONE',  ( -18.35172899305704064, 9.167379654309337766, -29.42880166646513018 ) ) ;
#36965=CARTESIAN_POINT ( 'NONE',  ( 12.43149986465983581, -22.02020054580998476, -17.42080020519824757 ) ) ;
#36967=CARTESIAN_POINT ( 'NONE',  ( -11.41987377193683528, -19.41918266173334828, -20.90349153980999475 ) ) ;
#36968=CARTESIAN_POINT ( 'NONE',  ( -15.00814140074610137, 26.00168467618496848, -9.236653823862166490 ) ) ;
#36969=CIRCLE ( 'NONE', #18161, 16.00000000000000000 ) ;
#36970=CARTESIAN_POINT ( 'NONE',  ( -13.64791795088057569, -15.39248673868869943, -28.54146132201631758 ) ) ;
#36971=CARTESIAN_POINT ( 'NONE',  ( 8.501265317358036810, -19.09793930249271199, -26.33487222037532760 ) ) ;
#36973=ORIENTED_EDGE ( 'NONE', *, *, #36169, .F. ) ;
#36975=CARTESIAN_POINT ( 'NONE',  ( -7.311911706866655258, 22.04011237685605806, -22.15126999930638974 ) ) ;
#36982=CARTESIAN_POINT ( 'NONE',  ( 24.54342919967269054, 0.4649732435212016179, -18.45589562361645619 ) ) ;
#36986=CARTESIAN_POINT ( 'NONE',  ( -29.32665613511613500, 0.1060819663625076903, -10.65436168154521646 ) ) ;
#36989=CARTESIAN_POINT ( 'NONE',  ( 33.33462692813205308, -5.949911538848129844, -9.434312102335114858 ) ) ;
#36994=ADVANCED_FACE ( 'NONE', ( #27331 ), #30185, .T. ) ;
#37003=CARTESIAN_POINT ( 'NONE',  ( 6.978616903035645080, 30.76321682976233163, -13.89331903619694231 ) ) ;
#37005=CARTESIAN_POINT ( 'NONE',  ( 16.05151241257415506, -23.71462521554112257, -14.24666968269734291 ) ) ;
#37010=CARTESIAN_POINT ( 'NONE',  ( -15.41384351598270719, 26.69841823979104589, -5.946086308406814069 ) ) ;
#37013=CARTESIAN_POINT ( 'NONE',  ( 9.808896528483906252, -18.87720056256629775, -25.03243745114713903 ) ) ;
#37017=CARTESIAN_POINT ( 'NONE',  ( -13.86191765000858034, 30.49075772208747992, -5.458815180633147968 ) ) ;
#37019=CARTESIAN_POINT ( 'NONE',  ( -20.49308938538982616, -27.11270024657357425, -6.352872741783973431 ) ) ;
#37020=CARTESIAN_POINT ( 'NONE',  ( 15.29245034862073283, 32.56469986092002955, -4.999999999999995559 ) ) ;
#37022=CARTESIAN_POINT ( 'NONE',  ( -20.10573352757293009, -5.610599920320681555, -27.07607080465070837 ) ) ;
#37023=CARTESIAN_POINT ( 'NONE',  ( -12.13390174137889943, -22.02765613461586369, -17.45112777453272557 ) ) ;
#37026=CARTESIAN_POINT ( 'NONE',  ( 20.43785338154470921, 1.730618592969307867, -29.36392387493818035 ) ) ;
#37033=CARTESIAN_POINT ( 'NONE',  ( -25.22586935555838394, 0.3525131807024055042, -17.43529033463691746 ) ) ;
#37035=CARTESIAN_POINT ( 'NONE',  ( 20.54762595280696047, -0.6097413519664565129, -28.65496405823322590 ) ) ;
#37039=CARTESIAN_POINT ( 'NONE',  ( -20.40386927488033919, 2.900997764857453198, -28.16784849636700372 ) ) ;
#37049=CARTESIAN_POINT ( 'NONE',  ( -23.58215323251389250, 7.916431794952161205, -10.35477734161397123 ) ) ;
#37053=CARTESIAN_POINT ( 'NONE',  ( 23.53567760670948772, -25.90459182271207794, -8.508653576017058739 ) ) ;
#37056=CARTESIAN_POINT ( 'NONE',  ( 15.09835175993660172, 26.53469318400227905, -8.288073639389835989 ) ) ;
#37058=CARTESIAN_POINT ( 'NONE',  ( -12.29080222946883794, 16.45214217256524236, -28.75623754596550441 ) ) ;
#37061=CARTESIAN_POINT ( 'NONE',  ( 14.04351365870728685, 23.90287290350755711, -13.51466990167370064 ) ) ;
#37065=CARTESIAN_POINT ( 'NONE',  ( -14.83272754704879581, 26.11747447809059253, -9.691566001703526112 ) ) ;
#37067=CARTESIAN_POINT ( 'NONE',  ( -11.65106285942700559, -20.96414419292345599, -19.48341064667247124 ) ) ;
#37070=CARTESIAN_POINT ( 'NONE',  ( -34.68504811378230812, -15.55931908636949856, -6.702081268225836830 ) ) ;
#37071=CARTESIAN_POINT ( 'NONE',  ( -8.882954391321824517, -18.80275190887125092, -26.89438617859911318 ) ) ;
#37073=CARTESIAN_POINT ( 'NONE',  ( 11.95648576969578514, 17.00773961595601946, -26.90402825398920683 ) ) ;
#37075=CARTESIAN_POINT ( 'NONE',  ( 25.36334589218571622, 5.533731653267201622, -9.821327216179092545 ) ) ;
#37080=CARTESIAN_POINT ( 'NONE',  ( -20.57926082878400820, -27.21289976832866842, -5.911089126657673276 ) ) ;
#37082=CARTESIAN_POINT ( 'NONE',  ( -29.50951042545606740, -0.6464191806711061528, -11.53192585844440288 ) ) ;
#37083=ADVANCED_FACE ( 'NONE', ( #34033 ), #36679, .F. ) ;
#37084=CARTESIAN_POINT ( 'NONE',  ( 30.94917753044411057, -0.3725058681004523864, -7.345268830895530954 ) ) ;
#37091=CARTESIAN_POINT ( 'NONE',  ( 37.49625565938770677, -14.69322820095493221, -4.999999999999991118 ) ) ;
#37094=CARTESIAN_POINT ( 'NONE',  ( -14.98890122036483419, -28.67928442680469203, -4.999999999999999112 ) ) ;
#37099=CARTESIAN_POINT ( 'NONE',  ( 2.591799644895701693, 25.51815422415490531, -19.65972820106781072 ) ) ;
#37108=CARTESIAN_POINT ( 'NONE',  ( 10.49180330207988554, 18.23678832236204883, -26.15052258653890149 ) ) ;
#37111=CARTESIAN_POINT ( 'NONE',  ( -16.84514298104724617, 16.73865939197028396, -15.83090985262360739 ) ) ;
#37115=CARTESIAN_POINT ( 'NONE',  ( 15.48852768438595362, -26.74270545139661337, -5.000000000000000888 ) ) ;
#37116=CARTESIAN_POINT ( 'NONE',  ( -12.29725303649800594, -16.76881851035475890, -27.24954791347179395 ) ) ;
#37118=CARTESIAN_POINT ( 'NONE',  ( 12.92139572017179461, 21.66467470877940826, -17.43601754788530656 ) ) ;
#37121=CARTESIAN_POINT ( 'NONE',  ( -15.33721547441370170, -26.62960585016953985, -6.417084653855770426 ) ) ;
#37123=CARTESIAN_POINT ( 'NONE',  ( -25.99964108865075829, -21.70810690337949111, -12.01446658603936868 ) ) ;
#37124=CARTESIAN_POINT ( 'NONE',  ( -0.2709479841607694284, -20.69534288464836180, -26.62127205292360443 ) ) ;
#37125=CARTESIAN_POINT ( 'NONE',  ( 15.16228493941223476, 25.10766862421788659, -9.719789186029419881 ) ) ;
#37126=CARTESIAN_POINT ( 'NONE',  ( 19.31451997534437837, 9.825694766287540460, -21.17302188312822508 ) ) ;
#37128=CARTESIAN_POINT ( 'NONE',  ( -3.578418739405598181, 25.33586860667721297, -19.68557914504843964 ) ) ;
#37130=CARTESIAN_POINT ( 'NONE',  ( -27.98118135240622095, -5.186583525525977123, -15.94789710196255150 ) ) ;
#37134=CARTESIAN_POINT ( 'NONE',  ( -19.48557158514985588, -11.25000000000002309, 3.000000000000000000 ) ) ;
#37136=CARTESIAN_POINT ( 'NONE',  ( -29.78651012600981218, 0.8611516314391640670, -7.362443450658839872 ) ) ;
#37137=CARTESIAN_POINT ( 'NONE',  ( 20.25988315325368205, -6.799842207391387561, -25.67160698062978952 ) ) ;
#37140=DIRECTION ( 'NONE',  ( 0.000000000000000000, 0.000000000000000000, -1.000000000000000000 ) ) ;
#37147=CARTESIAN_POINT ( 'NONE',  ( -2.236895112781582817, 20.38702974553298830, -29.21783655675459102 ) ) ;
#37152=CARTESIAN_POINT ( 'NONE',  ( 19.49879619062026137, -14.97211638113389398, -20.74291969904744803 ) ) ;
#37154=CARTESIAN_POINT ( 'NONE',  ( 18.53780643774816994, 14.90836240266203738, -13.87402227025345525 ) ) ;
#37155=CARTESIAN_POINT ( 'NONE',  ( 12.95609944032581673, 31.22932257616612972, -7.688727340897671958 ) ) ;
#37157=CARTESIAN_POINT ( 'NONE',  ( -17.63234478075006706, 10.48641262593123535, -29.42979450428692090 ) ) ;
#37159=CARTESIAN_POINT ( 'NONE',  ( 10.92341448429028361, -19.97047823036292158, -21.60572769884808153 ) ) ;
#37161=CARTESIAN_POINT ( 'NONE',  ( 15.72991998290128990, -16.18894361744929000, -20.11584339644706887 ) ) ;
#37164=CARTESIAN_POINT ( 'NONE',  ( -11.66180094259661182, 18.93490399102544686, -22.73092985986360404 ) ) ;
#37165=CARTESIAN_POINT ( 'NONE',  ( -24.43784849675204285, -25.81124019920631696, -8.053843953535672284 ) ) ;
#37166=CARTESIAN_POINT ( 'NONE',  ( 10.37471708997861164, -24.99497222897499782, -9.781170498600573637 ) ) ;
#37170=CARTESIAN_POINT ( 'NONE',  ( -9.313421446828321848, 28.11428578405463341, -14.94527526474085732 ) ) ;
#37177=CARTESIAN_POINT ( 'NONE',  ( 25.85566401745649756, 0.3314906535464867132, -16.44492392060781327 ) ) ;
#37182=ORIENTED_EDGE ( 'NONE', *, *, #25517, .T. ) ;
#37183=CARTESIAN_POINT ( 'NONE',  ( -20.60872544724836786, 0.8785077229891553596, -28.07890803345969388 ) ) ;
#37187=CARTESIAN_POINT ( 'NONE',  ( 27.13811364924229963, -5.609222319042479477, -16.88217377438804689 ) ) ;
#37204=CARTESIAN_POINT ( 'NONE',  ( 7.308504912602463932, 28.32893145372440813, -15.82008540585032641 ) ) ;
#37206=CARTESIAN_POINT ( 'NONE',  ( 14.21603707476194067, -21.19223970495677634, -18.18584086863970128 ) ) ;
#37207=( LENGTH_UNIT ( ) NAMED_UNIT ( * ) SI_UNIT ( .MILLI., .METRE. ) );
#37211=CARTESIAN_POINT ( 'NONE',  ( -13.78507581919008196, 23.36291329981870035, -14.47800459695361397 ) ) ;
#37214=CARTESIAN_POINT ( 'NONE',  ( 9.346475367005044887, -18.24555389153483631, -29.35143642865414648 ) ) ;
#37218=CARTESIAN_POINT ( 'NONE',  ( -13.78620412469754974, 30.29238551392001000, -6.816998145928632624 ) ) ;
#37219=CARTESIAN_POINT ( 'NONE',  ( -11.05369788186578539, -17.27790053512912039, -29.31532796641473837 ) ) ;
#37224=CARTESIAN_POINT ( 'NONE',  ( -33.72291166692595255, -10.47593345224562533, -9.784983549797274804 ) ) ;
#37225=CARTESIAN_POINT ( 'NONE',  ( -14.42315031391927604, -25.58824056110956846, -10.18640137108187105 ) ) ;
#37228=CARTESIAN_POINT ( 'NONE',  ( 23.84616085791028439, 0.7114667219658915576, -19.52213106094174933 ) ) ;
#37233=CARTESIAN_POINT ( 'NONE',  ( -28.36098518925343015, 0.1130484564961234811, -12.54774101850605206 ) ) ;
#37235=CARTESIAN_POINT ( 'NONE',  ( 22.53479768705193109, -0.8417541303772992922, -22.54520765563958307 ) ) ;
#37237=CARTESIAN_POINT ( 'NONE',  ( 10.50003573332661411, -17.62042850385381243, -30.00000000000000000 ) ) ;
#37240=CARTESIAN_POINT ( 'NONE',  ( -20.19374099270470779, 4.300116008667979273, -27.62586759252641144 ) ) ;
#37249=CARTESIAN_POINT ( 'NONE',  ( -19.55289733891971693, 6.410511261044660181, -28.26509928457950949 ) ) ;
#37252=CARTESIAN_POINT ( 'NONE',  ( 14.35507674797322153, -14.94651742297148722, -27.81134915278669340 ) ) ;
#37254=CARTESIAN_POINT ( 'NONE',  ( 10.79262732167511274, 17.48354943385782079, -28.69806840933970804 ) ) ;
#37257=CARTESIAN_POINT ( 'NONE',  ( -12.82984808660655318, 16.00373636590108362, -30.00000000000000355 ) ) ;
#37260=CARTESIAN_POINT ( 'NONE',  ( 11.01299302568612859, 17.29057472414998742, -30.00000000000000000 ) ) ;
#37264=CARTESIAN_POINT ( 'NONE',  ( -10.92223089246044587, 17.60308047634757500, -27.43605944492403381 ) ) ;
#37266=CARTESIAN_POINT ( 'NONE',  ( -10.97957011535166494, -19.95710388766885401, -21.59818507530883025 ) ) ;
#37269=CARTESIAN_POINT ( 'NONE',  ( -34.41005778243852120, -16.71535200144834832, -6.277988090640136853 ) ) ;
#37271=CARTESIAN_POINT ( 'NONE',  ( -7.523214604281919904, -19.21852453499634450, -28.17917537356595403 ) ) ;
#37273=CARTESIAN_POINT ( 'NONE',  ( 16.83483527457651974, 22.12433461383112032, -6.427118072085295175 ) ) ;
#37274=ORIENTED_EDGE ( 'NONE', *, *, #31204, .T. ) ;
#37275=CARTESIAN_POINT ( 'NONE',  ( 19.90454223993690874, 5.930672848293738753, -26.54186067485865053 ) ) ;
#37280=CARTESIAN_POINT ( 'NONE',  ( -31.08811179967121419, -0.4156326309829680432, -6.876971461052154844 ) ) ;
#37282=CARTESIAN_POINT ( 'NONE',  ( 20.48743909015156106, 0.7225425954259894201, -29.34587392400671391 ) ) ;
#37287=CARTESIAN_POINT ( 'NONE',  ( -15.72991998290134141, -16.18894361744923316, -20.11584339644716479 ) ) ;
#37289=AXIS2_PLACEMENT_3D ( 'NONE', #27449, #2873, #15461 ) ;
#37294=CARTESIAN_POINT ( 'NONE',  ( 2.684628480821892982, 37.27707400732953857, -8.408764988529911832 ) ) ;
#37303=CARTESIAN_POINT ( 'NONE',  ( 10.35162965265407387, 18.32793675510878728, -26.13581186062965145 ) ) ;
#37306=CARTESIAN_POINT ( 'NONE',  ( -17.05325914272468779, 17.02370371989225006, -14.81479654505746169 ) ) ;
#37308=ADVANCED_FACE ( 'NONE', ( #35220 ), #19174, .F. ) ;
#37310=CARTESIAN_POINT ( 'NONE',  ( 9.495448100151719473, -18.16828483302926145, -29.34839842954884048 ) ) ;
#37312=CARTESIAN_POINT ( 'NONE',  ( -17.08966005492841944, -22.85233455301158756, -15.10154554800658744 ) ) ;
#37313=CARTESIAN_POINT ( 'NONE',  ( 11.00500201062592076, 17.34882336543233450, -28.70691125584460934 ) ) ;
#37314=CARTESIAN_POINT ( 'NONE',  ( 11.46769351692955752, 18.45166467387952380, -23.85133428991321125 ) ) ;
#37315=ORIENTED_EDGE ( 'NONE', *, *, #6394, .F. ) ;
#37318=CARTESIAN_POINT ( 'NONE',  ( -14.27994367031277001, -25.05694730131601133, -11.60121664921379114 ) ) ;
#37322=CARTESIAN_POINT ( 'NONE',  ( -31.58328445775233106, -21.78494312990649462, -5.000000000000002665 ) ) ;
#37323=CARTESIAN_POINT ( 'NONE',  ( -2.574564127703440786, -24.67429484068291146, -7.426918231604072496 ) ) ;
#37324=CARTESIAN_POINT ( 'NONE',  ( 14.72309051804893798, 24.45547455918983459, -11.61434635058594900 ) ) ;
#37325=CARTESIAN_POINT ( 'NONE',  ( 18.23997498585743671, 9.357756550322328337, -29.42875180487423847 ) ) ;
#37328=CARTESIAN_POINT ( 'NONE',  ( -33.31713789998030251, -3.466154907495874848, -6.811614906419716675 ) ) ;
#37335=CARTESIAN_POINT ( 'NONE',  ( -29.73804506707628192, 0.6556055609695065067, -8.304321593376053912 ) ) ;
#37336=CARTESIAN_POINT ( 'NONE',  ( 35.42505292462669786, -13.05524145712385042, -5.000000000000000000 ) ) ;
#37348=CARTESIAN_POINT ( 'NONE',  ( -3.330156562440208745, 29.86612940616478440, -15.70309549552822226 ) ) ;
#37354=CARTESIAN_POINT ( 'NONE',  ( 12.83000963327528865, 28.50739036967297224, -11.36264415545698370 ) ) ;
#37356=CARTESIAN_POINT ( 'NONE',  ( -18.62251848404639176, 10.14620980242720272, -23.33001570770051103 ) ) ;
#37358=CARTESIAN_POINT ( 'NONE',  ( 15.36705230571556946, -26.32838276033183789, -8.290462328652061785 ) ) ;
#37360=CARTESIAN_POINT ( 'NONE',  ( 14.50667584134738775, 25.04428483107196968, -11.59352418477084434 ) ) ;
#37361=CARTESIAN_POINT ( 'NONE',  ( -26.31271763591399804, -28.25584584496044727, -14.26382729546507555 ) ) ;
#37363=CARTESIAN_POINT ( 'NONE',  ( -13.19593879056965591, 22.26071678948836308, -16.44094010185055765 ) ) ;
#37364=CARTESIAN_POINT ( 'NONE',  ( -14.57624227410516404, -14.53651728905030183, -28.50876045855337892 ) ) ;
#37365=CARTESIAN_POINT ( 'NONE',  ( 13.06131125295109996, -26.10018571120846431, -6.421009571025454221 ) ) ;
#37366=CARTESIAN_POINT ( 'NONE',  ( 15.38983201598744266, 26.43745849338104037, -6.888277659600019476 ) ) ;
#37367=CARTESIAN_POINT ( 'NONE',  ( 17.51558450279301837, -11.83370107486374501, -26.26684009027794175 ) ) ;
#37370=CARTESIAN_POINT ( 'NONE',  ( -9.589722423178423938, 32.07510805956650302, -11.18595533578888279 ) ) ;
#37377=CARTESIAN_POINT ( 'NONE',  ( 22.72129020795306786, 0.6420447253098271467, -21.62132452122856918 ) ) ;
#37383=CARTESIAN_POINT ( 'NONE',  ( -28.31117062388397443, 0.1748750734513740968, -12.55189785114625245 ) ) ;
#37386=CARTESIAN_POINT ( 'NONE',  ( 34.68475117796653251, -6.257323052730294322, -5.891097102607844249 ) ) ;
#37395=CARTESIAN_POINT ( 'NONE',  ( -7.292293556685349287, 19.17084528979847491, -29.99999999999998224 ) ) ;
#37399=CARTESIAN_POINT ( 'NONE',  ( 9.020565442340009454, 35.12981360116603469, -7.597900073285591915 ) ) ;
#37404=CARTESIAN_POINT ( 'NONE',  ( 12.61212348447421228, -20.17736113527566744, -20.35657553128955755 ) ) ;
#37405=SURFACE_STYLE_FILL_AREA ( #39845 ) ;
#37408=CARTESIAN_POINT ( 'NONE',  ( -11.63857042517895835, 18.30432797884460783, -23.87741341467080147 ) ) ;
#37411=CARTESIAN_POINT ( 'NONE',  ( 10.14633863637189393, -19.19177985329903535, -23.86353120736796640 ) ) ;
#37415=CARTESIAN_POINT ( 'NONE',  ( -13.68010871116744731, 25.96172115623508603, -12.42778920982119928 ) ) ;
#37416=CARTESIAN_POINT ( 'NONE',  ( -20.35363307782489883, -26.94962879673899181, -7.247870004610525108 ) ) ;
#37419=CARTESIAN_POINT ( 'NONE',  ( -23.37192198891547434, -6.525024743817787076, -20.88787227384175083 ) ) ;
#37420=CARTESIAN_POINT ( 'NONE',  ( -10.43671498305923606, -19.60464466685017015, -22.74714329939464363 ) ) ;
#37423=CARTESIAN_POINT ( 'NONE',  ( 29.94912702968606055, 0.2658994707610922714, -8.770941407747322671 ) ) ;
#37426=ORIENTED_EDGE ( 'NONE', *, *, #17315, .F. ) ;
#37428=CARTESIAN_POINT ( 'NONE',  ( -26.52412813069345532, 0.2470591091748601809, -15.44714408431404173 ) ) ;
#37431=CARTESIAN_POINT ( 'NONE',  ( 27.47914625674854250, -1.352420133889514764, -15.26936114680716550 ) ) ;
#37434=CARTESIAN_POINT ( 'NONE',  ( 2.793143654148522170, -20.31935452177206969, -30.00000000000001421 ) ) ;
#37437=CARTESIAN_POINT ( 'NONE',  ( -21.90799695884349774, 4.299728261586824196, -20.92328423790911884 ) ) ;
#37448=CARTESIAN_POINT ( 'NONE',  ( -23.24656352754010769, 7.851391979896635398, -11.84231981378251497 ) ) ;
#37449=CARTESIAN_POINT ( 'NONE',  ( -19.48557158514988785, -11.24999999999987743, 10.00000000000000000 ) ) ;
#37451=CARTESIAN_POINT ( 'NONE',  ( 23.11526344011869938, -26.83253816688370819, -5.000000000000002665 ) ) ;
#37453=CARTESIAN_POINT ( 'NONE',  ( 11.52907589320744464, 19.06142540582696654, -22.70785398504575170 ) ) ;
#37456=CARTESIAN_POINT ( 'NONE',  ( -15.71345004126338907, 23.14940864091746064, -10.22852350719944958 ) ) ;
#37461=CARTESIAN_POINT ( 'NONE',  ( 12.16656640916057697, 19.88180003594682788, -20.54734239706648680 ) ) ;
#37465=CARTESIAN_POINT ( 'NONE',  ( -14.93646167759306387, 26.23028568784196324, -9.225374686410800606 ) ) ;
#37467=CARTESIAN_POINT ( 'NONE',  ( -13.50903009133150334, -23.63675682006747891, -14.46352174718241024 ) ) ;
#37471=CARTESIAN_POINT ( 'NONE',  ( -24.11028944448099054, -11.71693609780529677, -18.62405750076642619 ) ) ;
#37472=CARTESIAN_POINT ( 'NONE',  ( -9.288864052834329144, -19.07931708185379449, -25.08847946617766667 ) ) ;
#37473=DIRECTION ( 'NONE',  ( -0.000000000000000000, -0.000000000000000000, 1.000000000000000000 ) ) ;
#37474=CARTESIAN_POINT ( 'NONE',  ( 16.42302884132381635, 23.18804532280490704, -6.898824423637220704 ) ) ;
#37476=CARTESIAN_POINT ( 'NONE',  ( 26.52510315481259440, 4.669929872087335454, -7.390039225938844325 ) ) ;
#37482=CARTESIAN_POINT ( 'NONE',  ( -31.16128978838004215, -0.4216671695662963515, -6.408873994583965228 ) ) ;
#37484=CARTESIAN_POINT ( 'NONE',  ( 30.50596941830245967, -0.3378608342927111874, -8.747934072216118295 ) ) ;
#37487=CARTESIAN_POINT ( 'NONE',  ( -19.54664213359414404, -11.28525909758381829, -30.00000000000000711 ) ) ;
#37496=CARTESIAN_POINT ( 'NONE',  ( 37.57549957648898697, 32.94422479542058824, 0.000000000000000000 ) ) ;
#37497=CARTESIAN_POINT ( 'NONE',  ( 2.599036944496103452, 35.98214420759691734, -10.17776264407841857 ) ) ;
#37505=CARTESIAN_POINT ( 'NONE',  ( 12.09704535053124097, 21.84084311221952746, -18.33700071698500977 ) ) ;
#37508=CARTESIAN_POINT ( 'NONE',  ( -18.27253818691323062, 18.69021931283398530, -5.478664268103901946 ) ) ;
#37511=CARTESIAN_POINT ( 'NONE',  ( 9.602585878379885642, -18.34980316067541750, -27.44912381818026859 ) ) ;
#37512=CARTESIAN_POINT ( 'NONE',  ( -22.64013887523591606, -26.77760336401204100, -6.771740173302402077 ) ) ;
#37513=CARTESIAN_POINT ( 'NONE',  ( 12.39760697099640652, 20.48158002049096282, -19.49775760875778019 ) ) ;
#37514=CARTESIAN_POINT ( 'NONE',  ( 15.01370201814430061, 25.98344539277131204, -9.237562102240422846 ) ) ;
#37517=CARTESIAN_POINT ( 'NONE',  ( -9.458459612945102180, -18.23765197637141711, -28.70940629815209633 ) ) ;
#37521=CARTESIAN_POINT ( 'NONE',  ( -16.85969849069656590, -12.36963956004071186, -26.98632881526714655 ) ) ;
#37522=CARTESIAN_POINT ( 'NONE',  ( -0.3846874604185267499, -24.60652018611802205, -7.918091565281228483 ) ) ;
#37523=CARTESIAN_POINT ( 'NONE',  ( 14.68761894541005475, 23.48803088349838220, -12.58875248005314873 ) ) ;
#37525=CARTESIAN_POINT ( 'NONE',  ( 19.48270368550455700, 8.998075144385749624, -22.23371150557425935 ) ) ;
#37528=ORIENTED_EDGE ( 'NONE', *, *, #29476, .T. ) ;
#37529=CARTESIAN_POINT ( 'NONE',  ( -20.34904904974839468, -3.057566804462165777, -28.57235194868102113 ) ) ;
#37537=CARTESIAN_POINT ( 'NONE',  ( -26.12154978825257956, 0.8729768346659233513, -15.49655606007314113 ) ) ;
#37538=CARTESIAN_POINT ( 'NONE',  ( 25.90986923523073315, -9.535114592619988727, -17.67153410330361041 ) ) ;
#37550=CARTESIAN_POINT ( 'NONE',  ( -2.819557190764113930, 25.49732518862137454, -19.66265949721264761 ) ) ;
#37556=CARTESIAN_POINT ( 'NONE',  ( 8.851496467661105427, 18.99526148928798719, -26.62540179812685892 ) ) ;
#37558=CARTESIAN_POINT ( 'NONE',  ( -17.63234478075006706, 10.48641262593123535, -29.99999999999998934 ) ) ;
#37561=CARTESIAN_POINT ( 'NONE',  ( 9.659365752239464697, -18.32200075079210322, -27.44504324438285892 ) ) ;
#37563=CARTESIAN_POINT ( 'NONE',  ( 15.37658843025399413, 26.83106350242916704, -5.945231630724503447 ) ) ;
#37564=CARTESIAN_POINT ( 'NONE',  ( 22.45323650136968396, -2.382502413133517738, -29.99999999999998934 ) ) ;
#37566=CARTESIAN_POINT ( 'NONE',  ( -27.04961384508420608, -25.34883885810744886, -5.441318665117593767 ) ) ;
#37567=CARTESIAN_POINT ( 'NONE',  ( 9.100901191155434944, -19.97180529156877782, -22.89666456064600908 ) ) ;
#37568=CARTESIAN_POINT ( 'NONE',  ( 15.43128619640941857, 26.46390025712458183, -6.417237675877188963 ) ) ;
#37569=CARTESIAN_POINT ( 'NONE',  ( 22.18477674033645286, -15.00887286453208169, -18.62664606145825275 ) ) ;
#37573=CARTESIAN_POINT ( 'NONE',  ( -5.489946483366239249, 20.60753015119807330, -25.73531879562920111 ) ) ;
#37580=CARTESIAN_POINT ( 'NONE',  ( 30.89317523684279010, -0.03095884371312799394, -5.000000000000000000 ) ) ;
#37583=CARTESIAN_POINT ( 'NONE',  ( -37.48557158514985588, -11.24999999999982414, 6.000000000000000000 ) ) ;
#37587=CARTESIAN_POINT ( 'NONE',  ( -30.81224694139058329, 0.01613667459859374764, -5.946089668811439743 ) ) ;
#37589=CARTESIAN_POINT ( 'NONE',  ( -20.35363302287704101, -26.94962880062152877, -7.247870005599446053 ) ) ;
#37591=CARTESIAN_POINT ( 'NONE',  ( 27.93478377975757354, -4.930528639082491615, -15.96261009728761060 ) ) ;
#37602=CARTESIAN_POINT ( 'NONE',  ( -4.769256462637533112, 19.93975062605538184, -29.99999999999996803 ) ) ;
#37603=DIRECTION ( 'NONE',  ( 0.000000000000000000, 0.000000000000000000, 1.000000000000000000 ) ) ;
#37605=CARTESIAN_POINT ( 'NONE',  ( 14.52284994691540554, 15.12055744848739458, -25.35930744202923393 ) ) ;
#37606=CARTESIAN_POINT ( 'NONE',  ( 8.493348210982047064, 32.87541910339748341, -11.15327735273583620 ) ) ;
#37610=CARTESIAN_POINT ( 'NONE',  ( 17.77051926636400836, -26.05666342080411013, -10.02570539512946901 ) ) ;
#37614=ORIENTED_EDGE ( 'NONE', *, *, #4895, .F. ) ;
#37615=CARTESIAN_POINT ( 'NONE',  ( -11.07958958704495167, 17.49807219138947545, -27.44831219198803396 ) ) ;
#37617=CARTESIAN_POINT ( 'NONE',  ( 15.18788860438108124, -26.66571922823320051, -5.474128979186436261 ) ) ;
#37621=CARTESIAN_POINT ( 'NONE',  ( -10.01402912130534162, 17.90039694996872655, -29.32746991544585313 ) ) ;
#37624=CARTESIAN_POINT ( 'NONE',  ( -19.56896045557411767, -6.106514739740910969, -29.23677687923446911 ) ) ;
#37625=CARTESIAN_POINT ( 'NONE',  ( -15.36059797614417199, -26.70982037388659691, -5.000000000000000888 ) ) ;
#37628=CARTESIAN_POINT ( 'NONE',  ( 30.61281600001173686, 0.2212781233926191804, -5.946150247221624774 ) ) ;
#37632=CARTESIAN_POINT ( 'NONE',  ( -30.02005750921860638, -0.001135212662567658751, -9.236802755891959649 ) ) ;
#37635=CARTESIAN_POINT ( 'NONE',  ( 23.05089902286179893, -0.5612348335507770791, -21.46137821024467840 ) ) ;
#37641=CARTESIAN_POINT ( 'NONE',  ( -14.98890122036483419, -28.67928442680469203, -4.999999999999999112 ) ) ;
#37643=CARTESIAN_POINT ( 'NONE',  ( -15.48853126089653642, -26.74269726827072446, -4.999999999999999112 ) ) ;
#37648=CARTESIAN_POINT ( 'NONE',  ( -20.30282733015013363, 7.292259425124786532, -22.18016511663011059 ) ) ;
#37649=CARTESIAN_POINT ( 'NONE',  ( 21.74762051904238191, -24.00969798870548644, -12.12483235932745984 ) ) ;
#37652=CARTESIAN_POINT ( 'NONE',  ( 12.28203363025439288, 20.63554315272105555, -19.47339641021015311 ) ) ;
#37654=CARTESIAN_POINT ( 'NONE',  ( -13.08623023714802258, 18.08879695936160203, -21.80946885493514031 ) ) ;
#37657=CARTESIAN_POINT ( 'NONE',  ( 11.03147510093559269, 17.33177591260932715, -28.70801338942442982 ) ) ;
#37661=ORIENTED_EDGE ( 'NONE', *, *, #25378, .T. ) ;
#37662=CARTESIAN_POINT ( 'NONE',  ( -15.26899636581957687, 27.02509300740851472, -6.411569543597564369 ) ) ;
#37664=CARTESIAN_POINT ( 'NONE',  ( -13.14311512211350852, -23.10060485217718096, -15.43729266571827097 ) ) ;
#37667=CARTESIAN_POINT ( 'NONE',  ( -33.45518794257092310, -14.98363075432738789, -9.291991822186489003 ) ) ;
#37668=CARTESIAN_POINT ( 'NONE',  ( -12.02413919917706764, -23.04697477249095883, -15.51450891573247048 ) ) ;
#37670=CARTESIAN_POINT ( 'NONE',  ( 12.38972167065434782, 16.33584955698245977, -30.00000000000000711 ) ) ;
#37672=CARTESIAN_POINT ( 'NONE',  ( 25.47574744270427516, 5.541576092252077146, -9.334551064280120158 ) ) ;
#37674=CARTESIAN_POINT ( 'NONE',  ( 15.48853125999100833, -26.74269726803731118, -5.000000000000000000 ) ) ;
#37676=EDGE_LOOP ( 'NONE', ( #11552, #34173, #12805, #36866 ) ) ;
#37677=CARTESIAN_POINT ( 'NONE',  ( -26.07300228947948284, -0.03011411378347995590, -16.39941592429670081 ) ) ;
#37679=CARTESIAN_POINT ( 'NONE',  ( 20.82749634169985953, 0.6853679382005627430, -26.81932549163500568 ) ) ;
#37685=CARTESIAN_POINT ( 'NONE',  ( -26.31271763591404422, -28.25584584496042240, -5.000000000000000888 ) ) ;
#37688=ORIENTED_EDGE ( 'NONE', *, *, #2798, .F. ) ;
#37690=DIRECTION ( 'NONE',  ( 1.000000000000000000, 0.000000000000000000, 0.000000000000000000 ) ) ;
#37693=CARTESIAN_POINT ( 'NONE',  ( 4.646098203774434943, 34.72221286985408284, -11.08844531243078890 ) ) ;
#37702=CARTESIAN_POINT ( 'NONE',  ( 14.60593664522046353, 26.75915035538402265, -9.657648197979836979 ) ) ;
#37706=CARTESIAN_POINT ( 'NONE',  ( -18.18070401533917035, 18.56346265111594462, -7.404067847983029083 ) ) ;
#37710=CARTESIAN_POINT ( 'NONE',  ( 11.89284648857719695, -21.48584275349674400, -18.45356361586392779 ) ) ;
#37712=CARTESIAN_POINT ( 'NONE',  ( 14.94089887612034673, 25.78092154341846864, -9.709267021671619702 ) ) ;
#37714=CARTESIAN_POINT ( 'NONE',  ( 11.28971518877922264, 18.05388930042798634, -25.01178682049573609 ) ) ;
#37717=CARTESIAN_POINT ( 'NONE',  ( -14.67000517685553440, -25.63834831813752047, -10.18194144610326468 ) ) ;
#37719=CARTESIAN_POINT ( 'NONE',  ( -30.45757913935707961, -22.41806408542251816, -7.125453223155250093 ) ) ;
#37720=CARTESIAN_POINT ( 'NONE',  ( -2.095722264221089315, -22.15702150879218024, -19.05869434001748886 ) ) ;
#37721=CARTESIAN_POINT ( 'NONE',  ( 13.54937698026857262, 21.63598032874356036, -16.49571944579557936 ) ) ;
#37723=CARTESIAN_POINT ( 'NONE',  ( 18.58241799660420668, 8.688807075854512618, -29.99999999999999645 ) ) ;
#37726=ORIENTED_EDGE ( 'NONE', *, *, #9525, .F. ) ;
#37727=CARTESIAN_POINT ( 'NONE',  ( -20.65377969610915443, -2.455125782780259502, -27.23826263681096549 ) ) ;
#37734=CARTESIAN_POINT ( 'NONE',  ( -20.67119347756820602, 2.193161261697490705, -26.92867794748204702 ) ) ;
#37735=CARTESIAN_POINT ( 'NONE',  ( 21.94494290708799866, -8.860422532852833655, -21.89653876190107340 ) ) ;
#37745=CARTESIAN_POINT ( 'NONE',  ( -1.902173617953080376, 37.83571591983437088, -7.545775875163593049 ) ) ;
#37752=CARTESIAN_POINT ( 'NONE',  ( 13.61253233593243550, 30.46620566788191198, -7.261355557076043965 ) ) ;
#37755=CARTESIAN_POINT ( 'NONE',  ( -18.11210683354745044, 9.887672296931658167, -27.17641187830589189 ) ) ;
#37757=CARTESIAN_POINT ( 'NONE',  ( 13.07450261122289881, -23.09593886341139779, -15.44440162208020872 ) ) ;
#37760=CARTESIAN_POINT ( 'NONE',  ( 12.89273306925234586, 21.71245797589364912, -17.42948357415733796 ) ) ;
#37761=CARTESIAN_POINT ( 'NONE',  ( 20.90924525106828114, -8.502318254486461058, -19.80438750953544513 ) ) ;
#37763=CARTESIAN_POINT ( 'NONE',  ( -23.45180357993919884, -24.82439038927461183, -10.28237032673689733 ) ) ;
#37764=CARTESIAN_POINT ( 'NONE',  ( 5.727881898942783323, -19.93915831793329119, -27.08029247955964891 ) ) ;
#37765=CARTESIAN_POINT ( 'NONE',  ( 11.99126504055620224, 19.27700041912028084, -21.63417993446100240 ) ) ;
#37766=CARTESIAN_POINT ( 'NONE',  ( 18.50037648924358891, -13.33006404268201273, -23.01361493332205299 ) ) ;
#37769=EDGE_LOOP ( 'NONE', ( #32054, #25147, #38817, #4547 ) ) ;
#37770=CARTESIAN_POINT ( 'NONE',  ( -8.976254749716225945, 33.67889951363163448, -9.809507123318200073 ) ) ;
#37773=CARTESIAN_POINT ( 'NONE',  ( 30.90370714462332202, -0.07739494692734212589, -5.945536237155164550 ) ) ;
#37778=CARTESIAN_POINT ( 'NONE',  ( -22.72062348006680921, 0.6442621738748725013, -21.62159724769585267 ) ) ;
#37781=CARTESIAN_POINT ( 'NONE',  ( 19.94806447466153543, -4.723319992639698484, -29.99999999999998579 ) ) ;
#37783=ORIENTED_EDGE ( 'NONE', *, *, #15504, .T. ) ;
#37785=CARTESIAN_POINT ( 'NONE',  ( 19.48557158514982746, -11.25000000000009415, 3.000000000000000000 ) ) ;
#37786=CARTESIAN_POINT ( 'NONE',  ( -20.71630303010418572, -29.20803740758281464, -4.999999999999997335 ) ) ;
#37790=CARTESIAN_POINT ( 'NONE',  ( -5.408911131318492771, 19.77578011155457816, -29.99999999999996803 ) ) ;
#37793=CARTESIAN_POINT ( 'NONE',  ( 14.28645338827841726, 14.73924105482272751, -28.81583157955228458 ) ) ;
#37795=CARTESIAN_POINT ( 'NONE',  ( 6.508078574177585729, 28.74780359284325826, -15.78726989322525398 ) ) ;
#37799=CARTESIAN_POINT ( 'NONE',  ( 16.20692150584794078, -26.83310280674016468, -6.404917216296185600 ) ) ;
#37803=CARTESIAN_POINT ( 'NONE',  ( -15.41471391286399317, 26.78795929021520550, -5.474190302194672952 ) ) ;
#37806=CARTESIAN_POINT ( 'NONE',  ( 14.40512807539449547, -25.86522860305755600, -9.245460395081696703 ) ) ;
#37810=EDGE_LOOP ( 'NONE', ( #9037, #9787 ) ) ;
#37812=CARTESIAN_POINT ( 'NONE',  ( -13.19605298241623714, 31.11796965224743516, -7.247223247613001185 ) ) ;
#37815=CARTESIAN_POINT ( 'NONE',  ( -30.13885734736032518, -8.367891793043197524, -13.92058473770290661 ) ) ;
#37817=ORIENTED_EDGE ( 'NONE', *, *, #16535, .F. ) ;
#37818=CARTESIAN_POINT ( 'NONE',  ( 20.80626354190386351, 0.9384790171570499551, -26.83885795680234310 ) ) ;
#37822=CARTESIAN_POINT ( 'NONE',  ( -27.16660938874878539, 0.1989104985245108981, -14.47297071791797052 ) ) ;
#37824=CARTESIAN_POINT ( 'NONE',  ( 28.64846384017765502, -1.091167704362612678, -13.38480877307776851 ) ) ;
#37825=CARTESIAN_POINT ( 'NONE',  ( 0.04788021487524250774, -20.50383365384739776, -30.00000000000000711 ) ) ;
#37833=CIRCLE ( 'NONE', #25498, 21.00000000000002842 ) ;
#37839=CARTESIAN_POINT ( 'NONE',  ( -22.59715888466356049, 9.764328767929328023, -9.387076417448387389 ) ) ;
#37840=CARTESIAN_POINT ( 'NONE',  ( 13.26265854479622419, -15.63203989815269779, -29.26899939535988437 ) ) ;
#37843=CARTESIAN_POINT ( 'NONE',  ( 15.17653370639157728, 26.59493482429561340, -7.821537767519052053 ) ) ;
#37845=CARTESIAN_POINT ( 'NONE',  ( -14.56238555350499020, 22.71997793191525616, -13.57281493169755571 ) ) ;
#37849=CARTESIAN_POINT ( 'NONE',  ( 13.50802936482910610, 22.78328071161119794, -15.45283427980578139 ) ) ;
#37852=CARTESIAN_POINT ( 'NONE',  ( 18.02495589071083160, -9.945986095653781334, -28.44476012898337203 ) ) ;
#37855=CARTESIAN_POINT ( 'NONE',  ( -15.11187235763720160, 27.11521598415787437, -7.341895426520673062 ) ) ;
#37857=CARTESIAN_POINT ( 'NONE',  ( -13.24241402396536849, -21.98623490292562721, -17.32878092716321561 ) ) ;
#37861=CARTESIAN_POINT ( 'NONE',  ( -30.04644516860189185, -14.57369536713954083, -12.89617642488422966 ) ) ;
#37862=CARTESIAN_POINT ( 'NONE',  ( -10.24989465074190420, -20.12788835074411864, -21.68738911211123721 ) ) ;
#37864=CARTESIAN_POINT ( 'NONE',  ( 16.87377372029358469, 22.19217076240406428, -5.475293046584253531 ) ) ;
#37866=CARTESIAN_POINT ( 'NONE',  ( 19.90281409743823815, 5.211047685906170734, -28.23787101014183420 ) ) ;
#37871=CARTESIAN_POINT ( 'NONE',  ( -30.89143654367048342, -0.3087187454278746968, -7.347449338435406929 ) ) ;
#37872=CARTESIAN_POINT ( 'NONE',  ( 26.66507754537762409, 0.03537578240675859353, -15.42101455173288649 ) ) ;
#37877=CARTESIAN_POINT ( 'NONE',  ( 17.81784622497951176, -13.85677843414110555, -19.80438750953540961 ) ) ;
#37882=CIRCLE ( 'NONE', #19074, 57.00000000000003553 ) ;
#37885=CARTESIAN_POINT ( 'NONE',  ( 5.962758689501411524, 36.33297212300762880, -8.430188468140666913 ) ) ;
#37890=CARTESIAN_POINT ( 'NONE',  ( 16.99588821486303303, -13.03532880417942508, -25.61570463410847154 ) ) ;
#37894=CARTESIAN_POINT ( 'NONE',  ( -15.41558956984166251, 26.78481017248024898, -5.000000000000000000 ) ) ;
#37895=CARTESIAN_POINT ( 'NONE',  ( 10.43719446462658240, 17.70184934034695345, -28.68331232917914164 ) ) ;
#37897=VERTEX_POINT ( 'NONE', #38823 ) ;
#37898=CARTESIAN_POINT ( 'NONE',  ( -14.97620661933688346, 15.43604710290467708, -23.16381367993152907 ) ) ;
#37903=CARTESIAN_POINT ( 'NONE',  ( 9.684905122972589098, -18.44378311763584577, -26.83090883577152397 ) ) ;
#37905=CARTESIAN_POINT ( 'NONE',  ( 13.49439698208447602, 22.80992317807017500, -15.45087343220999010 ) ) ;
#37906=ORIENTED_EDGE ( 'NONE', *, *, #7689, .T. ) ;
#37907=CARTESIAN_POINT ( 'NONE',  ( 11.11724078106343683, 17.61836477313612193, -26.82968543565921848 ) ) ;
#37911=CARTESIAN_POINT ( 'NONE',  ( -9.759121109861677468, -18.57581161978397688, -26.22736366997701651 ) ) ;
#37915=CARTESIAN_POINT ( 'NONE',  ( -21.53702042946260420, -15.83689332051200616, -18.64419367562588192 ) ) ;
#37916=CARTESIAN_POINT ( 'NONE',  ( -3.457094704751060288, -20.82358164328624639, -24.37237690483107855 ) ) ;
#37917=CARTESIAN_POINT ( 'NONE',  ( 11.59920991657710942, 17.45000162638225660, -26.26810536156576603 ) ) ;
#37919=CARTESIAN_POINT ( 'NONE',  ( 18.58241799660420668, 8.688807075854512618, -29.42769849846112606 ) ) ;
#37923=CARTESIAN_POINT ( 'NONE',  ( -20.59263868462731750, -3.100282240389482080, -27.20017962400196865 ) ) ;
#37931=CARTESIAN_POINT ( 'NONE',  ( 27.50296097836364240, -12.04087961669551987, -15.70514145711053899 ) ) ;
#37937=DIRECTION ( 'NONE',  ( -0.000000000000000000, -0.000000000000000000, 1.000000000000000000 ) ) ;
#37941=CARTESIAN_POINT ( 'NONE',  ( -0.7532367600618588011, 38.47464941728308929, -5.855549327213532607 ) ) ;
#37949=CARTESIAN_POINT ( 'NONE',  ( 13.30718649135118348, 26.63099661339894197, -12.38017239920473678 ) ) ;
#37953=CARTESIAN_POINT ( 'NONE',  ( -18.82575331703998955, 11.22376865745672880, -20.12444327678071332 ) ) ;
#37957=CARTESIAN_POINT ( 'NONE',  ( 14.80057364270156484, -25.66573095307622054, -10.17772232356911211 ) ) ;
#37959=CARTESIAN_POINT ( 'NONE',  ( 15.14564224390120373, 26.37900145172237032, -8.294075276387847140 ) ) ;
#37960=CARTESIAN_POINT ( 'NONE',  ( -16.24796006241077961, 15.88921519459651499, -21.50719306941234876 ) ) ;
#37962=CARTESIAN_POINT ( 'NONE',  ( -19.94212141337140665, -19.90605279271622408, -16.79278165465914796 ) ) ;
#37963=CARTESIAN_POINT ( 'NONE',  ( 8.467881093281681260, -25.26349163305798839, -6.435158416897623468 ) ) ;
#37964=CARTESIAN_POINT ( 'NONE',  ( 11.81931059556923103, 18.78345403663103852, -22.75672908190094645 ) ) ;
#37965=CARTESIAN_POINT ( 'NONE',  ( 29.70735205375613219, -21.47756445264377589, -9.292127997619706647 ) ) ;
#37966=DIRECTION ( 'NONE',  ( -0.000000000000000000, -0.000000000000000000, 1.000000000000000000 ) ) ;
#37969=CARTESIAN_POINT ( 'NONE',  ( -6.748174487910753250, 28.62818041414330850, -15.79635236281668931 ) ) ;
#37973=CARTESIAN_POINT ( 'NONE',  ( 30.50043281132222717, -0.02822430422811177814, -7.827654197346148202 ) ) ;
#37978=CARTESIAN_POINT ( 'NONE',  ( -28.76033270383555518, 0.2571929453871795168, -11.60468438384830847 ) ) ;
#37981=CARTESIAN_POINT ( 'NONE',  ( 35.01769949592260645, -8.410817939179214164, -6.748082837904874509 ) ) ;
#37985=ORIENTED_EDGE ( 'NONE', *, *, #8762, .T. ) ;
#37993=SURFACE_STYLE_USAGE ( .BOTH. , #22542 ) ;
#37997=CARTESIAN_POINT ( 'NONE',  ( 15.17757647933641785, 16.16795567397082678, -20.97689461799007304 ) ) ;
#37998=CARTESIAN_POINT ( 'NONE',  ( 9.968257018404958814, 34.74234079311501233, -6.744892496327541842 ) ) ;
#38000=CARTESIAN_POINT ( 'NONE',  ( 12.67385491020283439, -21.41802064514664750, -18.35960277857459033 ) ) ;
#38006=CARTESIAN_POINT ( 'NONE',  ( -15.34056339507122324, 26.60929180672939509, -6.888178519148794976 ) ) ;
#38009=CARTESIAN_POINT ( 'NONE',  ( 13.52481987067865532, -24.53642209463285084, -12.56943988586981398 ) ) ;
#38010=CARTESIAN_POINT ( 'NONE',  ( 19.48557158514982746, -11.25000000000009415, 3.000000000000000000 ) ) ;
#38013=CARTESIAN_POINT ( 'NONE',  ( -8.267738057345434655, 18.77097771606736032, -29.29219651185118067 ) ) ;
#38014=CARTESIAN_POINT ( 'NONE',  ( -17.60052854559279467, -23.51059659377553501, -14.14515744271393238 ) ) ;
#38016=CARTESIAN_POINT ( 'NONE',  ( -20.25697106145711146, -4.992088383670172824, -27.10335080208274050 ) ) ;
#38019=CARTESIAN_POINT ( 'NONE',  ( 24.47508212618827628, 0.6084701833738710430, -18.47132725458562419 ) ) ;
#38023=CARTESIAN_POINT ( 'NONE',  ( -28.90304507515644517, 0.08656617661839061117, -11.59782457920430687 ) ) ;
#38026=CARTESIAN_POINT ( 'NONE',  ( 20.50882952253471103, -1.590216141173560249, -28.62054632307110680 ) ) ;
#38027=CARTESIAN_POINT ( 'NONE',  ( 20.46225145915602894, 1.418922334520018591, -30.00000000000000355 ) ) ;
#38043=CARTESIAN_POINT ( 'NONE',  ( -23.26956309474883966, 8.880304990950326882, -8.885970393110802945 ) ) ;
#38044=CARTESIAN_POINT ( 'NONE',  ( 21.65887295875352692, -26.69628545518032325, -7.666996354092982635 ) ) ;
#38046=CARTESIAN_POINT ( 'NONE',  ( 13.41755757912196323, 22.96584331339203544, -15.43348952276526731 ) ) ;
#38048=CARTESIAN_POINT ( 'NONE',  ( -15.41005911881606849, 24.37590047215257982, -9.731608369055816610 ) ) ;
#38052=CARTESIAN_POINT ( 'NONE',  ( 13.79295119906300116, 23.34604900139666483, -14.47902606294586469 ) ) ;
#38054=CARTESIAN_POINT ( 'NONE',  ( 26.45322076532816524, -14.58567879916042287, -15.67905774910988193 ) ) ;
#38057=CARTESIAN_POINT ( 'NONE',  ( -12.79458690931549292, 21.87333156960552927, -17.40760258954136219 ) ) ;
#38059=CARTESIAN_POINT ( 'NONE',  ( -16.75447718561904864, -27.02424154557581915, -5.468381619150384232 ) ) ;
#38063=CARTESIAN_POINT ( 'NONE',  ( -34.61197078468903499, -14.29155545462818111, -7.558879141708873206 ) ) ;
#38064=CARTESIAN_POINT ( 'NONE',  ( -13.74012441838748622, -25.29379767668099888, -10.67230615080171496 ) ) ;
#38066=CARTESIAN_POINT ( 'NONE',  ( 14.83232221668444595, 20.29379547517063997, -15.62825253669702263 ) ) ;
#38068=CARTESIAN_POINT ( 'NONE',  ( 27.20667665144295455, 2.902151610605352872, -10.24982003146635812 ) ) ;
#38072=CARTESIAN_POINT ( 'NONE',  ( -30.45015951236765517, -0.2748756232826376489, -8.751359642228980107 ) ) ;
#38073=CARTESIAN_POINT ( 'NONE',  ( 30.48202640438653432, -0.5154105689507647581, -9.204797512474263144 ) ) ;
#38076=EDGE_CURVE ( 'NONE', #17093, #38149, #30082, .T. ) ;
#38077=CARTESIAN_POINT ( 'NONE',  ( 31.47283671532267846, -25.12609584734865464, -14.45070082761209207 ) ) ;
#38089=CARTESIAN_POINT ( 'NONE',  ( 19.98643085710752132, -17.36878015847262446, -18.71496154814925461 ) ) ;
#38093=CARTESIAN_POINT ( 'NONE',  ( 14.32388773374254320, 25.53991067870101972, -11.55678267441725460 ) ) ;
#38097=CARTESIAN_POINT ( 'NONE',  ( -14.58236326528782989, 14.81821449170132787, -26.51297324595556759 ) ) ;
#38101=CARTESIAN_POINT ( 'NONE',  ( 15.01285564717599463, -26.13052058328588956, -8.768336206249326636 ) ) ;
#38104=CARTESIAN_POINT ( 'NONE',  ( 11.18751224735468597, 17.75405741225261735, -26.22522718368986361 ) ) ;
#38105=ORIENTED_EDGE ( 'NONE', *, *, #39843, .F. ) ;
#38106=CARTESIAN_POINT ( 'NONE',  ( 15.41298789278284964, 26.79417030376202291, -5.000000000000000000 ) ) ;
#38108=CARTESIAN_POINT ( 'NONE',  ( -15.31337224364676430, 26.70488253798198031, -6.886087685327574093 ) ) ;
#38110=CARTESIAN_POINT ( 'NONE',  ( -11.86903598408506610, -21.48771982887699750, -18.45589563282124601 ) ) ;
#38112=CARTESIAN_POINT ( 'NONE',  ( -31.37628010478545804, -21.64920164695394789, -6.699869314472419290 ) ) ;
#38113=CARTESIAN_POINT ( 'NONE',  ( -2.493492096549495773, -24.25124555584876518, -10.38337496618507849 ) ) ;
#38114=CARTESIAN_POINT ( 'NONE',  ( 11.41005643133681957, 17.03110932016596735, -30.00000000000000000 ) ) ;
#38116=CARTESIAN_POINT ( 'NONE',  ( 22.83139634148907504, 9.074226536428001921, -10.36981227567709318 ) ) ;
#38117=CARTESIAN_POINT ( 'NONE',  ( 34.79718219320302097, -16.04917476651427677, -4.999999999999997335 ) ) ;
#38120=CARTESIAN_POINT ( 'NONE',  ( -32.45035485798955222, -3.331808296535164970, -9.070745509778980420 ) ) ;
#38126=CARTESIAN_POINT ( 'NONE',  ( 3.485571585149744411, -11.24999999999998224, 10.00000000000000000 ) ) ;
#38129=CARTESIAN_POINT ( 'NONE',  ( 19.59228734373462899, -7.919684095842580263, -26.29579143822741827 ) ) ;
#38138=CARTESIAN_POINT ( 'NONE',  ( -0.4159103488080192479, 21.44268089392220134, -25.57552980935893672 ) ) ;
#38146=CARTESIAN_POINT ( 'NONE',  ( 13.64911103968386108, 28.40416279045285108, -10.02753699536989451 ) ) ;
#38149=VERTEX_POINT ( 'NONE', #15641 ) ;
#38150=CARTESIAN_POINT ( 'NONE',  ( -19.84768973869175923, 14.36017750439766871, -9.881426833975718083 ) ) ;
#38153=CARTESIAN_POINT ( 'NONE',  ( 12.32002675448889661, -22.02230990502341967, -17.43383621429965302 ) ) ;
#38155=CARTESIAN_POINT ( 'NONE',  ( 15.27745585280835705, 26.57502206593006022, -7.356517642319687411 ) ) ;
#38157=CARTESIAN_POINT ( 'NONE',  ( -35.84808252048276955, -3.038699442442200027, -5.000000000000002665 ) ) ;
#38161=CARTESIAN_POINT ( 'NONE',  ( -26.03722647915365584, -25.89241862741840094, -5.442903191855394063 ) ) ;
#38162=CARTESIAN_POINT ( 'NONE',  ( 5.759131531303930629, -23.85034579298850232, -12.81924329913233152 ) ) ;
#38163=CARTESIAN_POINT ( 'NONE',  ( 13.56948375875568580, 22.66347568585478101, -15.46163780264717147 ) ) ;
#38164=B_SPLINE_CURVE_WITH_KNOTS ( 'NONE', 3,
 ( #15053, #27644, #11417, #33363, #39831, #14660, #36790, #27051, #40026, #39436 ),
 .UNSPECIFIED., .F., .F.,
 ( 4, 1, 1, 1, 1, 1, 1, 4 ),
 ( 0.1282122296533009798, 0.2500000000108080211, 0.3749999999994781952, 0.4999999999881489243, 0.6249999999768196535, 0.7499999999654909377, 0.8749999999541600015, 1.000000000000000000 ),
 .UNSPECIFIED. ) ;
#38165=CARTESIAN_POINT ( 'NONE',  ( 31.11517615530266667, -21.06909056454590612, -7.976281376848859850 ) ) ;
#38169=CARTESIAN_POINT ( 'NONE',  ( -5.552924998094717957, 23.69300943437540852, -20.85599012649669959 ) ) ;
#38172=ORIENTED_EDGE ( 'NONE', *, *, #2619, .F. ) ;
#38173=CARTESIAN_POINT ( 'NONE',  ( 28.37209621850218610, 0.09959924578248532945, -12.54634125719528370 ) ) ;
#38177=CARTESIAN_POINT ( 'NONE',  ( -20.47826699597012023, 0.9446083685552523201, -30.00000000000000000 ) ) ;
#38181=CARTESIAN_POINT ( 'NONE',  ( 21.88878013244432097, -5.201535098629216591, -23.24105192260414654 ) ) ;
#38184=ORIENTED_EDGE ( 'NONE', *, *, #3166, .T. ) ;
#38199=CARTESIAN_POINT ( 'NONE',  ( 17.52599447534131727, 19.76765755371411615, -8.359901029784603921 ) ) ;
#38200=CARTESIAN_POINT ( 'NONE',  ( 11.51234731484127138, 32.76683130581704972, -8.088018125610085818 ) ) ;
#38204=CARTESIAN_POINT ( 'NONE',  ( 11.52690546367544222, -19.81741541769655512, -21.52521232598608947 ) ) ;
#38211=CARTESIAN_POINT ( 'NONE',  ( -11.49511999468828272, 18.42800739041194902, -23.85559909385690247 ) ) ;
#38214=CARTESIAN_POINT ( 'NONE',  ( 14.94022627794961089, -26.48256000415716471, -6.888844992090954911 ) ) ;
#38219=CARTESIAN_POINT ( 'NONE',  ( -8.958378443170586181, 18.74800665029167135, -27.28932216422303370 ) ) ;
#38222=CARTESIAN_POINT ( 'NONE',  ( -35.03892046201376331, -7.681061316508860592, -5.883781484302339493 ) ) ;
#38225=CARTESIAN_POINT ( 'NONE',  ( 20.68604710019807769, 0.9517672083310861897, -27.45507450208132738 ) ) ;
#38229=CARTESIAN_POINT ( 'NONE',  ( -27.15044877466180751, 0.2209970037928831732, -14.47560764752908824 ) ) ;
#38233=CARTESIAN_POINT ( 'NONE',  ( 21.07461541020998297, -1.002319088913975476, -26.06574103777582962 ) ) ;
#38234=CARTESIAN_POINT ( 'NONE',  ( 20.16769042714938109, -3.693422412194586446, -29.99999999999997868 ) ) ;
#38248=CARTESIAN_POINT ( 'NONE',  ( -19.05143584731581186, 7.817709358104996120, -27.71748753264345311 ) ) ;
#38249=CARTESIAN_POINT ( 'NONE',  ( 13.24265028322465731, -16.59376028717886342, -25.88933090075440191 ) ) ;
#38252=CARTESIAN_POINT ( 'NONE',  ( 15.04512796001890074, 26.32317767946528164, -8.759451899191230240 ) ) ;
#38254=CARTESIAN_POINT ( 'NONE',  ( -15.85862229823199776, 25.25472105652747246, -5.474027676197895431 ) ) ;
#38257=CARTESIAN_POINT ( 'NONE',  ( 11.08276198488759867, 17.39680518735769965, -28.07995138869140206 ) ) ;
#38259=CARTESIAN_POINT ( 'NONE',  ( 18.60907781376031522, -9.552212779558386657, -26.96908054186706494 ) ) ;
#38263=CARTESIAN_POINT ( 'NONE',  ( -14.87679345494665029, 26.41285975656771612, -9.216490526136041694 ) ) ;
#38265=CARTESIAN_POINT ( 'NONE',  ( -16.11582280033900005, -26.76908378381648390, -6.872361183095262227 ) ) ;
#38269=CARTESIAN_POINT ( 'NONE',  ( -35.15805814088607661, -13.30077706419156414, -6.711668136891848491 ) ) ;
#38270=CARTESIAN_POINT ( 'NONE',  ( -12.65038256605562772, -23.99880442748382947, -13.56128062147820579 ) ) ;
#38272=CARTESIAN_POINT ( 'NONE',  ( 16.40281439508208194, 21.37890742408058031, -10.26485299642392945 ) ) ;
#38274=CARTESIAN_POINT ( 'NONE',  ( 20.30148177599484427, 3.803005773571547454, -27.60600077430455102 ) ) ;
#38279=CARTESIAN_POINT ( 'NONE',  ( -29.04989216121797213, -0.08486885121559410716, -11.58176799329598516 ) ) ;
#38280=CARTESIAN_POINT ( 'NONE',  ( 24.14174240845033026, 0.003122030948076066903, -19.43079603134119893 ) ) ;
#38283=CARTESIAN_POINT ( 'NONE',  ( 4.336808689942017736E-15, 40.84107189184581443, -5.000000000000008882 ) ) ;
#38294=CARTESIAN_POINT ( 'NONE',  ( 27.36121244743086578, -25.22392150776288133, -5.440726707707272958 ) ) ;
#38298=CARTESIAN_POINT ( 'NONE',  ( 10.55968626961773360, 17.57118088696260827, -30.00000000000000355 ) ) ;
#38301=CARTESIAN_POINT ( 'NONE',  ( -14.46390983480181092, 16.02145941329244394, -23.10970177944547643 ) ) ;
#38304=CARTESIAN_POINT ( 'NONE',  ( 11.17102189095818687, -20.47090416160008886, -20.54315939279690895 ) ) ;
#38306=CARTESIAN_POINT ( 'NONE',  ( 15.40963821861455862, 26.71342488439698570, -5.946084157768660283 ) ) ;
#38308=CARTESIAN_POINT ( 'NONE',  ( 15.01833821314314044, 25.96818848446413952, -9.238322678839537616 ) ) ;
#38310=CARTESIAN_POINT ( 'NONE',  ( -14.98463571429964780, 26.07793220091295083, -9.232870696221679552 ) ) ;
#38312=CARTESIAN_POINT ( 'NONE',  ( -9.667542991474126879, -18.45194233073163659, -26.83237868059747555 ) ) ;
#38314=CARTESIAN_POINT ( 'NONE',  ( -32.98459937871956527, -19.91850110786283423, -4.999999999999999112 ) ) ;
#38315=CARTESIAN_POINT ( 'NONE',  ( -4.727592086853887210, -24.67674636019700785, -8.392755456812066583 ) ) ;
#38316=CARTESIAN_POINT ( 'NONE',  ( 15.37979459131270588, 24.85259051631702221, -9.252807986672786811 ) ) ;
#38319=CARTESIAN_POINT ( 'NONE',  ( 19.30637010739042125, 7.335522903491736635, -27.14430384761622861 ) ) ;
#38322=CARTESIAN_POINT ( 'NONE',  ( -2.510240365544621266, -24.77672057674680772, -5.000000000000000888 ) ) ;
#38326=CARTESIAN_POINT ( 'NONE',  ( -29.26784074738422703, -2.117567468756759830, -13.29754803565872123 ) ) ;
#38332=CARTESIAN_POINT ( 'NONE',  ( 31.06344462049394295, -14.71666030541080161, -11.98151952013437693 ) ) ;
#38341=CARTESIAN_POINT ( 'NONE',  ( -1.842295339504430807, 36.47303149705159342, -9.727466432712501998 ) ) ;
#38348=CARTESIAN_POINT ( 'NONE',  ( 12.48692422165860094, 25.74591318921861927, -14.24962641246380457 ) ) ;
#38351=CARTESIAN_POINT ( 'NONE',  ( -19.60099714212322297, 15.55874775609486882, -7.421013871162296383 ) ) ;
#38354=CARTESIAN_POINT ( 'NONE',  ( 9.825092482715485076, -18.54622831478960165, -26.22104406996453108 ) ) ;
#38357=CARTESIAN_POINT ( 'NONE',  ( 15.08290252549542920, 26.19981407040120658, -8.764898325908280441 ) ) ;
#38358=CARTESIAN_POINT ( 'NONE',  ( -22.40982762235196191, 2.618079236897031148, -29.99999999999999645 ) ) ;
#38361=CARTESIAN_POINT ( 'NONE',  ( -25.88768482325948028, -24.33645162349362678, -9.343698090164346937 ) ) ;
#38362=CARTESIAN_POINT ( 'NONE',  ( 7.456069066676004553, -20.04449398788877090, -24.14870290390329188 ) ) ;
#38363=CARTESIAN_POINT ( 'NONE',  ( 11.78620804298909519, 18.81532866151945171, -22.75140267569650021 ) ) ;
#38364=CARTESIAN_POINT ( 'NONE',  ( 16.93799999173078419, 12.15640281848874871, -25.49561531272128789 ) ) ;
#38368=CARTESIAN_POINT ( 'NONE',  ( -8.386326804491467612, 35.75291558016277094, -7.156120314017831774 ) ) ;
#38370=CARTESIAN_POINT ( 'NONE',  ( -14.59943873959954352, -25.62395699127592508, -10.18321298866148972 ) ) ;
#38374=CARTESIAN_POINT ( 'NONE',  ( 22.22387256208718043, 0.6525034796978533835, -22.73371951963157400 ) ) ;
#38379=CARTESIAN_POINT ( 'NONE',  ( -25.16170031353656356, 0.4714222071989471741, -17.44778650913232099 ) ) ;
#38381=CARTESIAN_POINT ( 'NONE',  ( 23.39873936915197916, -6.309811595435544263, -20.90194788542293125 ) ) ;
#38396=CARTESIAN_POINT ( 'NONE',  ( 19.03553521139049209, 16.91159591655264904, -6.445528870334666927 ) ) ;
#38397=CARTESIAN_POINT ( 'NONE',  ( 10.34309936930504925, 32.23458342254649978, -10.30124509090378915 ) ) ;
#38401=CARTESIAN_POINT ( 'NONE',  ( 9.937768194491171769, -17.93102150851172993, -29.33920091550964671 ) ) ;
#38405=ORIENTED_EDGE ( 'NONE', *, *, #13311, .F. ) ;
#38406=CARTESIAN_POINT ( 'NONE',  ( -11.19011939127313049, 17.75217256258857645, -26.22551013601530912 ) ) ;
#38408=CARTESIAN_POINT ( 'NONE',  ( 11.48325201437814158, -21.51848809436486931, -18.49319478269642403 ) ) ;
#38415=CARTESIAN_POINT ( 'NONE',  ( -9.138473067724239840, 20.98330350826042690, -22.34731987422578570 ) ) ;
#38420=CARTESIAN_POINT ( 'NONE',  ( -24.34759780290428566, -6.015430600026174801, -19.86655231846714287 ) ) ;
#38423=CARTESIAN_POINT ( 'NONE',  ( 23.27325054855478470, 0.6741572905409627392, -20.55679979627661425 ) ) ;
#38424=CARTESIAN_POINT ( 'NONE',  ( 15.11440468493446687, 26.16449293604169668, -8.767649845972018241 ) ) ;
#38428=CARTESIAN_POINT ( 'NONE',  ( -29.36168537595271744, 0.06585758006631414752, -10.65324670958523967 ) ) ;
#38431=CARTESIAN_POINT ( 'NONE',  ( 20.88446507122673168, -1.639503378383732279, -26.63968719893129133 ) ) ;
#38448=CARTESIAN_POINT ( 'NONE',  ( -19.30322778826291596, 7.114745259177782444, -28.27681454190587473 ) ) ;
#38449=CARTESIAN_POINT ( 'NONE',  ( 21.77381489986708729, -26.82402092198213950, -7.223031671328368652 ) ) ;
#38452=CARTESIAN_POINT ( 'NONE',  ( 10.98290474487089341, 17.71099146112738154, -26.81703527214839156 ) ) ;
#38454=CARTESIAN_POINT ( 'NONE',  ( -12.17818915529227475, 17.82757546800293724, -23.95589322833938084 ) ) ;
#38458=CARTESIAN_POINT ( 'NONE',  ( 11.93447970895564936, 19.33730221226423396, -21.62440255458760774 ) ) ;
#38460=CARTESIAN_POINT ( 'NONE',  ( 33.12547343259578980, -19.59933603596603291, -5.855473759911283160 ) ) ;
#38463=CARTESIAN_POINT ( 'NONE',  ( -14.09052875053176024, 24.98470579825722027, -12.50744983255499676 ) ) ;
#38465=CARTESIAN_POINT ( 'NONE',  ( -9.913802546424228979, -17.94660116923212456, -29.33974538417603384 ) ) ;
#38469=CARTESIAN_POINT ( 'NONE',  ( -25.62699182077987814, -10.58736709928222197, -17.64213997670373146 ) ) ;
#38470=CARTESIAN_POINT ( 'NONE',  ( -9.194505705513583038, -18.37015698959482890, -28.71945744372206022 ) ) ;
#38472=CARTESIAN_POINT ( 'NONE',  ( 16.90293753726015780, 20.49095762985944447, -9.799744462339120332 ) ) ;
#38474=CARTESIAN_POINT ( 'NONE',  ( 27.37006007402764496, 2.900043331923816581, -9.768361963922430391 ) ) ;
#38479=CARTESIAN_POINT ( 'NONE',  ( -20.49112616741955506, 0.6095660351776280850, -29.34380360967770685 ) ) ;
#38480=CARTESIAN_POINT ( 'NONE',  ( 30.22309925524323759, -0.6771996511655676843, -10.12731539925492541 ) ) ;
#38483=CARTESIAN_POINT ( 'NONE',  ( -28.28304003931276966, 1.770888965579145324, -9.744255481737679858 ) ) ;
#38484=CARTESIAN_POINT ( 'NONE',  ( -23.06249103411543544, 13.31513540672989926, -13.39439507595155554 ) ) ;
#38496=CARTESIAN_POINT ( 'NONE',  ( 22.40086744732950308, -20.72561197270982447, -14.82888506793862859 ) ) ;
#38499=CARTESIAN_POINT ( 'NONE',  ( 15.18041152575273500, 27.55477496851653640, -5.470520559687252593 ) ) ;
#38502=AXIS2_PLACEMENT_3D ( 'NONE', #27395, #11368, #39786 ) ;
#38503=CARTESIAN_POINT ( 'NONE',  ( -14.43025776552523709, 14.57938852240508965, -30.00000000000000711 ) ) ;
#38505=CARTESIAN_POINT ( 'NONE',  ( 9.439680310844765998, -18.19733056428809803, -30.00000000000000000 ) ) ;
#38507=CARTESIAN_POINT ( 'NONE',  ( 11.19190749613552072, 17.75087991604564053, -26.22569030697802717 ) ) ;
#38509=CARTESIAN_POINT ( 'NONE',  ( 11.88987759224297669, 19.38458514940646893, -21.61667515872348133 ) ) ;
#38511=CARTESIAN_POINT ( 'NONE',  ( -15.19914089571920890, 26.51953392815337196, -7.824019997130747583 ) ) ;
#38513=CARTESIAN_POINT ( 'NONE',  ( -13.34033674645691647, -23.61967562324617731, -14.47800511745506213 ) ) ;
#38515=CARTESIAN_POINT ( 'NONE',  ( -31.30459858316601185, -18.91178069307321152, -9.725088435557024624 ) ) ;
#38516=VECTOR ( 'NONE', #21405, 1000.000000000000000 ) ;
#38517=CARTESIAN_POINT ( 'NONE',  ( -7.194050238941392728, -21.51981635923818104, -19.89556854701389099 ) ) ;
#38518=CARTESIAN_POINT ( 'NONE',  ( 13.13555678008467353, 20.35422080500006459, -18.53327313025195977 ) ) ;
#38520=CARTESIAN_POINT ( 'NONE',  ( 23.60508491000810594, 8.220972298804724687, -9.371835443833486323 ) ) ;
#38522=CARTESIAN_POINT ( 'NONE',  ( 12.74984837297361828, -26.03613044200378113, -5.000000000000000000 ) ) ;
#38525=CARTESIAN_POINT ( 'NONE',  ( -26.24583311168948185, -1.798973365801582291, -17.17928807732686280 ) ) ;
#38529=DIRECTION ( 'NONE',  ( -0.000000000000000000, -0.000000000000000000, -1.000000000000000000 ) ) ;
#38532=CARTESIAN_POINT ( 'NONE',  ( 33.19857134126652909, -14.52248378749990820, -9.739578698604827167 ) ) ;
#38544=CARTESIAN_POINT ( 'NONE',  ( -0.7332251858107181608, 37.19956836493663843, -8.842669820069614772 ) ) ;
#38551=CARTESIAN_POINT ( 'NONE',  ( 11.54610483293918755, 23.61922780243806486, -17.18207871116365837 ) ) ;
#38554=CARTESIAN_POINT ( 'NONE',  ( -19.24418432356083386, 12.60524799736691115, -15.94388489509767837 ) ) ;
#38557=CARTESIAN_POINT ( 'NONE',  ( 14.06819841691203266, -24.61544153353286646, -12.54891093376155986 ) ) ;
#38559=CARTESIAN_POINT ( 'NONE',  ( 14.72345531851253853, 25.43898799495751106, -10.65037270653031598 ) ) ;
#38560=CARTESIAN_POINT ( 'NONE',  ( -6.155076441694329326, 21.71698211341365692, -29.99999999999997868 ) ) ;
#38562=CIRCLE ( 'NONE', #37289, 18.00000000000000355 ) ;
#38563=CARTESIAN_POINT ( 'NONE',  ( -26.29711927695796092, -24.70225483488810170, -8.459928924156699281 ) ) ;
#38564=CARTESIAN_POINT ( 'NONE',  ( 8.347004892849424706, -25.02468466642049449, -8.361640715383630962 ) ) ;
#38565=CARTESIAN_POINT ( 'NONE',  ( 11.14613432397584880, 17.25733169733589989, -28.71274769282841888 ) ) ;
#38566=CARTESIAN_POINT ( 'NONE',  ( 17.21149163973099760, 11.38646518709530220, -27.17255296939820752 ) ) ;
#38571=ORIENTED_EDGE ( 'NONE', *, *, #25247, .T. ) ;
#38572=CARTESIAN_POINT ( 'NONE',  ( -7.326431115582969333, 35.94962014070476641, -8.009053875344944728 ) ) ;
#38574=CARTESIAN_POINT ( 'NONE',  ( -15.09037123163817640, -26.35566568629046103, -7.828641914250869860 ) ) ;
#38579=ORIENTED_EDGE ( 'NONE', *, *, #35196, .F. ) ;
#38580=CARTESIAN_POINT ( 'NONE',  ( -20.80888993467136316, 0.9087143968972012376, -26.83659548020632002 ) ) ;
#38582=CARTESIAN_POINT ( 'NONE',  ( 34.50741919436119787, -9.298902886619249131, -8.474956792276689299 ) ) ;
#38588=DIRECTION ( 'NONE',  ( -1.000000000000000000, 0.000000000000000000, 0.000000000000000000 ) ) ;
#38594=DIRECTION ( 'NONE',  ( 0.000000000000000000, 0.000000000000000000, 1.000000000000000000 ) ) ;
#38597=CARTESIAN_POINT ( 'NONE',  ( 15.53294352554807034, 13.99868018475545561, -25.43220508911406341 ) ) ;
#38598=CARTESIAN_POINT ( 'NONE',  ( 6.888886835531742747, 21.38082869974457623, -23.27631121293514838 ) ) ;
#38602=CARTESIAN_POINT ( 'NONE',  ( 10.11113855348066615, -17.88931650804065754, -28.68331442007524856 ) ) ;
#38603=DIRECTION ( 'NONE',  ( -1.000000000000000000, 0.000000000000000000, 0.000000000000000000 ) ) ;
#38607=CARTESIAN_POINT ( 'NONE',  ( -11.06212937511586958, 17.50982107800345133, -27.44695155360371075 ) ) ;
#38609=CARTESIAN_POINT ( 'NONE',  ( 14.79195119394937308, -26.44684019677998421, -6.889201696584072110 ) ) ;
#38615=CARTESIAN_POINT ( 'NONE',  ( -11.87470576980882697, 27.72462808436429071, -13.19994123200545744 ) ) ;
#38616=AXIS2_PLACEMENT_3D ( 'NONE', #34864, #16782, #29168 ) ;
#38620=CARTESIAN_POINT ( 'NONE',  ( -26.22468522521110046, -6.472231845536984274, -17.80872549056464749 ) ) ;
#38624=CARTESIAN_POINT ( 'NONE',  ( 21.25435618972812790, 0.9309806893528798089, -25.03105100026559171 ) ) ;
#38629=CARTESIAN_POINT ( 'NONE',  ( -26.50930299955345504, 0.2689666410773219885, -15.44989252601773266 ) ) ;
#38633=CARTESIAN_POINT ( 'NONE',  ( 28.04465044637506921, -2.531702322499061353, -15.16146178204541073 ) ) ;
#38646=CIRCLE ( 'NONE', #16610, 17.00000000000000355 ) ;
#38647=CARTESIAN_POINT ( 'NONE',  ( 4.861068763497363499, 36.44255459974750266, -8.860485891349553000 ) ) ;
#38651=CARTESIAN_POINT ( 'NONE',  ( -20.92786251698451494, 10.22285104615988693, -14.91617428519021082 ) ) ;
#38652=CARTESIAN_POINT ( 'NONE',  ( 21.40359050063177904, -26.41076042838597004, -8.557087298424924882 ) ) ;
#38656=CARTESIAN_POINT ( 'NONE',  ( 15.38842093998857230, 26.88136989284191003, -5.473725555427078504 ) ) ;
#38658=CARTESIAN_POINT ( 'NONE',  ( -15.63977754581427959, 25.75093463275924677, -6.418238443301547136 ) ) ;
#38661=CARTESIAN_POINT ( 'NONE',  ( 15.26439360241955612, 26.29740473991443039, -7.828362627414925612 ) ) ;
#38663=CARTESIAN_POINT ( 'NONE',  ( 30.18950977129052049, -16.64208564415852365, -11.97445339315004809 ) ) ;
#38665=CARTESIAN_POINT ( 'NONE',  ( -13.86789451117665095, 24.32149117241265301, -13.47705164427899938 ) ) ;
#38668=CARTESIAN_POINT ( 'NONE',  ( -9.941839879247096334, -17.98565085000458197, -28.69025900671589824 ) ) ;
#38672=CARTESIAN_POINT ( 'NONE',  ( -27.67975872713484975, -11.41987064963364062, -15.71665464447120186 ) ) ;
#38673=CARTESIAN_POINT ( 'NONE',  ( -9.133854131406611288, -18.57253604913642420, -27.48140049201442636 ) ) ;
#38675=CARTESIAN_POINT ( 'NONE',  ( 15.09486127709339875, 17.52762106458872893, -18.81276594169348471 ) ) ;
#38677=CARTESIAN_POINT ( 'NONE',  ( 26.02691584061487973, 3.766903892757499595, -11.72995947271240524 ) ) ;
#38682=CARTESIAN_POINT ( 'NONE',  ( -20.82975236705524580, 0.6559526755414205601, -26.81703596920652544 ) ) ;
#38683=CARTESIAN_POINT ( 'NONE',  ( 23.42995061493359543, 0.2370758946468835837, -20.49876334635902353 ) ) ;
#38689=CARTESIAN_POINT ( 'NONE',  ( -27.03853842261034046, 1.817756925060996176, -12.62724191157268194 ) ) ;
#38690=CARTESIAN_POINT ( 'NONE',  ( -16.84920187454418539, 29.09530251867925443, -5.000000000000000000 ) ) ;
#38702=CARTESIAN_POINT ( 'NONE',  ( 16.15654479250856213, -14.01367662916781143, -25.66150427861421690 ) ) ;
#38705=CARTESIAN_POINT ( 'NONE',  ( 11.39958526853898668, 19.89188415871232252, -21.52512903687211221 ) ) ;
#38708=CARTESIAN_POINT ( 'NONE',  ( -17.41140981635742691, 20.80174530708337244, -5.000000000000000000 ) ) ;
#38711=CARTESIAN_POINT ( 'NONE',  ( 12.59484304515129516, -22.55689553818449156, -16.44840651353704786 ) ) ;
#38713=CARTESIAN_POINT ( 'NONE',  ( 10.99531269100861763, 17.30182433700542788, -30.00000000000001421 ) ) ;
#38715=CARTESIAN_POINT ( 'NONE',  ( 14.93529390890679664, 25.79829262747109198, -9.709001792061677349 ) ) ;
#38717=CARTESIAN_POINT ( 'NONE',  ( -14.71284311239260667, 25.47114600920629002, -10.64827379499097226 ) ) ;
#38720=CARTESIAN_POINT ( 'NONE',  ( -15.31510379003943356, -26.50301315550676762, -7.358184284617420801 ) ) ;
#38722=EDGE_CURVE ( 'NONE', #23375, #19728, #4688, .T. ) ;
#38723=CARTESIAN_POINT ( 'NONE',  ( -27.21050208389111447, -17.59196774493118198, -13.80967687889205919 ) ) ;
#38724=CARTESIAN_POINT ( 'NONE',  ( -4.980521078259840806, -20.55575703614546512, -24.29636214656850868 ) ) ;
#38725=CARTESIAN_POINT ( 'NONE',  ( 15.93428740759538265, 25.01899822204553203, -5.000000000000000888 ) ) ;
#38727=CARTESIAN_POINT ( 'NONE',  ( 20.37439232564474523, 8.397279452178770143, -20.08687019429353882 ) ) ;
#38728=LINE ( 'NONE', #20247, #17378 ) ;
#38732=CARTESIAN_POINT ( 'NONE',  ( -20.71492070759099136, -1.809969325171036481, -27.27634564961995878 ) ) ;
#38738=CARTESIAN_POINT ( 'NONE',  ( 19.88015388149283780, -9.459153964528258740, -24.23427547882557320 ) ) ;
#38747=CARTESIAN_POINT ( 'NONE',  ( 1.146085828710420085, 27.91706644536319359, -17.59780091161095328 ) ) ;
#38749=CARTESIAN_POINT ( 'NONE',  ( -75.15099915297791711, 43.38844959084113384, -5.000000000000000000 ) ) ;
#38753=CARTESIAN_POINT ( 'NONE',  ( 10.34603125738301266, 20.85552122335373681, -21.35002345354203968 ) ) ;
#38756=CARTESIAN_POINT ( 'NONE',  ( -17.23503577783534624, 11.12556197759191967, -30.00000000000000000 ) ) ;
#38759=CARTESIAN_POINT ( 'NONE',  ( 11.57930096821026744, -20.97270239393662550, -19.49257125052969641 ) ) ;
#38761=CARTESIAN_POINT ( 'NONE',  ( 14.00631563109706512, 23.99234777561873599, -13.50787202288133848 ) ) ;
#38762=CARTESIAN_POINT ( 'NONE',  ( -21.88444403592365362, 6.126538576424530369, -30.00000000000001066 ) ) ;
#38766=CARTESIAN_POINT ( 'NONE',  ( -28.02256666113110128, -24.77408825670562820, -5.866844285589661645 ) ) ;
#38767=CARTESIAN_POINT ( 'NONE',  ( 3.780512468825520056, -23.99670114915234720, -11.86248818774162572 ) ) ;
#38768=CARTESIAN_POINT ( 'NONE',  ( 15.39800120669520389, 26.16141782975133623, -7.359158868726225045 ) ) ;
#38769=CARTESIAN_POINT ( 'NONE',  ( 20.90635927389905291, 12.88005819179653599, -8.408867834709406353 ) ) ;
#38773=CARTESIAN_POINT ( 'NONE',  ( -6.922216865142736708, 33.79108910511520492, -11.11993846343762016 ) ) ;
#38783=CARTESIAN_POINT ( 'NONE',  ( -23.89935431336828842, 0.5844314413813609388, -19.50775400706428897 ) ) ;
#38785=CARTESIAN_POINT ( 'NONE',  ( 23.29525806319241710, -7.038873791111292633, -20.85594693144456357 ) ) ;
#38796=ORIENTED_EDGE ( 'NONE', *, *, #21993, .F. ) ;
#38797=CARTESIAN_POINT ( 'NONE',  ( -19.48557158514998022, -11.24999999999982414, 3.000000000000000000 ) ) ;
#38801=CARTESIAN_POINT ( 'NONE',  ( 18.72104006414143029, 16.54790594782236113, -9.860094852877404392 ) ) ;
#38803=CARTESIAN_POINT ( 'NONE',  ( 9.917373875393378668, 30.84216450598692916, -12.12503220460585851 ) ) ;
#38807=CARTESIAN_POINT ( 'NONE',  ( 11.18272573551269566, -19.90824572261553271, -21.57092338806107179 ) ) ;
#38808=CARTESIAN_POINT ( 'NONE',  ( 37.48507449946188785, -12.38247117345842341, -5.000000000000004441 ) ) ;
#38811=CARTESIAN_POINT ( 'NONE',  ( -14.73694251361284913, 25.39790523529706334, -10.65305906957618021 ) ) ;
#38813=CARTESIAN_POINT ( 'NONE',  ( 14.29043209799990777, -26.44292502402198863, -5.000000000000000888 ) ) ;
#38817=ORIENTED_EDGE ( 'NONE', *, *, #33101, .T. ) ;
#38818=CARTESIAN_POINT ( 'NONE',  ( -9.053254851683428583, 24.89655747824621201, -17.93160491756381347 ) ) ;
#38822=CARTESIAN_POINT ( 'NONE',  ( -20.80768648429576473, -4.462460184070209834, -25.80116617916775823 ) ) ;
#38823=CARTESIAN_POINT ( 'NONE',  ( 15.48853125999100833, -26.74269726803731118, -0.000000000000000000 ) ) ;
#38825=CARTESIAN_POINT ( 'NONE',  ( 20.96220882709428324, 0.8789131500063240843, -26.23105454971878459 ) ) ;
#38827=CARTESIAN_POINT ( 'NONE',  ( -12.27050296327057666, -16.73575495843078187, -27.23024630153084402 ) ) ;
#38828=CARTESIAN_POINT ( 'NONE',  ( 32.33143948541783885, 1.358872982501748927, -5.000000000000000000 ) ) ;
#38833=CARTESIAN_POINT ( 'NONE',  ( -25.21380665299743740, 0.3741287532325562881, -17.43820136744484017 ) ) ;
#38836=CARTESIAN_POINT ( 'NONE',  ( 31.81590626430815050, -2.991356775276182489, -9.994954404607028664 ) ) ;
#38850=CARTESIAN_POINT ( 'NONE',  ( 4.739855970000743213, 35.45921866945190004, -10.19245697289364649 ) ) ;
#38854=CARTESIAN_POINT ( 'NONE',  ( 11.84905944520939158, -16.93912730843665315, -27.94593565603549123 ) ) ;
#38860=CARTESIAN_POINT ( 'NONE',  ( 13.16052575310691175, 22.32601956860930059, -16.43275809617471239 ) ) ;
#38861=ORIENTED_EDGE ( 'NONE', *, *, #6394, .T. ) ;
#38862=CARTESIAN_POINT ( 'NONE',  ( -15.36331629305222535, 25.66072101725646348, -8.302433069061233795 ) ) ;
#38865=CARTESIAN_POINT ( 'NONE',  ( 15.44105900787717900, 26.60157864969849228, -5.946102268273840252 ) ) ;
#38867=CARTESIAN_POINT ( 'NONE',  ( 17.40478573504346471, -11.01252481820737117, -28.44515566755788072 ) ) ;
#38869=CARTESIAN_POINT ( 'NONE',  ( -15.17875652326131863, 27.47441271400335694, -5.938670991771770602 ) ) ;
#38871=CARTESIAN_POINT ( 'NONE',  ( -16.58921006345730120, -26.12567795957870942, -9.624075946779614199 ) ) ;
#38875=CARTESIAN_POINT ( 'NONE',  ( -32.35609090632282658, -13.32965902131102709, -11.08975651091474468 ) ) ;
#38876=CARTESIAN_POINT ( 'NONE',  ( -10.52791161976172596, -20.06334676836660336, -21.65469227164354038 ) ) ;
#38878=CARTESIAN_POINT ( 'NONE',  ( 15.29136776227527150, 19.45896063891741079, -15.68350118317069608 ) ) ;
#38880=CARTESIAN_POINT ( 'NONE',  ( 21.44184074642562976, 4.518366863407804246, -22.01530538004446669 ) ) ;
#38882=CARTESIAN_POINT ( 'NONE',  ( 36.48557158514975640, -11.24999999999995559, 6.000000000000000000 ) ) ;
#38884=CARTESIAN_POINT ( 'NONE',  ( -20.71012148218438043, 0.5861083848712056454, -27.43142461003399291 ) ) ;
#38886=CARTESIAN_POINT ( 'NONE',  ( 22.87208170588712264, 0.1283377855311399196, -21.55196105168392151 ) ) ;
#38890=CARTESIAN_POINT ( 'NONE',  ( -20.49897829065735166, 2.206463918494783627, -28.14064370775090751 ) ) ;
#38892=CARTESIAN_POINT ( 'NONE',  ( -33.62187204924172335, 0.04418559750806001774, -13.79123840944734347 ) ) ;
#38900=CARTESIAN_POINT ( 'NONE',  ( -25.77311405540110911, 5.286159686137065883, -8.844531936936238736 ) ) ;
#38903=CARTESIAN_POINT ( 'NONE',  ( 28.35230428231212230, -24.61827297795788638, -5.000000000000000000 ) ) ;
#38906=CARTESIAN_POINT ( 'NONE',  ( 10.90819920133987964, 17.95289977334026688, -26.19501740155092406 ) ) ;
#38909=CARTESIAN_POINT ( 'NONE',  ( -13.94411147149912367, 15.13589321949257460, -28.21918225953774240 ) ) ;
#38911=CARTESIAN_POINT ( 'NONE',  ( 9.458291886585664443, -18.18766449894053849, -29.34916192869308560 ) ) ;
#38913=CARTESIAN_POINT ( 'NONE',  ( 14.30088122820257368, 24.44632208664130246, -12.55129266994459059 ) ) ;
#38917=CARTESIAN_POINT ( 'NONE',  ( -11.24611422795147853, 18.08780201161743406, -25.00577628530580299 ) ) ;
#38919=CARTESIAN_POINT ( 'NONE',  ( -11.24122759046548481, -20.45868835281356723, -20.53405996523489563 ) ) ;
#38922=CARTESIAN_POINT ( 'NONE',  ( -32.77147431096915398, -19.79161752149877174, -6.696281051292849895 ) ) ;
#38923=CARTESIAN_POINT ( 'NONE',  ( -6.072675937371057486, -22.95838016832008677, -15.82819075888657068 ) ) ;
#38924=CARTESIAN_POINT ( 'NONE',  ( 15.67293563814069124, 24.96974998548517277, -7.836397927719035650 ) ) ;
#38927=CARTESIAN_POINT ( 'NONE',  ( 23.77017115979666428, 8.255607362891254297, -8.390682868101873026 ) ) ;
#38929=DIRECTION ( 'NONE',  ( 1.000000000000000000, 0.000000000000000000, 0.000000000000000000 ) ) ;
#38932=CARTESIAN_POINT ( 'NONE',  ( -31.69715058011894016, -2.389216380787061222, -9.565402919442236751 ) ) ;
#38938=CARTESIAN_POINT ( 'NONE',  ( 18.59608826487667343, -8.852250640322028019, -28.44979860309804920 ) ) ;
#38939=DIRECTION ( 'NONE',  ( -1.000000000000000000, 0.000000000000000000, 0.000000000000000000 ) ) ;
#38946=ADVANCED_FACE ( 'NONE', ( #14552 ), #39333, .T. ) ;
#38949=CARTESIAN_POINT ( 'NONE',  ( 1.565334152085329888, 38.07008842306128571, -7.117895202388205611 ) ) ;
#38955=CARTESIAN_POINT ( 'NONE',  ( 11.69402330146858482, 21.36632422587266689, -19.35895708507096202 ) ) ;
#38959=CARTESIAN_POINT ( 'NONE',  ( -18.76357486801690655, 13.43274215842698993, -15.92991587464894288 ) ) ;
#38962=CARTESIAN_POINT ( 'NONE',  ( 14.39131927975945402, -25.07688395697384465, -11.59674742285950089 ) ) ;
#38964=CARTESIAN_POINT ( 'NONE',  ( 11.66333929151196713, 18.93342404723955852, -22.73119902039520568 ) ) ;
#38965=CARTESIAN_POINT ( 'NONE',  ( 11.31392148919590923, 36.91540483778863546, -5.000000000000002665 ) ) ;
#38968=CARTESIAN_POINT ( 'NONE',  ( -15.43503188818483451, -13.62775707822376070, -28.48261797098671266 ) ) ;
#38969=CARTESIAN_POINT ( 'NONE',  ( 4.192399910511806382, -20.06660217949758618, -30.00000000000001776 ) ) ;
#38970=CARTESIAN_POINT ( 'NONE',  ( 11.16317946027923824, 17.19403390828999889, -30.00000000000000355 ) ) ;
#38972=CARTESIAN_POINT ( 'NONE',  ( 20.85031025169343266, 12.84359668456042591, -8.901149520029621343 ) ) ;
#38976=CARTESIAN_POINT ( 'NONE',  ( -7.236536542773612801, 35.44204148769340179, -8.885907059458707735 ) ) ;
#38983=CARTESIAN_POINT ( 'NONE',  ( -24.49105222923185821, 0.5749155098870283309, -18.46773377504650782 ) ) ;
#38985=CARTESIAN_POINT ( 'NONE',  ( 34.58134563245810256, -10.42100876475338467, -8.458827757296450756 ) ) ;
#39000=CARTESIAN_POINT ( 'NONE',  ( 18.25029525998795066, 16.00669453228446670, -12.84108188352884206 ) ) ;
#39001=CARTESIAN_POINT ( 'NONE',  ( 7.669720458042128541, 19.54291380638433040, -26.53555194593364064 ) ) ;
#39005=CARTESIAN_POINT ( 'NONE',  ( 14.28460229709901519, -24.65033995194861660, -12.53151620945226341 ) ) ;
#39006=CARTESIAN_POINT ( 'NONE',  ( 20.55563217186196212, -29.52600041847795254, -5.000000000000018652 ) ) ;
#39008=CARTESIAN_POINT ( 'NONE',  ( -12.38581555130674872, 20.49744764627239491, -19.49524353550787126 ) ) ;
#39010=CARTESIAN_POINT ( 'NONE',  ( 8.962294377823376124, -18.56986243642861112, -28.10993916399811354 ) ) ;
#39015=CARTESIAN_POINT ( 'NONE',  ( -11.29360755245008718, 31.24910176029843711, -10.34195632950957844 ) ) ;
#39018=CARTESIAN_POINT ( 'NONE',  ( -21.37767459502805778, -3.913953112044378457, -24.54261330738080460 ) ) ;
#39021=CARTESIAN_POINT ( 'NONE',  ( 30.26282733560709559, 0.09093532349598118514, -8.298613290467722337 ) ) ;
#39027=CARTESIAN_POINT ( 'NONE',  ( -20.48192033757745278, 0.8608427067432725677, -30.00000000000000000 ) ) ;
#39030=CARTESIAN_POINT ( 'NONE',  ( 29.94967456567781028, -3.579765429977533220, -13.19994935436286809 ) ) ;
#39043=CARTESIAN_POINT ( 'NONE',  ( 2.701375607076830221, 20.57380448486020086, -27.72792284495386994 ) ) ;
#39044=CARTESIAN_POINT ( 'NONE',  ( 28.79410123593972415, 4.962698632456642223, -5.000000000000000000 ) ) ;
#39049=CARTESIAN_POINT ( 'NONE',  ( 12.97325122237492145, -17.30183730846044554, -24.66100610027864093 ) ) ;
#39054=CARTESIAN_POINT ( 'NONE',  ( 13.97401297928019481, 24.07084740764522124, -13.50045613746490325 ) ) ;
#39056=CARTESIAN_POINT ( 'NONE',  ( -11.43474607271607724, 17.01453699462772207, -29.35782462692642625 ) ) ;
#39059=CARTESIAN_POINT ( 'NONE',  ( 15.04605592278479875, 25.88023467481654905, -9.239420567519900374 ) ) ;
#39061=CARTESIAN_POINT ( 'NONE',  ( 29.70373973584631955, -17.57897857355148830, -11.97277981779456901 ) ) ;
#39063=CARTESIAN_POINT ( 'NONE',  ( -12.97748996312875747, 22.65302653440283009, -16.39225588091346353 ) ) ;
#39065=CARTESIAN_POINT ( 'NONE',  ( -11.66758301494133043, -19.21216028216936422, -22.58759682042235184 ) ) ;
#39068=CARTESIAN_POINT ( 'NONE',  ( -31.87840698781867133, -10.92544140939488173, -12.02591668823370874 ) ) ;
#39069=CARTESIAN_POINT ( 'NONE',  ( -12.15224344198015949, -22.55312021461349303, -16.48165687185815642 ) ) ;
#39070=AXIS2_PLACEMENT_3D ( 'NONE', #30767, #27702, #15522 ) ;
#39073=CARTESIAN_POINT ( 'NONE',  ( 21.18854743806299368, 3.064997187841227877, -24.09357946227068936 ) ) ;
#39079=CARTESIAN_POINT ( 'NONE',  ( -22.26224525938009435, 0.4962469403767001963, -22.71332818809632670 ) ) ;
#39080=CARTESIAN_POINT ( 'NONE',  ( 22.37143894708468395, 0.01545002306387475294, -22.65172220279661275 ) ) ;
#39084=CARTESIAN_POINT ( 'NONE',  ( -22.03994032835833750, 1.381754348432899349, -22.81883089661271669 ) ) ;
#39085=CARTESIAN_POINT ( 'NONE',  ( 11.10756861982301125, 19.59949212537556562, -30.00000000000000000 ) ) ;
#39086=DIRECTION ( 'NONE',  ( 0.000000000000000000, 0.000000000000000000, -1.000000000000000000 ) ) ;
#39094=CARTESIAN_POINT ( 'NONE',  ( -20.36895863172275156, 5.751155262373932153, -24.28491833738754835 ) ) ;
#39097=CARTESIAN_POINT ( 'NONE',  ( 17.32694539406390177, -16.96442657344122296, -20.89054752054989805 ) ) ;
#39099=CARTESIAN_POINT ( 'NONE',  ( 10.72215843559913750, 17.73370681071187605, -27.42052473872761098 ) ) ;
#39103=CARTESIAN_POINT ( 'NONE',  ( -15.20072915685657122, 20.47391248462032465, -14.64817096683644593 ) ) ;
#39107=CARTESIAN_POINT ( 'NONE',  ( 14.74653517655818291, 25.36980923495725548, -10.65380407947966823 ) ) ;
#39111=CARTESIAN_POINT ( 'NONE',  ( -14.69323628723109998, 25.52969830242819427, -10.64447204089981014 ) ) ;
#39112=LINE ( 'NONE', #27325, #30276 ) ;
#39113=CARTESIAN_POINT ( 'NONE',  ( -15.57263558642642032, -26.76429566359157164, -5.000000000000000888 ) ) ;
#39116=CARTESIAN_POINT ( 'NONE',  ( -30.97886774876783633, -18.71541742275284648, -10.17228780496799878 ) ) ;
#39117=CARTESIAN_POINT ( 'NONE',  ( -6.137033441707241188, -19.64448462102270909, -28.81001259779947077 ) ) ;
#39118=CARTESIAN_POINT ( 'NONE',  ( 13.39920212058827964, 20.89892004213690768, -17.51356503033543888 ) ) ;
#39120=CARTESIAN_POINT ( 'NONE',  ( 24.66102986608180103, 7.389241230280822137, -5.000000000000000888 ) ) ;
#39126=CARTESIAN_POINT ( 'NONE',  ( -32.30815150485408793, -1.680769291408187538, -5.465098400837421266 ) ) ;
#39128=CARTESIAN_POINT ( 'NONE',  ( 24.56621758168594738, 0.4171823343055403588, -18.45072505565352472 ) ) ;
#39142=CARTESIAN_POINT ( 'NONE',  ( 0.8699709723833062291, 21.42695088328918018, -25.57864724691659930 ) ) ;
#39149=CARTESIAN_POINT ( 'NONE',  ( 12.04999115871534876, 22.98224508480782902, -17.26137212625882000 ) ) ;
#39153=CARTESIAN_POINT ( 'NONE',  ( -18.19708040568177410, 15.52697327766063218, -13.86016582398509556 ) ) ;
#39157=CARTESIAN_POINT ( 'NONE',  ( 15.50471485482113820, -26.74686345152265332, -5.000000000000000888 ) ) ;
#39159=CARTESIAN_POINT ( 'NONE',  ( 15.32564493454926513, 26.66194327151340815, -6.887025365065524873 ) ) ;
#39160=CARTESIAN_POINT ( 'NONE',  ( 11.10756861982301125, 19.59949212537556562, -30.00000000000000000 ) ) ;
#39163=CARTESIAN_POINT ( 'NONE',  ( -26.61378535533439305, -24.97840923415078862, -7.589850937743148229 ) ) ;
#39164=CARTESIAN_POINT ( 'NONE',  ( 3.837299910079773557, -24.19987090832864496, -10.86751699812955962 ) ) ;
#39165=CARTESIAN_POINT ( 'NONE',  ( 11.16317946027923824, 17.19403390828999889, -29.35217987579671117 ) ) ;
#39166=CARTESIAN_POINT ( 'NONE',  ( 19.71714621942704326, 13.31983420865925005, -12.88265316112568293 ) ) ;
#39170=CARTESIAN_POINT ( 'NONE',  ( -6.146602377671369410, 30.05109521024887798, -14.81031381684638859 ) ) ;
#39178=CARTESIAN_POINT ( 'NONE',  ( -1.829593030691901284E-15, 22.50000000000001066, 3.000000000000000000 ) ) ;
#39180=CARTESIAN_POINT ( 'NONE',  ( -20.47628691903608811, 0.9865603022909629205, -29.35067870942681267 ) ) ;
#39182=CARTESIAN_POINT ( 'NONE',  ( 33.36650818028201826, -11.13369706517688407, -10.22289954697786030 ) ) ;
#39199=CARTESIAN_POINT ( 'NONE',  ( 15.33041871681650292, 15.00779217446572744, -23.19570158157604567 ) ) ;
#39200=CARTESIAN_POINT ( 'NONE',  ( 12.31217864997667810, 32.24565435429136073, -7.223754960023913263 ) ) ;
#39206=CARTESIAN_POINT ( 'NONE',  ( 15.68560287515114560, -26.71608784079017340, -6.412881614423534771 ) ) ;
#39209=CARTESIAN_POINT ( 'NONE',  ( -15.23129526741244533, 26.40958019939556323, -7.827668941241471501 ) ) ;
#39212=CARTESIAN_POINT ( 'NONE',  ( 13.07091773603987406, -25.33042880074001602, -10.21159384544662885 ) ) ;
#39216=CARTESIAN_POINT ( 'NONE',  ( -7.928368490687788928, 21.70034315306905981, -22.21406577488186684 ) ) ;
#39223=CARTESIAN_POINT ( 'NONE',  ( 30.73050688267034758, 0.03238439121148584815, -6.417084242708104291 ) ) ;
#39224=DIRECTION ( 'NONE',  ( 1.000000000000000000, 0.000000000000000000, 0.000000000000000000 ) ) ;
#39228=CARTESIAN_POINT ( 'NONE',  ( -20.69342229627120133, 0.8482707436503026388, -27.44844477688208073 ) ) ;
#39231=CARTESIAN_POINT ( 'NONE',  ( 28.60017629935383354, -4.227747798920739264, -15.04471679130755390 ) ) ;
#39232=AXIS2_PLACEMENT_3D ( 'NONE', #38797, #38594, #10768 ) ;
#39245=CARTESIAN_POINT ( 'NONE',  ( 5.880693269542113910, 30.13551902636890389, -14.80509325191231618 ) ) ;
#39248=CARTESIAN_POINT ( 'NONE',  ( 13.55783596901029853, -19.12971960218908762, -21.26853342772727729 ) ) ;
#39253=CARTESIAN_POINT ( 'NONE',  ( 14.68930050026369827, 25.54147410505130722, -10.64370694421165453 ) ) ;
#39256=CARTESIAN_POINT ( 'NONE',  ( -12.30634478552224031, 18.94025476089912985, -21.68721750851181085 ) ) ;
#39260=CARTESIAN_POINT ( 'NONE',  ( 15.37921949410162981, 26.47433205842913750, -6.888199520723817137 ) ) ;
#39262=CARTESIAN_POINT ( 'NONE',  ( 32.39246062267798010, -20.52362622975203266, -6.276506097946584539 ) ) ;
#39264=CARTESIAN_POINT ( 'NONE',  ( -11.86077688257339524, 20.24129428177698742, -20.48706616378117928 ) ) ;
#39266=CARTESIAN_POINT ( 'NONE',  ( -11.00841538111624551, -18.87725956289415308, -23.75370681038233656 ) ) ;
#39269=CARTESIAN_POINT ( 'NONE',  ( -33.61361311049479639, -12.67649022699521311, -9.755067238301116106 ) ) ;
#39270=CARTESIAN_POINT ( 'NONE',  ( -13.61052633586881555, -24.54839736670113837, -12.56630099801351719 ) ) ;
#39273=CARTESIAN_POINT ( 'NONE',  ( 28.82737146255313476, 2.000641240079708894, -6.895424389095080819 ) ) ;
#39279=CARTESIAN_POINT ( 'NONE',  ( -25.26188173616072419, 0.2875138470135812363, -17.42658750387904121 ) ) ;
#39280=CARTESIAN_POINT ( 'NONE',  ( 20.50011096633554786, 0.05624224123783994750, -30.00000000000000000 ) ) ;
#39283=CARTESIAN_POINT ( 'NONE',  ( -26.72686952400124483, 3.517128624037218820, -10.26466785145276717 ) ) ;
#39295=CARTESIAN_POINT ( 'NONE',  ( -26.18615939189180608, 5.309650895087318467, -5.955328271003301310 ) ) ;
#39299=CARTESIAN_POINT ( 'NONE',  ( 25.29206606878849328, -26.20377346906149185, -4.999999999999997335 ) ) ;
#39300=DIRECTION ( 'NONE',  ( -0.000000000000000000, -0.000000000000000000, -1.000000000000000000 ) ) ;
#39302=CARTESIAN_POINT ( 'NONE',  ( 13.01074387160668522, 22.59504030922215279, -16.39937294696464676 ) ) ;
#39305=CARTESIAN_POINT ( 'NONE',  ( -14.53441762336499998, 17.65377433136575647, -19.82464443782235008 ) ) ;
#39308=CARTESIAN_POINT ( 'NONE',  ( 11.02265137815304108, 17.33746510307418731, -28.70764649880413089 ) ) ;
#39309=ORIENTED_EDGE ( 'NONE', *, *, #32917, .T. ) ;
#39310=CARTESIAN_POINT ( 'NONE',  ( 11.03878455726504093, 17.42581041319598611, -28.07733810068037528 ) ) ;
#39313=CARTESIAN_POINT ( 'NONE',  ( -15.13066917251539145, 26.42877163258943796, -8.292150810359242286 ) ) ;
#39315=CARTESIAN_POINT ( 'NONE',  ( -13.73555582509986728, -24.12058157067978570, -13.51135623849643075 ) ) ;
#39319=CARTESIAN_POINT ( 'NONE',  ( -17.86905274512871244, -10.06606982860865607, -30.00000000000002132 ) ) ;
#39320=CARTESIAN_POINT ( 'NONE',  ( -4.698712440877560681, -19.95451542538867784, -30.00000000000000355 ) ) ;
#39322=CARTESIAN_POINT ( 'NONE',  ( 11.69146759026597238, 16.83997637742415776, -30.00000000000000000 ) ) ;
#39324=CARTESIAN_POINT ( 'NONE',  ( 20.53763572180891828, 6.763609892796464074, -22.15629058788150729 ) ) ;
#39331=CARTESIAN_POINT ( 'NONE',  ( -22.44886821189929904, -0.3562293043217420463, -22.60475047268272775 ) ) ;
#39332=CARTESIAN_POINT ( 'NONE',  ( 27.25673043994063960, 0.07488738648532623776, -14.45827337014668679 ) ) ;
#39333=CYLINDRICAL_SURFACE ( 'NONE', #13112, 62.00000000000001421 ) ;
#39343=DIRECTION ( 'NONE',  ( -1.000000000000000000, 0.000000000000000000, 0.000000000000000000 ) ) ;
#39344=CARTESIAN_POINT ( 'NONE',  ( 0.3901599449075797699, 36.15865306409283875, -10.17303319637575676 ) ) ;
#39354=CARTESIAN_POINT ( 'NONE',  ( 9.943094648483580045, 18.21399347630012144, -27.36083611208444566 ) ) ;
#39357=CARTESIAN_POINT ( 'NONE',  ( -17.07654005633402150, 13.06277261991058580, -22.21483479645549153 ) ) ;
#39360=CARTESIAN_POINT ( 'NONE',  ( 15.28437775947960908, -26.40254534672767406, -7.826725057383953299 ) ) ;
#39362=CARTESIAN_POINT ( 'NONE',  ( 11.01243325502136372, 17.44311777400445607, -28.07576541037593287 ) ) ;
#39365=CARTESIAN_POINT ( 'NONE',  ( -29.58504087036580188, -23.16551093242282278, -7.131814702964139663 ) ) ;
#39366=CARTESIAN_POINT ( 'NONE',  ( 2.775580681383440051, -20.45610540486786277, -27.72389806004756352 ) ) ;
#39367=CARTESIAN_POINT ( 'NONE',  ( 14.15536964391180241, 23.64370951135699173, -13.52742165616817438 ) ) ;
#39368=CARTESIAN_POINT ( 'NONE',  ( 21.31969949502798656, 11.87203962839359761, -9.396023366860072557 ) ) ;
#39371=CARTESIAN_POINT ( 'NONE',  ( -4.242919837288198437, 20.95646936440089547, -25.66960880586146843 ) ) ;
#39375=CIRCLE ( 'NONE', #21845, 21.00000000000001776 ) ;
#39381=CARTESIAN_POINT ( 'NONE',  ( -23.87967171433753677, 0.6314381994875827298, -19.51309412989072456 ) ) ;
#39382=CARTESIAN_POINT ( 'NONE',  ( 35.24497909167011045, -11.81349549158436041, -6.720739232717652278 ) ) ;
#39394=CARTESIAN_POINT ( 'NONE',  ( 15.80417486761067813, 13.15001486149802901, -28.27561554616373130 ) ) ;
#39396=CARTESIAN_POINT ( 'NONE',  ( 10.38712762836738790, 29.35899506542313731, -13.09421097062898376 ) ) ;
#39398=CARTESIAN_POINT ( 'NONE',  ( -21.39046744509776232, 10.41410512707694558, -12.88491266128117196 ) ) ;
#39400=DIRECTION ( 'NONE',  ( -1.000000000000000000, 0.000000000000000000, 0.000000000000000000 ) ) ;
#39401=CARTESIAN_POINT ( 'NONE',  ( 14.16828251099090608, -24.17632410410987021, -13.47354249254208192 ) ) ;
#39404=CARTESIAN_POINT ( 'NONE',  ( 23.06249103411542478, 13.31513540672987972, -13.39439507595155199 ) ) ;
#39406=CARTESIAN_POINT ( 'NONE',  ( -11.17299096545415793, 17.76456080679757932, -26.22365104219313992 ) ) ;
#39407=CARTESIAN_POINT ( 'NONE',  ( -13.25611089641869000, -15.90730867704575857, -27.86709263596938158 ) ) ;
#39408=CARTESIAN_POINT ( 'NONE',  ( 10.01790345176820374, -20.67646280627521804, -20.67097678944346484 ) ) ;
#39412=CARTESIAN_POINT ( 'NONE',  ( -12.11690442435413217, 30.76865878555264544, -9.918238614674569575 ) ) ;
#39416=DIRECTION ( 'NONE',  ( -0.000000000000000000, -0.000000000000000000, -1.000000000000000000 ) ) ;
#39418=CARTESIAN_POINT ( 'NONE',  ( 30.83880836401509029, 0.02450782886024078025, -4.999999999999999112 ) ) ;
#39424=CARTESIAN_POINT ( 'NONE',  ( -30.89051437471967887, -0.02824647624105830826, -4.999999999999999112 ) ) ;
#39427=CARTESIAN_POINT ( 'NONE',  ( 20.30048362414427743, -2.857582090605152558, -29.28181927125163853 ) ) ;
#39428=AXIS2_PLACEMENT_3D ( 'NONE', #31088, #3051, #5897 ) ;
#39436=CARTESIAN_POINT ( 'NONE',  ( -32.33143948542088708, 1.358872982498823268, -5.000000000000000888 ) ) ;
#39445=CARTESIAN_POINT ( 'NONE',  ( 6.820427054864983241, 34.96104138684941631, -9.769343582562422412 ) ) ;
#39448=CARTESIAN_POINT ( 'NONE',  ( 18.61788257364777266, -27.16959213022483510, -6.373035692954665876 ) ) ;
#39453=CARTESIAN_POINT ( 'NONE',  ( 11.62397448804718536, 18.97120798431754096, -22.72432224387674538 ) ) ;
#39456=CARTESIAN_POINT ( 'NONE',  ( -15.13210240647062399, 25.19633130894646911, -9.718349095871507970 ) ) ;
#39460=CARTESIAN_POINT ( 'NONE',  ( 15.46782449521607283, 26.59794325776330481, -4.999999999999998224 ) ) ;
#39462=CARTESIAN_POINT ( 'NONE',  ( 30.86005551239754396, -19.56640338714962013, -9.726560286790116194 ) ) ;
#39465=CARTESIAN_POINT ( 'NONE',  ( -13.55369973957343532, 23.86660515378133240, -14.42750371290488154 ) ) ;
#39468=CARTESIAN_POINT ( 'NONE',  ( -16.00326414221997240, -25.30023022726772552, -11.48905281562103653 ) ) ;
#39472=ORIENTED_EDGE ( 'NONE', *, *, #28400, .T. ) ;
#39473=CARTESIAN_POINT ( 'NONE',  ( -35.49576857290053766, -12.23958519446773785, -5.000000000000004441 ) ) ;
#39474=CARTESIAN_POINT ( 'NONE',  ( -13.09227930551162444, -23.59843141973120595, -14.49164938364699751 ) ) ;
#39476=ORIENTED_EDGE ( 'NONE', *, *, #26148, .T. ) ;
#39477=CARTESIAN_POINT ( 'NONE',  ( 25.86870765427833163, 2.101442506354480599, -14.59862430777500464 ) ) ;
#39482=CARTESIAN_POINT ( 'NONE',  ( -20.52994536750384214, 0.7932886217482892910, -28.70470255602677057 ) ) ;
#39484=CARTESIAN_POINT ( 'NONE',  ( 20.54983429119329941, 0.05123126462676740045, -28.67845366199332346 ) ) ;
#39487=CARTESIAN_POINT ( 'NONE',  ( -26.89440075162845289, 4.411995506115219179, -5.952929326054199777 ) ) ;
#39497=CARTESIAN_POINT ( 'NONE',  ( -20.05673146015622521, 4.300176513202893958, -29.99999999999999645 ) ) ;
#39500=CARTESIAN_POINT ( 'NONE',  ( 14.90381431695064585, -14.60044926573648283, -27.07745846674980683 ) ) ;
#39503=CARTESIAN_POINT ( 'NONE',  ( 12.16824354003327535, 20.78390325353091228, -19.44999157952565128 ) ) ;
#39506=CARTESIAN_POINT ( 'NONE',  ( -16.44063469669066535, 22.69260288965874750, -7.852988990058472396 ) ) ;
#39509=CARTESIAN_POINT ( 'NONE',  ( 15.11779573149777178, 26.08460211011391294, -8.768163045224820706 ) ) ;
#39511=CARTESIAN_POINT ( 'NONE',  ( 12.65336495216310553, 21.05333586549351921, -18.45227026116430125 ) ) ;
#39512=VERTEX_POINT ( 'NONE', #3853 ) ;
#39513=CARTESIAN_POINT ( 'NONE',  ( -15.23016191995029445, 26.73636172458780180, -7.352086281858299266 ) ) ;
#39515=CARTESIAN_POINT ( 'NONE',  ( -10.58818753192410966, -19.56084638205915027, -22.72817583048230006 ) ) ;
#39519=CARTESIAN_POINT ( 'NONE',  ( -32.68238800772844144, -18.40062344110566883, -8.403867360342845316 ) ) ;
#39520=CARTESIAN_POINT ( 'NONE',  ( -10.79967333563281429, -24.51318330059240935, -11.70098447834189059 ) ) ;
#39522=CARTESIAN_POINT ( 'NONE',  ( 12.40075146136572215, 17.14821721898418261, -25.15186329211611493 ) ) ;
#39524=CARTESIAN_POINT ( 'NONE',  ( 21.85184851404966366, 6.109037027396825081, -18.92964341907457637 ) ) ;
#39530=CARTESIAN_POINT ( 'NONE',  ( -31.67541566499863137, -1.212671030267491457, -7.318079979765841792 ) ) ;
#39531=CARTESIAN_POINT ( 'NONE',  ( 29.86521059342267037, -0.02516630548550341170, -9.704683626496786175 ) ) ;
#39539=B_SPLINE_CURVE_WITH_KNOTS ( 'NONE', 3,
 ( #2579, #27351, #39739, #18812, #12312, #12508 ),
 .UNSPECIFIED., .F., .F.,
 ( 4, 1, 1, 4 ),
 ( 0.000000000000000000, 0.1250000000429448144, 0.2500000000286252688, 0.3034822677883343145 ),
 .UNSPECIFIED. ) ;
#39543=CARTESIAN_POINT ( 'NONE',  ( 1.576739634193315531, 38.46478598617967748, -5.435507960873805722 ) ) ;
#39552=CARTESIAN_POINT ( 'NONE',  ( 10.64953201439048591, 19.84495155912917852, -22.56251018198367220 ) ) ;
#39555=CARTESIAN_POINT ( 'NONE',  ( -16.01363482889661682, 13.06226528883478721, -27.14623243372550832 ) ) ;
#39559=CARTESIAN_POINT ( 'NONE',  ( 14.97993852148964145, -25.99036409581853846, -9.238322188113263778 ) ) ;
#39562=CARTESIAN_POINT ( 'NONE',  ( 15.16414560994073035, 26.31667483029525556, -8.296495527103925127 ) ) ;
#39564=CARTESIAN_POINT ( 'NONE',  ( 11.10756861982301125, 19.59949212537556562, -20.90349153980999475 ) ) ;
#39566=CARTESIAN_POINT ( 'NONE',  ( -17.31219681121567788, -13.52410775897827477, -24.27504181234872505 ) ) ;
#39567=CARTESIAN_POINT ( 'NONE',  ( 4.011976552904903848, -24.82011946043718353, -6.449216445830162847 ) ) ;
#39568=CARTESIAN_POINT ( 'NONE',  ( 13.43547369680725012, 21.83571133183076540, -16.47867356606642986 ) ) ;
#39569=CARTESIAN_POINT ( 'NONE',  ( 21.54236824818556073, 11.99210819226683711, -7.428645542648590450 ) ) ;
#39572=CARTESIAN_POINT ( 'NONE',  ( -4.142698204329950507, 24.13178648764145606, -20.78291476969486951 ) ) ;
#39582=CARTESIAN_POINT ( 'NONE',  ( -22.69002229967135520, 0.7462262646974573421, -21.63419033603206643 ) ) ;
#39583=CARTESIAN_POINT ( 'NONE',  ( 35.38149650531432400, -10.69973295221460141, -6.299277470973589921 ) ) ;
#39594=CARTESIAN_POINT ( 'NONE',  ( -19.48557158514988785, -11.24999999999987743, 10.00000000000000000 ) ) ;
#39597=ADVANCED_FACE ( 'NONE', ( #34735 ), #15515, .F. ) ;
#39598=CARTESIAN_POINT ( 'NONE',  ( 28.89712736758817613, -22.26113267439890109, -9.299949049805807277 ) ) ;
#39599=CARTESIAN_POINT ( 'NONE',  ( 16.25326542110554939, 12.54616751129404584, -28.85328854345905469 ) ) ;
#39600=CARTESIAN_POINT ( 'NONE',  ( 9.822137042998281942, 25.39517083171130096, -16.97761038151271862 ) ) ;
#39602=CARTESIAN_POINT ( 'NONE',  ( -21.81785358434161637, 11.77199115278586028, -5.000000000000000000 ) ) ;
#39605=CARTESIAN_POINT ( 'NONE',  ( 9.791560039807741589, -18.01123673837627592, -29.34227149249296929 ) ) ;
#39608=CARTESIAN_POINT ( 'NONE',  ( -11.10259761515444765, 17.62853563763367859, -26.82830193443789568 ) ) ;
#39609=CARTESIAN_POINT ( 'NONE',  ( -13.59989706787225572, -15.33919494678365680, -30.00000000000001421 ) ) ;
#39610=CARTESIAN_POINT ( 'NONE',  ( 14.19885085794842894, -26.30396096727126221, -6.890628514556540907 ) ) ;
#39614=CARTESIAN_POINT ( 'NONE',  ( -8.796796072880949779, 22.03530637549132365, -21.13878428389095632 ) ) ;
#39620=CARTESIAN_POINT ( 'NONE',  ( 20.47975215921984216, 0.9111364859620186829, -30.00000000000000000 ) ) ;
#39626=CARTESIAN_POINT ( 'NONE',  ( -25.20729123572924379, 0.3862878095295266823, -17.43940099721178782 ) ) ;
#39629=CARTESIAN_POINT ( 'NONE',  ( 30.71250582953177144, -3.685950063347092076, -12.25764069449938809 ) ) ;
#39639=CARTESIAN_POINT ( 'NONE',  ( 14.23945615837883949, -31.58416516429907972, 3.000000000000000000 ) ) ;
#39642=CARTESIAN_POINT ( 'NONE',  ( 7.734772747480874067, 34.12887688845987810, -10.23333199772818070 ) ) ;
#39648=CARTESIAN_POINT ( 'NONE',  ( 12.38700900889000422, -16.57502586561705016, -27.91489560070839460 ) ) ;
#39649=LINE ( 'NONE', #3476, #6748 ) ;
#39653=CARTESIAN_POINT ( 'NONE',  ( 10.95197819135580630, 17.38279901324217036, -28.70470247791863727 ) ) ;
#39655=CARTESIAN_POINT ( 'NONE',  ( -15.04084753456836410, 25.47187635758209368, -9.713999766003432512 ) ) ;
#39658=CARTESIAN_POINT ( 'NONE',  ( 11.49405981918322439, -20.98321110018536828, -19.50239126088900221 ) ) ;
#39660=CARTESIAN_POINT ( 'NONE',  ( 15.41013925098940440, 26.53795535406381489, -6.417150894498828251 ) ) ;
#39662=CARTESIAN_POINT ( 'NONE',  ( 19.29646234545531769, -12.21333632372317091, -22.98710221298432543 ) ) ;
#39664=CARTESIAN_POINT ( 'NONE',  ( -15.11591168330041235, 27.33994589239279804, -6.872610621541277887 ) ) ;
#39666=CARTESIAN_POINT ( 'NONE',  ( -14.88990478036455833, -23.71550094554306654, -14.34039717371376810 ) ) ;
#39669=CARTESIAN_POINT ( 'NONE',  ( -35.34736855013350976, -11.03791369283689328, -6.297914269266797760 ) ) ;
#39670=CARTESIAN_POINT ( 'NONE',  ( -9.320207966883044648, -18.25898334416423197, -29.35196178604148542 ) ) ;
#39673=CARTESIAN_POINT ( 'NONE',  ( 29.29107452043095350, 1.132527418749026182, -8.309007812652541958 ) ) ;
#39679=CARTESIAN_POINT ( 'NONE',  ( -23.34145163311095672, 0.4855504374881212115, -20.53287417781590918 ) ) ;
#39682=CARTESIAN_POINT ( 'NONE',  ( 30.92579311035478895, -1.297794089189396871, -9.623581977891010553 ) ) ;
#39687=CARTESIAN_POINT ( 'NONE',  ( -24.50095130057663084, 3.514676660001284425, -15.68173609412164282 ) ) ;
#39696=VERTEX_POINT ( 'NONE', #27712 ) ;
#39697=CARTESIAN_POINT ( 'NONE',  ( -21.25477442056000399, 6.622378896756878852, -20.01598680303737154 ) ) ;
#39700=CARTESIAN_POINT ( 'NONE',  ( 21.59233126178605033, -21.18517331184714081, -14.86128476917193630 ) ) ;
#39702=CARTESIAN_POINT ( 'NONE',  ( 11.01155832696060166, 17.88005758764968789, -26.20616980121537409 ) ) ;
#39705=CARTESIAN_POINT ( 'NONE',  ( -13.53617536424694379, 15.84659297203116424, -26.44149828717701567 ) ) ;
#39708=CARTESIAN_POINT ( 'NONE',  ( 15.35276837714096487, 26.56664761675495967, -6.888009055590721630 ) ) ;
#39710=CARTESIAN_POINT ( 'NONE',  ( 12.13489577391687746, 19.91918273965261932, -20.54176214682888357 ) ) ;
#39712=CARTESIAN_POINT ( 'NONE',  ( -12.06785836680760937, 19.99931457666742318, -20.52815288208361011 ) ) ;
#39713=DIRECTION ( 'NONE',  ( -0.000000000000000000, -0.000000000000000000, -1.000000000000000000 ) ) ;
#39715=CARTESIAN_POINT ( 'NONE',  ( -10.54623483126699668, -19.57291301703272879, -22.73368254332207883 ) ) ;
#39717=CARTESIAN_POINT ( 'NONE',  ( -28.72041673430533137, -15.03451237313814204, -13.80826013931377005 ) ) ;
#39718=CARTESIAN_POINT ( 'NONE',  ( -11.41304656535760209, -25.54597899413777640, -7.851881303444170790 ) ) ;
#39720=CARTESIAN_POINT ( 'NONE',  ( 15.83034964957195179, 23.90031239945711761, -8.791623678892117155 ) ) ;
#39722=CARTESIAN_POINT ( 'NONE',  ( 20.06920181270377412, 5.944727635545681288, -25.41012073482777822 ) ) ;
#39728=CARTESIAN_POINT ( 'NONE',  ( -25.76299961875513844, -0.6882523748748244907, -17.30342747421279270 ) ) ;
#39729=CARTESIAN_POINT ( 'NONE',  ( 20.52955548149205001, 0.8017222527024847611, -28.70499869001353588 ) ) ;
#39733=CARTESIAN_POINT ( 'NONE',  ( 35.48557158514988430, -11.24999999999998046, 6.000000000000000000 ) ) ;
#39734=FACE_OUTER_BOUND ( 'NONE', #9126, .T. ) ;
#39739=CARTESIAN_POINT ( 'NONE',  ( 35.84808252048253507, -3.038699442442335030, -4.999999999999999112 ) ) ;
#39740=CARTESIAN_POINT ( 'NONE',  ( 1.474331469296633612, 20.86371088087402370, -26.97373403608622766 ) ) ;
#39748=CARTESIAN_POINT ( 'NONE',  ( 12.66415514388964247, 24.32263371310837030, -15.28493877312508964 ) ) ;
#39752=CARTESIAN_POINT ( 'NONE',  ( -18.28296541247297924, 14.26023631948706694, -15.91594685420020738 ) ) ;
#39753=CARTESIAN_POINT ( 'NONE',  ( -15.41558956984162521, 26.78481017248023832, 0.000000000000000000 ) ) ;
#39755=CARTESIAN_POINT ( 'NONE',  ( 13.71882174050663927, -24.11825156489150856, -13.51284417636739654 ) ) ;
#39756=CARTESIAN_POINT ( 'NONE',  ( -12.15296441974668262, -16.58779298946083358, -28.59925402789991367 ) ) ;
#39757=CARTESIAN_POINT ( 'NONE',  ( 12.65336495216307533, 21.05333586549357960, -18.45227026116427993 ) ) ;
#39758=CARTESIAN_POINT ( 'NONE',  ( 15.16184759445628139, 26.32446738171400824, -8.296192284030361463 ) ) ;
#39762=CARTESIAN_POINT ( 'NONE',  ( -16.46096347412068539, -13.67449536700828716, -25.64341775554081337 ) ) ;
#39764=CARTESIAN_POINT ( 'NONE',  ( -0.2650373451695002269, -20.49916026595607121, -29.42941051173712097 ) ) ;
#39765=CARTESIAN_POINT ( 'NONE',  ( 15.40551039434233083, 25.82709679606264430, -7.831030787721910968 ) ) ;
#39766=CARTESIAN_POINT ( 'NONE',  ( 20.06132735707487669, 11.19275764913479065, -15.94899771753667572 ) ) ;
#39768=CARTESIAN_POINT ( 'NONE',  ( -2.848530395113699321, 20.31062432315956201, -29.99999999999998224 ) ) ;
#39770=CARTESIAN_POINT ( 'NONE',  ( -34.83329005959444657, -6.589775719143758259, -5.000000000000002665 ) ) ;
#39778=CARTESIAN_POINT ( 'NONE',  ( -29.78284714116363574, 0.4461029049765271592, -8.773278634192886116 ) ) ;
#39779=CARTESIAN_POINT ( 'NONE',  ( 24.92085914673013036, -9.179035951187309195, -18.69283157082075775 ) ) ;
#39783=CARTESIAN_POINT ( 'NONE',  ( -35.48557158514985588, -11.25000000000002309, 6.000000000000000000 ) ) ;
#39785=ADVANCED_FACE ( 'NONE', ( #15325 ), #33829, .T. ) ;
#39786=DIRECTION ( 'NONE',  ( 1.000000000000000000, 0.000000000000000000, -0.000000000000000000 ) ) ;
#39792=CARTESIAN_POINT ( 'NONE',  ( -16.00000000000000000, 22.50000000000000355, 0.000000000000000000 ) ) ;
#39794=CARTESIAN_POINT ( 'NONE',  ( 23.74751641108253253, -18.28319883384900990, -15.71451449610176887 ) ) ;
#39795=CARTESIAN_POINT ( 'NONE',  ( 16.64565377271186009, 14.14783685497081933, -21.10538628858365229 ) ) ;
#39796=CARTESIAN_POINT ( 'NONE',  ( 12.20628291170280733, 31.91935747496564701, -8.112038654058029152 ) ) ;
#39797=VERTEX_POINT ( 'NONE', #3332 ) ;
#39798=CARTESIAN_POINT ( 'NONE',  ( -22.03145203603800084, 10.67872040110599485, -9.392672953967160510 ) ) ;
#39802=EDGE_CURVE ( 'NONE', #1089, #30187, #25263, .T. ) ;
#39803=CARTESIAN_POINT ( 'NONE',  ( 13.49272883091155606, -23.63509699019526167, -14.46508437397573843 ) ) ;
#39806=CARTESIAN_POINT ( 'NONE',  ( -15.21760210513949829, 26.45671326379792987, -7.826101484237490524 ) ) ;
#39807=CARTESIAN_POINT ( 'NONE',  ( -17.15649068250308673, -19.26226397553716652, -18.90765395908277569 ) ) ;
#39808=CARTESIAN_POINT ( 'NONE',  ( 8.501931199692817742, -21.76549204576950203, -18.75867965171295282 ) ) ;
#39812=CARTESIAN_POINT ( 'NONE',  ( -6.868207022587211164, 20.65556158837918588, -24.50483338991505633 ) ) ;
#39818=CARTESIAN_POINT ( 'NONE',  ( 25.20856571035977467, 0.3839094494008684078, -17.43916632868277716 ) ) ;
#39822=CARTESIAN_POINT ( 'NONE',  ( -29.33832633994033046, 0.09267334156268687562, -10.65398983853952508 ) ) ;
#39826=CARTESIAN_POINT ( 'NONE',  ( 22.06145134990718404, -2.477892607279924775, -23.48296052362532294 ) ) ;
#39831=CARTESIAN_POINT ( 'NONE',  ( -35.36940577612494963, -20.42053594592269761, -4.999999999999992895 ) ) ;
#39836=CARTESIAN_POINT ( 'NONE',  ( 19.48557158514982746, -11.25000000000009415, 3.000000000000000000 ) ) ;
#39838=CARTESIAN_POINT ( 'NONE',  ( 3.888268390277564102, 20.12764833916413210, -29.23063393235646501 ) ) ;
#39843=EDGE_CURVE ( 'NONE', #33201, #6388, #9436, .T. ) ;
#39844=CARTESIAN_POINT ( 'NONE',  ( 17.57430537192386666, -27.14116438782096097, -5.925949327191978533 ) ) ;
#39845=FILL_AREA_STYLE ('',( #5721 ) ) ;
#39851=CARTESIAN_POINT ( 'NONE',  ( -15.30597197327310433, 26.47602732279704441, -7.358011888683543944 ) ) ;
#39853=CARTESIAN_POINT ( 'NONE',  ( 15.35461928258050612, -26.68267657520923919, -5.946095485900740663 ) ) ;
#39857=CARTESIAN_POINT ( 'NONE',  ( -10.03540317069667509, 17.94769342537721712, -28.66663826095419054 ) ) ;
#39859=CARTESIAN_POINT ( 'NONE',  ( -12.32505676087189350, -18.97741914115109907, -22.50295322248722130 ) ) ;
#39863=CARTESIAN_POINT ( 'NONE',  ( -27.91051972509944434, -10.53651564714228783, -15.73446641547097968 ) ) ;
#39864=CARTESIAN_POINT ( 'NONE',  ( -15.11465166066981247, -26.62188994178503876, -5.946145182990577815 ) ) ;
#39867=CARTESIAN_POINT ( 'NONE',  ( 26.36218513174588551, 2.083777371321898109, -13.61866023419330674 ) ) ;
#39871=CARTESIAN_POINT ( 'NONE',  ( -20.97825103701413951, 0.7222979316363659086, -26.21732548705084298 ) ) ;
#39874=CARTESIAN_POINT ( 'NONE',  ( 24.94893617927477436, -0.4134396669885003206, -18.34106591124777452 ) ) ;
#39877=CARTESIAN_POINT ( 'NONE',  ( -21.25151043518313898, 2.851751769872009401, -24.07782968374341337 ) ) ;
#39888=CARTESIAN_POINT ( 'NONE',  ( -24.07025619749217427, 8.010103448123961911, -7.414577760795920902 ) ) ;
#39891=CARTESIAN_POINT ( 'NONE',  ( 17.28033604266353507, -15.93370173550165347, -21.98823515398838779 ) ) ;
#39895=CARTESIAN_POINT ( 'NONE',  ( 10.77342450413916630, 17.44087877699069367, -29.34380338842519009 ) ) ;
#39898=CARTESIAN_POINT ( 'NONE',  ( -13.30210127107427986, 18.52526325335603730, -20.73340722121258750 ) ) ;
#39901=CARTESIAN_POINT ( 'NONE',  ( 13.50462022322065359, 22.78994049946557965, -15.45234425914835796 ) ) ;
#39905=CARTESIAN_POINT ( 'NONE',  ( -11.04193823641116801, 17.67045093990668292, -26.82258941759701543 ) ) ;
#39907=CARTESIAN_POINT ( 'NONE',  ( -10.06113038743805532, -18.77530449096024512, -25.00346255012576435 ) ) ;
#39910=CARTESIAN_POINT ( 'NONE',  ( -33.58157224492879322, -18.91014262129728962, -4.999999999999998224 ) ) ;
#39911=CARTESIAN_POINT ( 'NONE',  ( -13.80334467884919647, -26.14942442241866516, -7.363983261614664322 ) ) ;
#39913=CARTESIAN_POINT ( 'NONE',  ( 16.08594598475725590, 23.47361198360156820, -8.321775003293000239 ) ) ;
#39915=CARTESIAN_POINT ( 'NONE',  ( 21.78838290119088583, 6.945878216539049355, -17.92683057917631118 ) ) ;
#39921=CARTESIAN_POINT ( 'NONE',  ( -31.63647013363080873, -0.8270238094956995356, -4.999999999999999112 ) ) ;
#39923=CARTESIAN_POINT ( 'NONE',  ( 22.25509359485367256, 0.5259994801797849284, -22.71717593399117874 ) ) ;
#39929=CARTESIAN_POINT ( 'NONE',  ( 21.88444403592372112, 6.126538576424477966, -21.50719306941230613 ) ) ;
#39936=CARTESIAN_POINT ( 'NONE',  ( 0.8308715916267807033, 20.49243450554475743, -30.00000000000001066 ) ) ;
#39941=EDGE_CURVE ( 'NONE', #39797, #20959, #18380, .T. ) ;
#39946=CARTESIAN_POINT ( 'NONE',  ( 14.87731805253066142, 27.78693658398923461, -7.324495699756750078 ) ) ;
#39949=CARTESIAN_POINT ( 'NONE',  ( -16.47736608385881141, 12.45964520604596082, -27.15966153433127062 ) ) ;
#39954=CARTESIAN_POINT ( 'NONE',  ( 10.23053142960224804, -19.16244173123859440, -23.85327837102780180 ) ) ;
#39955=CARTESIAN_POINT ( 'NONE',  ( -12.67448603152304187, -16.20977607892205086, -28.57815234595146237 ) ) ;
#39957=CARTESIAN_POINT ( 'NONE',  ( 13.19408550500376265, 22.26414250881884982, -16.44051050966041316 ) ) ;
#39962=CARTESIAN_POINT ( 'NONE',  ( -24.51042783259964963, -20.45774332969374854, -13.85571432261770042 ) ) ;
#39963=CARTESIAN_POINT ( 'NONE',  ( 1.432041688667228030, -21.91824802019722895, -20.12581347459805414 ) ) ;
#39964=CARTESIAN_POINT ( 'NONE',  ( 14.03171047072867239, 22.83987516452802780, -14.50959830643082604 ) ) ;
#39965=CARTESIAN_POINT ( 'NONE',  ( 17.68185794339073169, 10.78269052861306321, -26.62269099698529473 ) ) ;
#39967=CARTESIAN_POINT ( 'NONE',  ( -5.264215711173335421, 37.05024581972982389, -7.560166499036732546 ) ) ;
#39969=CARTESIAN_POINT ( 'NONE',  ( -22.02142196946409669, -4.043980901898116542, -23.33374139521805901 ) ) ;
#39977=CARTESIAN_POINT ( 'NONE',  ( -20.45512865215935960, 1.365572444264179897, -30.00000000000000000 ) ) ;
#39978=CARTESIAN_POINT ( 'NONE',  ( 19.79492923429188522, -6.644088801164120817, -27.03743231145483961 ) ) ;
#39987=CARTESIAN_POINT ( 'NONE',  ( -4.146361853739318093, 37.19997570623368688, -7.982000101131666803 ) ) ;
#39991=CARTESIAN_POINT ( 'NONE',  ( 24.71324896981895591, -20.25039165369232208, -13.85207717093263646 ) ) ;
#39992=CARTESIAN_POINT ( 'NONE',  ( 16.38953877806516246, 12.68919556586870456, -26.59742149645854781 ) ) ;
#39993=CARTESIAN_POINT ( 'NONE',  ( 12.83069131337032509, 30.87910589201018041, -8.585112319502103517 ) ) ;
#39995=CARTESIAN_POINT ( 'NONE',  ( -20.34773337042144092, 9.024600177409785928, -19.04359522162117102 ) ) ;
#39997=CARTESIAN_POINT ( 'NONE',  ( 15.37979159366119397, -26.42576798054937370, -7.823598831600837578 ) ) ;
#40000=CARTESIAN_POINT ( 'NONE',  ( 22.40982762235196901, 2.618079236896951656, -21.24786896499729139 ) ) ;
#40002=CARTESIAN_POINT ( 'NONE',  ( -11.28807574537728442, 18.05517005563689281, -25.01156050316573243 ) ) ;
#40004=CARTESIAN_POINT ( 'NONE',  ( -13.59989706787225572, -15.33919494678365680, -29.26247283103435493 ) ) ;
#40005=CARTESIAN_POINT ( 'NONE',  ( 10.21648603655621379, -24.71841561882959581, -10.75073561233235253 ) ) ;
#40009=CARTESIAN_POINT ( 'NONE',  ( -6.548765011332742247, 19.65220123129988039, -27.84161395793670124 ) ) ;
#40014=CARTESIAN_POINT ( 'NONE',  ( 20.81540970976022109, 0.8324466887874750753, -26.83074899403284164 ) ) ;
#40015=CARTESIAN_POINT ( 'NONE',  ( 8.301277145684258230, 36.28737808747508353, -5.000000000000000888 ) ) ;
#40016=CARTESIAN_POINT ( 'NONE',  ( 0.000000000000000000, 0.000000000000000000, -30.00000000000000000 ) ) ;
#40018=CARTESIAN_POINT ( 'NONE',  ( -20.48057623381365033, 0.8922431241703845384, -30.00000000000000000 ) ) ;
#40021=CARTESIAN_POINT ( 'NONE',  ( 28.07197903033539532, -5.801645677830485681, -15.91382734764840201 ) ) ;
#40026=CARTESIAN_POINT ( 'NONE',  ( -33.62187204924172335, 0.04418559750806146796, -5.000000000000002665 ) ) ;
#40030=FACE_BOUND ( 'NONE', #5925, .T. ) ;
#40031=VERTEX_POINT ( 'NONE', #16324 ) ;
#40038=CARTESIAN_POINT ( 'NONE',  ( 7.873866743966726922, 34.78796317335525856, -9.337550848925753044 ) ) ;
#40042=CARTESIAN_POINT ( 'NONE',  ( 17.00416740508952174, -26.36028068555279447, -9.146751134521531768 ) ) ;
#40047=CARTESIAN_POINT ( 'NONE',  ( -11.71011565210685035, 18.88845938667280677, -22.73910212722063662 ) ) ;
#40049=CARTESIAN_POINT ( 'NONE',  ( 10.65270019876893137, -20.03412338725443220, -21.63978030402215680 ) ) ;
#40055=CARTESIAN_POINT ( 'NONE',  ( -9.673362312327872914, 18.76285134508493968, -26.06461302575264583 ) ) ;
#40056=CARTESIAN_POINT ( 'NONE',  ( -20.54949627891300779, -27.17849093361366641, -5.904791858424460749 ) ) ;
#40061=CARTESIAN_POINT ( 'NONE',  ( -35.33576435770064705, -9.891194556348709810, -6.303855711779147164 ) ) ;
#40062=CARTESIAN_POINT ( 'NONE',  ( -12.86026711733400774, -23.08413008810780198, -15.46047026364893995 ) ) ;
#40065=CARTESIAN_POINT ( 'NONE',  ( 20.87261353721463664, 1.691488166188070075, -26.30017656618466404 ) ) ;
#40070=CARTESIAN_POINT ( 'NONE',  ( -29.42332256357913067, -0.003158690108220226205, -10.64750720974525500 ) ) ;
#40072=CARTESIAN_POINT ( 'NONE',  ( 28.21183386950785632, -1.421389276423470127, -14.30337687367899235 ) ) ;
#40074=DIRECTION ( 'NONE',  ( -0.000000000000000000, -0.000000000000000000, -1.000000000000000000 ) ) ;
#40078=CARTESIAN_POINT ( 'NONE',  ( -26.22013064122013404, 3.515541298840649809, -11.72090826476172865 ) ) ;
#40080=FACE_OUTER_BOUND ( 'NONE', #8914, .T. ) ;
#40082=CARTESIAN_POINT ( 'NONE',  ( 17.34253826607186255, 27.32041144404028543, 0.000000000000000000 ) ) ;
#40090=CARTESIAN_POINT ( 'NONE',  ( -23.94224112514191205, 7.985727600362816148, -8.389107632434875228 ) ) ;
#40093=CARTESIAN_POINT ( 'NONE',  ( 18.05169300019579026, -18.77641457309465522, -18.83767055183944095 ) ) ;
#40097=CARTESIAN_POINT ( 'NONE',  ( 15.15757690463086149, 26.65769437118299479, -7.819476649599757856 ) ) ;
#40099=CARTESIAN_POINT ( 'NONE',  ( -14.75810761987182929, 21.35594160732316027, -14.59729096891024192 ) ) ;
#40102=CARTESIAN_POINT ( 'NONE',  ( 15.30435262198499480, 26.48161234833224498, -7.357992236420034970 ) ) ;
#40106=CARTESIAN_POINT ( 'NONE',  ( -15.31676148297655615, 27.12555199532522110, -5.472534537103582508 ) ) ;
#40108=CARTESIAN_POINT ( 'NONE',  ( -15.53934119414200410, -26.55776016592740163, -7.352091074212602884 ) ) ;
#40110=CARTESIAN_POINT ( 'NONE',  ( -18.72341571292924201, -9.819713513424439100, -26.25964704346830558 ) ) ;
#40111=CARTESIAN_POINT ( 'NONE',  ( -9.876300105305748644, -20.21249212776923443, -21.72942160044624771 ) ) ;
#40112=CARTESIAN_POINT ( 'NONE',  ( 75.15099915297797395, 43.38844959084117647, -5.000000000000000000 ) ) ;
#40113=CARTESIAN_POINT ( 'NONE',  ( 12.28921816709972248, 16.91395354023228492, -26.33542656321613151 ) ) ;
#40115=CARTESIAN_POINT ( 'NONE',  ( 21.86544796520013634, 5.303751907987186875, -19.93596551504636238 ) ) ;
#40116=DIRECTION ( 'NONE',  ( -0.000000000000000000, -0.000000000000000000, 1.000000000000000000 ) ) ;
#40118=CARTESIAN_POINT ( 'NONE',  ( -20.46001567034013391, -27.07608408263049427, -6.799282311406788182 ) ) ;
#40120=CARTESIAN_POINT ( 'NONE',  ( -31.98245490244095635, -1.244365697959704642, -5.467109644685292480 ) ) ;
#40122=CARTESIAN_POINT ( 'NONE',  ( 30.14155812561973846, -0.1321297161395868502, -9.228335630909516141 ) ) ;
#40129=CARTESIAN_POINT ( 'NONE',  ( 12.05832241004688399, 18.99596958976722760, -30.00000000000000000 ) ) ;
#40131=DIRECTION ( 'NONE',  ( 1.000000000000000000, 0.000000000000000000, 0.000000000000000000 ) ) ;
#40136=CARTESIAN_POINT ( 'NONE',  ( -15.48853125999098701, -26.74269726803709446, -5.000000000000000000 ) ) ;
#40138=CARTESIAN_POINT ( 'NONE',  ( 2.821578699638708887, 27.66899254656360441, -17.62327247309158906 ) ) ;
#40141=CARTESIAN_POINT ( 'NONE',  ( -17.00000000000000000, 22.50000000000000355, 10.00000000000000000 ) ) ;
#40146=CARTESIAN_POINT ( 'NONE',  ( 12.80256909985179092, 22.95103652443984998, -16.35598967180559171 ) ) ;
#40148=CIRCLE ( 'NONE', #27830, 17.00000000000000000 ) ;
#40150=CARTESIAN_POINT ( 'NONE',  ( -15.80284921427163880, 13.98913085816324298, -24.33118825873222590 ) ) ;
#40154=CARTESIAN_POINT ( 'NONE',  ( 15.48852768438595362, -26.74270545139661337, -5.474205978023907626 ) ) ;
#40155=CARTESIAN_POINT ( 'NONE',  ( -12.11431921870781281, -16.53859995802357474, -30.00000000000001066 ) ) ;
#40156=DIRECTION ( 'NONE',  ( 1.000000000000000000, 0.000000000000000000, 0.000000000000000000 ) ) ;
#40157=CARTESIAN_POINT ( 'NONE',  ( 13.20319059294109820, 22.24725340734820023, -16.44263110745769296 ) ) ;
#40161=CARTESIAN_POINT ( 'NONE',  ( -15.05265445420552517, -26.25383179241455878, -8.298612710543265436 ) ) ;
#40164=CARTESIAN_POINT ( 'NONE',  ( -25.25503446062520396, -21.08292511653661805, -12.93509045432853455 ) ) ;
#40165=CARTESIAN_POINT ( 'NONE',  ( 1.643370889305333371, -23.47708040232879867, -13.90816583911588467 ) ) ;
#40166=CARTESIAN_POINT ( 'NONE',  ( 15.32296600055157398, 25.42927303866269284, -8.774763805950231088 ) ) ;
#40167=CARTESIAN_POINT ( 'NONE',  ( 22.72267378955431028, 10.13466626278336769, -6.937383578344491930 ) ) ;
#40169=CARTESIAN_POINT ( 'NONE',  ( -5.311406340589158503, 37.48456040921701771, -6.284425160920512177 ) ) ;
#40171=CARTESIAN_POINT ( 'NONE',  ( -20.37366957899092057, -3.711739399828728470, -27.85939855946655186 ) ) ;
#40174=DIRECTION ( 'NONE',  ( 1.000000000000000000, 0.000000000000000000, -0.000000000000000000 ) ) ;
#40177=CARTESIAN_POINT ( 'NONE',  ( -23.78118149983960095, 0.8666473556403437861, -19.53966836938907292 ) ) ;
#40179=CARTESIAN_POINT ( 'NONE',  ( 34.88728563833267060, -12.83225574243902223, -7.568163508673742434 ) ) ;
#40182=LINE ( 'NONE', #39783, #17422 ) ;
#40184=AXIS2_PLACEMENT_3D ( 'NONE', #4262, #19705, #16663 ) ;
#40187=CARTESIAN_POINT ( 'NONE',  ( 19.48557158514975285, -11.24999999999995737, 10.00000000000000000 ) ) ;
#40189=CARTESIAN_POINT ( 'NONE',  ( -3.201270893313360233, 28.76478025971673702, -16.65328222338712294 ) ) ;
#40193=CARTESIAN_POINT ( 'NONE',  ( 21.15267166395459597, -16.25933725513243289, -18.65893975419588813 ) ) ;
#40195=CARTESIAN_POINT ( 'NONE',  ( 19.41339421492355299, 15.80365212772844430, -7.907966775341815691 ) ) ;
#40196=CARTESIAN_POINT ( 'NONE',  ( 9.218513230433782013, 21.74694333236849175, -21.18942908098420830 ) ) ;
#40198=CARTESIAN_POINT ( 'NONE',  ( -17.70440478334998247, 10.53096322850521460, -27.73763193811898375 ) ) ;
#40199=CARTESIAN_POINT ( 'NONE',  ( 12.19805850000708780, -24.73057336344299628, -11.66080542555461008 ) ) ;
ENDSEC;
END-ISO-10303-21;
